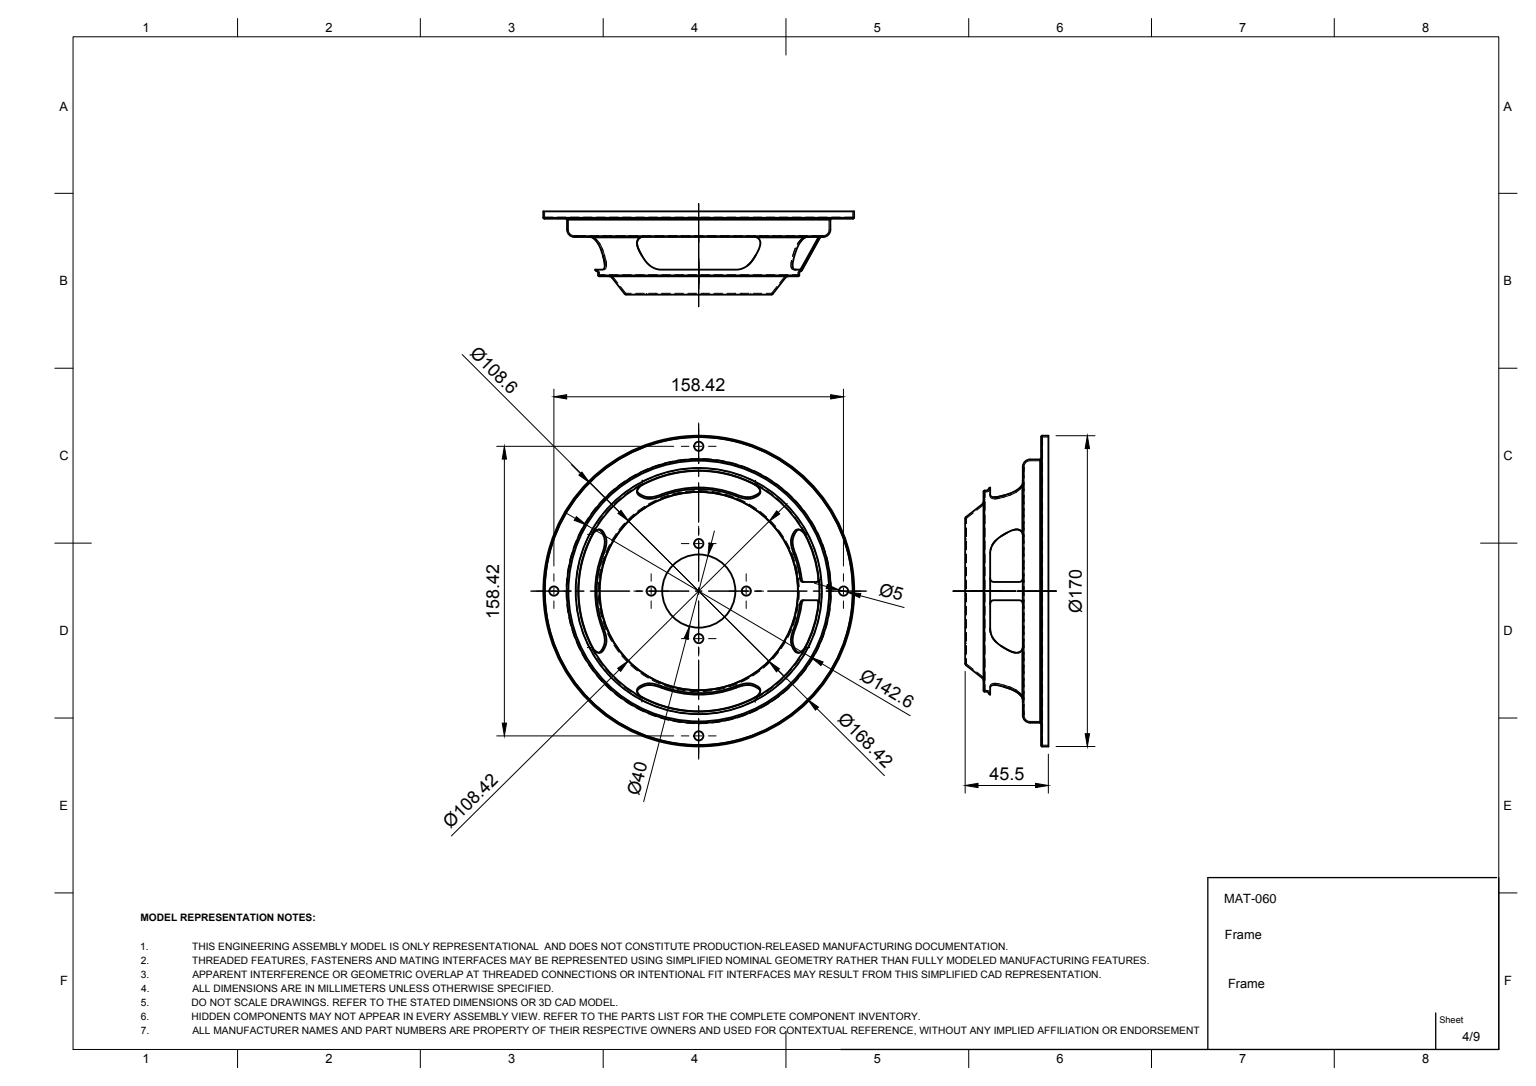
ISO-10303-21;
HEADER;
FILE_DESCRIPTION (('STEP AP214'),
    '1' );
FILE_NAME ('Frame.step',
    '2026-10-29T23:46:56',
    ( '' ),
    ( '' ),
    'SwSTEP 2.0',
    'SolidWorks 2020',
    '' );
FILE_SCHEMA (( 'AUTOMOTIVE_DESIGN' ));
ENDSEC;

DATA;
#1=ADVANCED_FACE ( 'NONE', ( #23407 ), #603, .F. ) ;
#9=CARTESIAN_POINT ( 'NONE',  ( 52.18344119656808289, -5.936379232154279428, 107.4303245894588628 ) ) ;
#10=ORIENTED_EDGE ( 'NONE', *, *, #17862, .T. ) ;
#11=DIRECTION ( 'NONE',  ( 0.000000000000000000, 0.000000000000000000, -1.000000000000000000 ) ) ;
#13=VECTOR ( 'NONE', #9862, 1000.000000000000000 ) ;
#23=DIRECTION ( 'NONE',  ( 0.000000000000000000, 0.000000000000000000, 1.000000000000000000 ) ) ;
#25=CONICAL_SURFACE ( 'NONE', #4214, 67.38776620500242132, 0.5061454830783623793 ) ;
#26=VERTEX_POINT ( 'NONE', #18783 ) ;
#40=CARTESIAN_POINT ( 'NONE',  ( 21.09785597605719332, 12.26495659406217342, 47.04930799450051637 ) ) ;
#48=DIRECTION ( 'NONE',  ( 1.000000000000000000, -3.756723415560144304E-15, 0.000000000000000000 ) ) ;
#62=PLANE ( 'NONE',  #14629 ) ;
#83=CONICAL_SURFACE ( 'NONE', #4821, 67.99999999999998579, 0.5061454830783623793 ) ;
#96=CARTESIAN_POINT ( 'NONE',  ( -35.64882101543633297, 9.925589859889722533, 42.04930799450051637 ) ) ;
#99=EDGE_LOOP ( 'NONE', ( #29307, #17559, #4595, #27909 ) ) ;
#106=DIRECTION ( 'NONE',  ( 0.000000000000000000, 0.000000000000000000, 1.000000000000000000 ) ) ;
#114=CARTESIAN_POINT ( 'NONE',  ( 80.65492537559437380, -5.936611295272316902, 15.94352045161622655 ) ) ;
#138=CIRCLE ( 'NONE', #18459, 2.500000000000003553 ) ;
#147=ORIENTED_EDGE ( 'NONE', *, *, #1574, .F. ) ;
#151=CARTESIAN_POINT ( 'NONE',  ( -9.910881874767294875, -5.936607700120025477, -13.36061728824001804 ) ) ;
#162=PRODUCT_CONTEXT ( 'NONE', #1750, 'mechanical' ) ;
#167=DIRECTION ( 'NONE',  ( -0.000000000000000000, -1.000000000000000000, -0.000000000000000000 ) ) ;
#186=EDGE_CURVE ( 'NONE', #20059, #17152, #210, .T. ) ;
#189=CARTESIAN_POINT ( 'NONE',  ( -29.27613032885505007, 5.786704587343633577, 77.24891569812123748 ) ) ;
#199=CARTESIAN_POINT ( 'NONE',  ( 42.60793425459065986, 11.86918370369814113, 98.63420711611333047 ) ) ;
#203=ORIENTED_EDGE ( 'NONE', *, *, #32319, .T. ) ;
#206=LINE ( 'NONE', #27459, #13028 ) ;
#208=ORIENTED_EDGE ( 'NONE', *, *, #19172, .F. ) ;
#210=CIRCLE ( 'NONE', #18531, 55.85791022362053582 ) ;
#235=CARTESIAN_POINT ( 'NONE',  ( -3.126678918709510313, 11.18855628041951711, -3.738293121569808086 ) ) ;
#239=CARTESIAN_POINT ( 'NONE',  ( 75.35669764717297880, -2.578969365796030200, 80.79736519221168578 ) ) ;
#245=CARTESIAN_POINT ( 'NONE',  ( 75.84373340226019877, -1.823725651226874023, 80.73552270632580985 ) ) ;
#251=DIRECTION ( 'NONE',  ( -0.000000000000000000, 1.000000000000000000, -0.000000000000000000 ) ) ;
#253=VERTEX_POINT ( 'NONE', #29471 ) ;
#259=CIRCLE ( 'NONE', #4453, 2.500000000000002220 ) ;
#274=ORIENTED_EDGE ( 'NONE', *, *, #5995, .T. ) ;
#276=CARTESIAN_POINT ( 'NONE',  ( -5.602943079677954685, 9.702389020015065313, -3.412202488244239884 ) ) ;
#279=CARTESIAN_POINT ( 'NONE',  ( -35.36141981399792655, 11.69881320456492979, 53.11437157513250895 ) ) ;
#288=AXIS2_PLACEMENT_3D ( 'NONE', #28339, #16328, #21250 ) ;
#300=EDGE_CURVE ( 'NONE', #14294, #4546, #9551, .T. ) ;
#302=ORIENTED_EDGE ( 'NONE', *, *, #7357, .T. ) ;
#308=CARTESIAN_POINT ( 'NONE',  ( -10.01358589504979513, -5.935454207834595763, -13.41617548937563598 ) ) ;
#310=ORIENTED_EDGE ( 'NONE', *, *, #2952, .T. ) ;
#313=VERTEX_POINT ( 'NONE', #14149 ) ;
#316=CARTESIAN_POINT ( 'NONE',  ( 54.19940832515395357, -4.668720686625173144, 103.9826627183073668 ) ) ;
#322=LINE ( 'NONE', #29718, #31776 ) ;
#324=CARTESIAN_POINT ( 'NONE',  ( -9.765095477396084078, -5.936631694656546721, 107.5327929641237290 ) ) ;
#336=ORIENTED_EDGE ( 'NONE', *, *, #3292, .T. ) ;
#337=EDGE_CURVE ( 'NONE', #10189, #17291, #29573, .T. ) ;
#343=CARTESIAN_POINT ( 'NONE',  ( 81.50778125879762115, -5.936607700120028142, 16.04057014367610989 ) ) ;
#355=ORIENTED_EDGE ( 'NONE', *, *, #11811, .F. ) ;
#359=CARTESIAN_POINT ( 'NONE',  ( -33.78823724555357444, -3.447124724799344175, 13.40102877645825075 ) ) ;
#370=EDGE_CURVE ( 'NONE', #26491, #3553, #7732, .T. ) ;
#378=DIRECTION ( 'NONE',  ( 1.313185983435984691E-29, -1.000000000000000000, -3.761114140369702165E-15 ) ) ;
#379=EDGE_LOOP ( 'NONE', ( #18763, #24620, #4258, #2283 ) ) ;
#388=CARTESIAN_POINT ( 'NONE',  ( 0.6836613156275053171, 11.92558985988973497, 99.90211174246701376 ) ) ;
#408=CARTESIAN_POINT ( 'NONE',  ( -38.57628410747783221, -4.281489722201563985, 13.63563177263803894 ) ) ;
#418=AXIS2_PLACEMENT_3D ( 'NONE', #18138, #28164, #5678 ) ;
#421=CARTESIAN_POINT ( 'NONE',  ( 49.52052953415556402, 8.310461108307681144, -3.337848843846767721 ) ) ;
#422=CARTESIAN_POINT ( 'NONE',  ( -9.880272688099118739, -5.935454078358227470, 107.6100695915628478 ) ) ;
#426=CARTESIAN_POINT ( 'NONE',  ( -14.15471437217249218, -3.295808585244886402, 97.43646483284780402 ) ) ;
#428=CARTESIAN_POINT ( 'NONE',  ( -34.67891837790644871, -3.387818899234932513, 80.71006381137655694 ) ) ;
#432=CARTESIAN_POINT ( 'NONE',  ( -11.20938414847590003, 2.044662169668923113, 99.18612600487385578 ) ) ;
#439=CARTESIAN_POINT ( 'NONE',  ( 21.09785597605719332, -5.986312001188950127, 47.04930799450051637 ) ) ;
#440=CARTESIAN_POINT ( 'NONE',  ( 21.09785597605719332, -19.93545420775220123, 47.04930799450051637 ) ) ;
#448=AXIS2_PLACEMENT_3D ( 'NONE', #832, #23322, #20846 ) ;
#453=ORIENTED_EDGE ( 'NONE', *, *, #7859, .T. ) ;
#458=AXIS2_PLACEMENT_3D ( 'NONE', #16097, #21670, #13655 ) ;
#461=DIRECTION ( 'NONE',  ( -0.000000000000000000, -1.000000000000000000, -0.000000000000000000 ) ) ;
#462=AXIS2_PLACEMENT_3D ( 'NONE', #31638, #14558, #26541 ) ;
#468=CARTESIAN_POINT ( 'NONE',  ( 52.49730020886497783, -5.900224301042255703, 106.3086101802585404 ) ) ;
#476=CARTESIAN_POINT ( 'NONE',  ( 54.28735269144078757, -4.535950511381776629, 103.8461761130624694 ) ) ;
#487=CARTESIAN_POINT ( 'NONE',  ( 21.09785597605719332, 24.86454579224779948, 73.04930799450052348 ) ) ;
#489=CARTESIAN_POINT ( 'NONE',  ( -31.01957187155556639, 11.71410389684668552, 24.52077559777409732 ) ) ;
#494=VECTOR ( 'NONE', #29690, 1000.000000000000000 ) ;
#499=FACE_OUTER_BOUND ( 'NONE', #20854, .T. ) ;
#501=CARTESIAN_POINT ( 'NONE',  ( -29.27613032885505007, -3.086612947480494196, 80.82450247980625591 ) ) ;
#509=DIRECTION ( 'NONE',  ( 0.000000000000000000, 0.000000000000000000, -1.000000000000000000 ) ) ;
#510=DIRECTION ( 'NONE',  ( 0.000000000000000000, 0.000000000000000000, 1.000000000000000000 ) ) ;
#516=LINE ( 'NONE', #23004, #15630 ) ;
#530=CARTESIAN_POINT ( 'NONE',  ( 21.09785597605719332, 15.56454579224779877, 47.04930799450051637 ) ) ;
#532=CIRCLE ( 'NONE', #18851, 65.75844861871132707 ) ;
#536=CARTESIAN_POINT ( 'NONE',  ( -39.42404159773660410, -5.935581334357459937, 77.97933121608268436 ) ) ;
#539=DIRECTION ( 'NONE',  ( 0.000000000000000000, 9.185193130005556732E-17, 1.000000000000000000 ) ) ;
#541=CIRCLE ( 'NONE', #29390, 39.69941114636694124 ) ;
#546=CARTESIAN_POINT ( 'NONE',  ( 21.09785597605719332, 25.56454579224779877, 73.04930799450052348 ) ) ;
#553=DIRECTION ( 'NONE',  ( 0.000000000000000000, 0.000000000000000000, -1.000000000000000000 ) ) ;
#558=ORIENTED_EDGE ( 'NONE', *, *, #25899, .F. ) ;
#559=CARTESIAN_POINT ( 'NONE',  ( 73.65314367107050941, 0.8961463385898641443, 79.88877559804848261 ) ) ;
#565=ORIENTED_EDGE ( 'NONE', *, *, #7783, .F. ) ;
#567=DIRECTION ( 'NONE',  ( 0.000000000000000000, 0.000000000000000000, 1.000000000000000000 ) ) ;
#588=FACE_OUTER_BOUND ( 'NONE', #2822, .T. ) ;
#592=CARTESIAN_POINT ( 'NONE',  ( -34.60289125444462854, 11.64119122789693961, 41.11328754109207040 ) ) ;
#595=CARTESIAN_POINT ( 'NONE',  ( -14.15471437217249218, -3.295808585244886402, 106.8025418868326284 ) ) ;
#598=CARTESIAN_POINT ( 'NONE',  ( -32.75748891819321074, -0.01103702217111705332, 80.26537595473334363 ) ) ;
#603=CYLINDRICAL_SURFACE ( 'NONE', #6358, 2.500000000000002220 ) ;
#610=FACE_OUTER_BOUND ( 'NONE', #4229, .T. ) ;
#619=ORIENTED_EDGE ( 'NONE', *, *, #25170, .T. ) ;
#621=CARTESIAN_POINT ( 'NONE',  ( -9.326276492376491589, 5.308358430270105899, 99.14268250727589304 ) ) ;
#631=VERTEX_POINT ( 'NONE', #4872 ) ;
#632=EDGE_CURVE ( 'NONE', #253, #29537, #8270, .T. ) ;
#644=CARTESIAN_POINT ( 'NONE',  ( 51.92833871100798149, 4.638969541771024829, 99.33413526210576094 ) ) ;
#649=VERTEX_POINT ( 'NONE', #13679 ) ;
#669=ADVANCED_FACE ( 'NONE', ( #28451, #21524, #18734, #1349, #11366, #13363 ), #3978, .T. ) ;
#674=CARTESIAN_POINT ( 'NONE',  ( 81.53764425905508517, -5.935454354499444918, 15.93786951028389254 ) ) ;
#677=FACE_OUTER_BOUND ( 'NONE', #17845, .T. ) ;
#681=CYLINDRICAL_SURFACE ( 'NONE', #3691, 19.99999999999999645 ) ;
#690=CARTESIAN_POINT ( 'NONE',  ( 51.67081420511490819, 5.053071141216423534, 98.28906612357258155 ) ) ;
#700=CARTESIAN_POINT ( 'NONE',  ( -39.43735134593180902, -5.935500344420906238, 77.98272432681935129 ) ) ;
#715=DIRECTION ( 'NONE',  ( 0.000000000000000000, 0.000000000000000000, -1.000000000000000000 ) ) ;
#716=DIRECTION ( 'NONE',  ( 0.000000000000000000, -1.000000000000000000, 0.000000000000000000 ) ) ;
#719=ORIENTED_EDGE ( 'NONE', *, *, #22379, .T. ) ;
#721=DIRECTION ( 'NONE',  ( 3.761114140369701376E-15, 1.000000000000000000, 0.000000000000000000 ) ) ;
#727=CARTESIAN_POINT ( 'NONE',  ( 21.09785597605720042, -5.935454207752337119, 114.2361189024295527 ) ) ;
#737=FACE_OUTER_BOUND ( 'NONE', #17782, .T. ) ;
#739=CARTESIAN_POINT ( 'NONE',  ( 50.61496291931489111, 6.662067023026866153, -4.700640528948444086 ) ) ;
#746=AXIS2_PLACEMENT_3D ( 'NONE', #5481, #25814, #3329 ) ;
#755=CARTESIAN_POINT ( 'NONE',  ( -35.36966210123092225, 10.42011316249520370, 42.00355930600723298 ) ) ;
#760=CARTESIAN_POINT ( 'NONE',  ( -30.89539544812951277, 5.684769981030545871, 77.22998724337006138 ) ) ;
#779=ORIENTED_EDGE ( 'NONE', *, *, #30659, .T. ) ;
#780=CARTESIAN_POINT ( 'NONE',  ( -12.63151429458831743, -2.181906231262896068, 102.0018054233023577 ) ) ;
#782=EDGE_CURVE ( 'NONE', #6039, #26, #8963, .T. ) ;
#787=ORIENTED_EDGE ( 'NONE', *, *, #4701, .T. ) ;
#794=CARTESIAN_POINT ( 'NONE',  ( 52.07598125554711999, -5.935454207752202116, 106.6682925056943958 ) ) ;
#803=CARTESIAN_POINT ( 'NONE',  ( 41.78490141557333004, 11.92558985988973497, 99.79672416560200077 ) ) ;
#820=EDGE_CURVE ( 'NONE', #7388, #14290, #12583, .T. ) ;
#821=ORIENTED_EDGE ( 'NONE', *, *, #29239, .F. ) ;
#822=AXIS2_PLACEMENT_3D ( 'NONE', #1912, #19630, #21767 ) ;
#825=ORIENTED_EDGE ( 'NONE', *, *, #300, .F. ) ;
#828=CARTESIAN_POINT ( 'NONE',  ( -44.53739698818294102, -4.628387878568079650, 52.16470011384033967 ) ) ;
#832=CARTESIAN_POINT ( 'NONE',  ( 47.09785597605719687, 25.56454579224779877, 47.04930799450042400 ) ) ;
#836=DIRECTION ( 'NONE',  ( 0.000000000000000000, 0.000000000000000000, -1.000000000000000000 ) ) ;
#837=CARTESIAN_POINT ( 'NONE',  ( -38.10732830366966084, -5.882756053366322568, 78.42076464377196032 ) ) ;
#840=DIRECTION ( 'NONE',  ( -0.000000000000000000, 1.000000000000000000, -0.000000000000000000 ) ) ;
#845=ORIENTED_EDGE ( 'NONE', *, *, #14632, .T. ) ;
#849=CARTESIAN_POINT ( 'NONE',  ( 50.74134730670688498, 6.496515553941725862, 97.90908627297329758 ) ) ;
#857=ADVANCED_FACE ( 'NONE', ( #10211 ), #16281, .F. ) ;
#859=CARTESIAN_POINT ( 'NONE',  ( -39.50719276739945229, -5.935457263800389960, 77.87558390080170057 ) ) ;
#870=ORIENTED_EDGE ( 'NONE', *, *, #17750, .F. ) ;
#872=CARTESIAN_POINT ( 'NONE',  ( 47.79865503179234310, 9.702389020015065313, 97.51081847724526597 ) ) ;
#874=CARTESIAN_POINT ( 'NONE',  ( -5.602943079677954685, 9.702389020015065313, 98.41455612196619995 ) ) ;
#880=CARTESIAN_POINT ( 'NONE',  ( 76.87534014094269708, -3.386628651589064898, 80.70757180512225659 ) ) ;
#892=ADVANCED_FACE ( 'NONE', ( #20693 ), #17421, .F. ) ;
#902=CARTESIAN_POINT ( 'NONE',  ( -36.15844848744088580, -5.643691937041874773, 79.05968474335206508 ) ) ;
#916=EDGE_LOOP ( 'NONE', ( #23883, #16207, #15273, #30027 ) ) ;
#919=ORIENTED_EDGE ( 'NONE', *, *, #1291, .F. ) ;
#923=CARTESIAN_POINT ( 'NONE',  ( 21.09785597605719332, -5.935454207752083988, -18.70914062421081425 ) ) ;
#935=CARTESIAN_POINT ( 'NONE',  ( -12.30971848159242121, -4.161241697801305151, 103.4774498197331667 ) ) ;
#946=LINE ( 'NONE', #24559, #9376 ) ;
#957=EDGE_LOOP ( 'NONE', ( #2500, #18429, #8067, #18740 ) ) ;
#960=CARTESIAN_POINT ( 'NONE',  ( 47.79865503179234310, 9.702389020015065313, 98.41455612196619995 ) ) ;
#966=EDGE_LOOP ( 'NONE', ( #8106, #14529, #18674, #26585 ) ) ;
#981=EDGE_LOOP ( 'NONE', ( #5763, #6597, #9287, #17362, #5522 ) ) ;
#999=CARTESIAN_POINT ( 'NONE',  ( 21.09785597605719332, 12.39166260509097484, 47.04930799450051637 ) ) ;
#1007=CARTESIAN_POINT ( 'NONE',  ( -58.11219453028166981, -15.93545420775219945, 49.54930799450023926 ) ) ;
#1009=CARTESIAN_POINT ( 'NONE',  ( -10.63512168728995100, -5.773219817368564044, 105.6277383086626145 ) ) ;
#1018=DIRECTION ( 'NONE',  ( 1.000000000000000000, -3.761114140369701376E-15, 0.000000000000000000 ) ) ;
#1028=DIRECTION ( 'NONE',  ( -0.000000000000000000, 1.000000000000000000, -0.000000000000000000 ) ) ;
#1029=DIRECTION ( 'NONE',  ( 0.000000000000000000, -1.000000000000000000, -1.251509963831984395E-16 ) ) ;
#1038=CARTESIAN_POINT ( 'NONE',  ( -63.90214402394282445, -3.935454207752203892, 40.04930799450051637 ) ) ;
#1050=CARTESIAN_POINT ( 'NONE',  ( 21.09785597605719332, -16.72540370141334520, 131.3493079945005491 ) ) ;
#1056=LINE ( 'NONE', #3025, #19895 ) ;
#1057=FACE_OUTER_BOUND ( 'NONE', #25387, .T. ) ;
#1065=VECTOR ( 'NONE', #30419, 1000.000000000000000 ) ;
#1081=PLANE ( 'NONE',  #5494 ) ;
#1096=DIRECTION ( 'NONE',  ( 0.000000000000000000, -1.000000000000000000, 0.000000000000000000 ) ) ;
#1099=AXIS2_PLACEMENT_3D ( 'NONE', #10139, #25067, #9972 ) ;
#1105=AXIS2_PLACEMENT_3D ( 'NONE', #19154, #12280, #17014 ) ;
#1115=ADVANCED_FACE ( 'NONE', ( #11018 ), #18219, .F. ) ;
#1124=DIRECTION ( 'NONE',  ( 1.177206059073964094E-16, -0.2756373558165849391, 0.9612616959384376880 ) ) ;
#1135=CIRCLE ( 'NONE', #4276, 56.47014401861810029 ) ;
#1141=CARTESIAN_POINT ( 'NONE',  ( -4.902144023942810236, 25.56454579224779877, 47.04930799450078638 ) ) ;
#1147=CARTESIAN_POINT ( 'NONE',  ( -36.31353488181962064, 10.17485700342523458, 42.04930799450051637 ) ) ;
#1152=VERTEX_POINT ( 'NONE', #19517 ) ;
#1175=ADVANCED_FACE ( 'NONE', ( #19187 ), #14452, .F. ) ;
#1176=ORIENTED_EDGE ( 'NONE', *, *, #19284, .F. ) ;
#1178=DIRECTION ( 'NONE',  ( 1.000000000000000000, -0.000000000000000000, -0.000000000000000000 ) ) ;
#1194=DIRECTION ( 'NONE',  ( 0.000000000000000000, 1.000000000000000000, 0.000000000000000000 ) ) ;
#1198=ORIENTED_EDGE ( 'NONE', *, *, #25045, .T. ) ;
#1208=CARTESIAN_POINT ( 'NONE',  ( 53.51600554467332671, -5.395280703882722406, -10.73892745771225599 ) ) ;
#1210=ORIENTED_EDGE ( 'NONE', *, *, #8305, .T. ) ;
#1215=VERTEX_POINT ( 'NONE', #17056 ) ;
#1220=CARTESIAN_POINT ( 'NONE',  ( -33.86637752982123573, -3.544489376609568421, 80.67335282074090230 ) ) ;
#1223=CARTESIAN_POINT ( 'NONE',  ( -34.46767470602752326, 11.80860034638430989, 40.73713547295701431 ) ) ;
#1224=VERTEX_POINT ( 'NONE', #15093 ) ;
#1230=CARTESIAN_POINT ( 'NONE',  ( 21.09785597605719332, -15.93545420775219945, 47.04930799450051637 ) ) ;
#1248=CARTESIAN_POINT ( 'NONE',  ( -10.01616728275229740, -5.935340315990530691, -13.32263710021335612 ) ) ;
#1273=CARTESIAN_POINT ( 'NONE',  ( 0.6836613156275053171, 11.92558985988973497, -5.803495753465989893 ) ) ;
#1285=FACE_OUTER_BOUND ( 'NONE', #3726, .T. ) ;
#1290=LINE ( 'NONE', #23943, #31888 ) ;
#1291=EDGE_CURVE ( 'NONE', #10579, #24958, #20556, .T. ) ;
#1299=EDGE_LOOP ( 'NONE', ( #8915, #25452, #7300, #565, #2321, #17317 ) ) ;
#1305=AXIS2_PLACEMENT_3D ( 'NONE', #9730, #19722, #27116 ) ;
#1309=CARTESIAN_POINT ( 'NONE',  ( -35.14417515838577089, 11.92558985988973674, 40.19270369045111124 ) ) ;
#1340=VERTEX_POINT ( 'NONE', #27894 ) ;
#1341=DIRECTION ( 'NONE',  ( -1.000000000000000000, 0.000000000000000000, 0.000000000000000000 ) ) ;
#1349=FACE_BOUND ( 'NONE', #4250, .T. ) ;
#1354=DIRECTION ( 'NONE',  ( 0.000000000000000000, 0.000000000000000000, 1.000000000000000000 ) ) ;
#1366=DIRECTION ( 'NONE',  ( -1.000000000000000000, -0.000000000000000000, -3.491481338843133355E-15 ) ) ;
#1367=CARTESIAN_POINT ( 'NONE',  ( 21.09785597605719332, -19.93545420775220123, 47.04930799450051637 ) ) ;
#1370=DIRECTION ( 'NONE',  ( -0.000000000000000000, -0.000000000000000000, -1.000000000000000000 ) ) ;
#1372=CARTESIAN_POINT ( 'NONE',  ( 51.66808379569695830, 5.388785998227650254, 106.7232700815558957 ) ) ;
#1430=ORIENTED_EDGE ( 'NONE', *, *, #12094, .F. ) ;
#1431=CARTESIAN_POINT ( 'NONE',  ( -10.77327584252841675, 2.854128177266956445, -4.829733788720330878 ) ) ;
#1464=MANIFOLD_SOLID_BREP ( 'Stock-MAT-060-1', #18928 ) ;
#1469=CARTESIAN_POINT ( 'NONE',  ( 76.12931116418575073, -2.304636120132655286, 13.31869760836049466 ) ) ;
#1509=ADVANCED_FACE ( 'NONE', ( #13448 ), #18665, .F. ) ;
#1524=CARTESIAN_POINT ( 'NONE',  ( -39.54681582271551576, -5.935578394679064118, 77.88069024016000697 ) ) ;
#1527=CARTESIAN_POINT ( 'NONE',  ( -44.16105795751995799, -3.935454207752190126, 42.04930799450051637 ) ) ;
#1535=AXIS2_PLACEMENT_3D ( 'NONE', #14725, #29989, #106 ) ;
#1552=DIRECTION ( 'NONE',  ( -0.000000000000000000, 1.000000000000000000, -0.000000000000000000 ) ) ;
#1562=DIRECTION ( 'NONE',  ( 0.000000000000000000, 0.000000000000000000, -1.000000000000000000 ) ) ;
#1563=CARTESIAN_POINT ( 'NONE',  ( -35.12632216515690686, 11.92558985988973674, 40.04930799450050216 ) ) ;
#1572=ORIENTED_EDGE ( 'NONE', *, *, #13901, .T. ) ;
#1574=EDGE_CURVE ( 'NONE', #5070, #14564, #7015, .T. ) ;
#1578=EDGE_CURVE ( 'NONE', #29191, #20681, #12935, .T. ) ;
#1592=AXIS2_PLACEMENT_3D ( 'NONE', #8643, #21258, #11114 ) ;
#1600=DIRECTION ( 'NONE',  ( 0.000000000000000000, 0.000000000000000000, 1.000000000000000000 ) ) ;
#1603=FACE_OUTER_BOUND ( 'NONE', #20703, .T. ) ;
#1620=FACE_OUTER_BOUND ( 'NONE', #14364, .T. ) ;
#1623=VECTOR ( 'NONE', #1124, 1000.000000000000000 ) ;
#1629=CARTESIAN_POINT ( 'NONE',  ( 21.09785597605719332, 15.63322284159649556, -0.008722863421593840538 ) ) ;
#1632=AXIS2_PLACEMENT_3D ( 'NONE', #17122, #14681, #14197 ) ;
#1636=CARTESIAN_POINT ( 'NONE',  ( 75.71263776093286424, -1.580002914024330574, 13.40786461638758098 ) ) ;
#1652=FACE_BOUND ( 'NONE', #19233, .T. ) ;
#1654=CARTESIAN_POINT ( 'NONE',  ( -9.316012264051970249, 5.323792735596123649, -5.040144599709082129 ) ) ;
#1661=CARTESIAN_POINT ( 'NONE',  ( 21.09785597605719332, -19.93545420775220123, 67.04930799450050927 ) ) ;
#1675=CARTESIAN_POINT ( 'NONE',  ( 54.84591317376816022, -2.578969365796082158, -7.209533676615418329 ) ) ;
#1689=ORIENTED_EDGE ( 'NONE', *, *, #14950, .F. ) ;
#1699=DIRECTION ( 'NONE',  ( -1.000000000000000000, 0.000000000000000000, 2.775557561562888984E-15 ) ) ;
#1701=CARTESIAN_POINT ( 'NONE',  ( 72.51299575579318457, 10.39233698702945929, 21.28292367868997204 ) ) ;
#1708=EDGE_CURVE ( 'NONE', #32242, #3463, #29778, .T. ) ;
#1713=VECTOR ( 'NONE', #6688, 1000.000000000000000 ) ;
#1716=CARTESIAN_POINT ( 'NONE',  ( -29.68171735516254373, 11.15114065686176303, 71.33410141647549096 ) ) ;
#1717=CARTESIAN_POINT ( 'NONE',  ( 81.75997733922811506, -5.936629510748242744, 77.99024554604916659 ) ) ;
#1737=CARTESIAN_POINT ( 'NONE',  ( -44.28695544631908376, -5.935454207752205669, 40.04930799450050216 ) ) ;
#1744=ORIENTED_EDGE ( 'NONE', *, *, #22791, .F. ) ;
#1750=APPLICATION_CONTEXT ( 'automotive_design' ) ;
#1755=VECTOR ( 'NONE', #11846, 1000.000000000000000 ) ;
#1763=CARTESIAN_POINT ( 'NONE',  ( -12.56410411622038303, -3.374355247260697244, -7.781004297996404695 ) ) ;
#1791=ADVANCED_FACE ( 'NONE', ( #17996 ), #8000, .F. ) ;
#1794=CARTESIAN_POINT ( 'NONE',  ( 21.09785597605719332, 15.06454579224778456, 102.0493079945005093 ) ) ;
#1800=CARTESIAN_POINT ( 'NONE',  ( 78.44397203118849404, -5.043292969097946887, 14.24782339319855318 ) ) ;
#1808=CARTESIAN_POINT ( 'NONE',  ( 21.09785597605719332, -15.93545420775219945, 126.2593585008393831 ) ) ;
#1809=CARTESIAN_POINT ( 'NONE',  ( -45.58211410561983001, -5.881662548112003286, 40.51623134221831890 ) ) ;
#1818=ORIENTED_EDGE ( 'NONE', *, *, #5124, .F. ) ;
#1819=CARTESIAN_POINT ( 'NONE',  ( -11.94109704398765537, 0.4256545730735167288, -6.630874157835914495 ) ) ;
#1822=DIRECTION ( 'NONE',  ( 0.000000000000000000, 0.000000000000000000, -1.000000000000000000 ) ) ;
#1827=AXIS2_PLACEMENT_3D ( 'NONE', #13329, #10539, #25781 ) ;
#1841=CARTESIAN_POINT ( 'NONE',  ( 21.09785597605720397, -15.43545420775221366, -24.95069200549946586 ) ) ;
#1857=CARTESIAN_POINT ( 'NONE',  ( -39.56017130034231144, -5.935730392421668888, 77.88797225724067630 ) ) ;
#1859=CARTESIAN_POINT ( 'NONE',  ( 80.71684048725118998, -5.935454207752202116, 16.07118271501079221 ) ) ;
#1864=CARTESIAN_POINT ( 'NONE',  ( 21.09785597605719332, 25.56454579224779877, 70.54930799450050927 ) ) ;
#1869=ORIENTED_EDGE ( 'NONE', *, *, #28980, .T. ) ;
#1873=ORIENTED_EDGE ( 'NONE', *, *, #18457, .T. ) ;
#1878=VERTEX_POINT ( 'NONE', #8638 ) ;
#1893=ADVANCED_FACE ( 'NONE', ( #9279 ), #83, .T. ) ;
#1894=VERTEX_POINT ( 'NONE', #21900 ) ;
#1907=AXIS2_PLACEMENT_3D ( 'NONE', #28226, #27904, #5419 ) ;
#1912=CARTESIAN_POINT ( 'NONE',  ( 21.09785597605719332, 25.56454579224779877, 47.04930799450051637 ) ) ;
#1918=CARTESIAN_POINT ( 'NONE',  ( -11.49897738644833645, -5.264348929021194223, -9.633576251181647621 ) ) ;
#1920=CARTESIAN_POINT ( 'NONE',  ( 81.79971628361815306, -5.937448199248381187, 77.92687966219790496 ) ) ;
#1922=AXIS2_PLACEMENT_3D ( 'NONE', #20265, #2460, #29877 ) ;
#1924=CARTESIAN_POINT ( 'NONE',  ( 21.09785597605719332, -8.535454207752287914, 47.04930799450051637 ) ) ;
#1931=CARTESIAN_POINT ( 'NONE',  ( 21.09785597605719332, -5.935454207752083988, 47.04930799449963530 ) ) ;
#1934=CARTESIAN_POINT ( 'NONE',  ( 41.51205063648687599, 11.92558985988973497, -37.95069200549950494 ) ) ;
#1938=CARTESIAN_POINT ( 'NONE',  ( -29.27337757263006424, 2.267350949466874432, 14.79705809024468088 ) ) ;
#1946=EDGE_LOOP ( 'NONE', ( #12322, #14844, #6465, #22478 ) ) ;
#1957=CARTESIAN_POINT ( 'NONE',  ( 75.25323102592015800, -0.6709275202869922072, 13.62290469009603022 ) ) ;
#1976=CARTESIAN_POINT ( 'NONE',  ( -6.242780362964605700, 9.162376348828958683, -4.318210402824582239 ) ) ;
#1986=ORIENTED_EDGE ( 'NONE', *, *, #27426, .F. ) ;
#1991=EDGE_CURVE ( 'NONE', #17686, #12130, #16391, .T. ) ;
#1999=CARTESIAN_POINT ( 'NONE',  ( 53.71827270862435455, -5.211355130743560160, -9.585364147679955593 ) ) ;
#2013=VECTOR ( 'NONE', #10033, 1000.000000000000000 ) ;
#2014=CARTESIAN_POINT ( 'NONE',  ( 52.81327818505165794, -5.811083640285383822, 104.5757368101217679 ) ) ;
#2015=ORIENTED_EDGE ( 'NONE', *, *, #27426, .T. ) ;
#2028=CARTESIAN_POINT ( 'NONE',  ( 72.31638179958355295, 11.69718155787697356, 24.43823011782819776 ) ) ;
#2039=CARTESIAN_POINT ( 'NONE',  ( -30.66701073789274901, 11.92468888572869723, 68.04721722412880069 ) ) ;
#2040=CARTESIAN_POINT ( 'NONE',  ( -29.27613032885505007, -5.935454207752198563, 77.87546120947918382 ) ) ;
#2043=CARTESIAN_POINT ( 'NONE',  ( 51.92400919103563695, -5.935454207752202116, -13.39445452378610568 ) ) ;
#2046=DIRECTION ( 'NONE',  ( -0.000000000000000000, -1.000000000000000000, -0.000000000000000000 ) ) ;
#2047=CARTESIAN_POINT ( 'NONE',  ( 71.61810346057937693, 10.40257568944042710, 72.79952121014760280 ) ) ;
#2073=CARTESIAN_POINT ( 'NONE',  ( 21.09785597605719332, 16.86454579224779948, 47.04930799450051637 ) ) ;
#2083=CARTESIAN_POINT ( 'NONE',  ( 21.09785597605719332, -6.314304012688826795, -18.91914050022838012 ) ) ;
#2085=CARTESIAN_POINT ( 'NONE',  ( -12.50119137592388441, -1.331120222581884560, -6.486951009445048655 ) ) ;
#2086=VERTEX_POINT ( 'NONE', #727 ) ;
#2104=CARTESIAN_POINT ( 'NONE',  ( -29.27337757263006424, 11.92558985988973497, 26.63511333407100778 ) ) ;
#2105=ORIENTED_EDGE ( 'NONE', *, *, #26289, .F. ) ;
#2109=ORIENTED_EDGE ( 'NONE', *, *, #21254, .T. ) ;
#2113=EDGE_CURVE ( 'NONE', #11449, #13013, #22617, .T. ) ;
#2127=DIRECTION ( 'NONE',  ( 0.000000000000000000, 3.754529891495955404E-16, -1.000000000000000000 ) ) ;
#2128=EDGE_LOOP ( 'NONE', ( #25205, #31539, #7322, #24885 ) ) ;
#2130=B_SPLINE_CURVE_WITH_KNOTS ( 'NONE', 3,
 ( #29565, #16909, #16580, #14301, #31697, #16739, #9209, #27088, #28917, #26765, #26929, #11503, #4284, #13979, #31855, #24302, #19200, #21499, #21673, #11838, #1819, #29396, #4445, #9370, #24627, #19533, #1654, #19366, #14467, #19039, #14623, #2147, #24461, #1976, #14138, #16425 ),
 .UNSPECIFIED., .F., .F.,
 ( 4, 2, 2, 2, 2, 2, 2, 2, 2, 2, 2, 2, 2, 2, 2, 2, 2, 4 ),
 ( 2.602085213965210642E-18, 0.001253900128824282905, 0.001880850193236422189, 0.002507800257648561473, 0.003134750322060700974, 0.003761700386472840475, 0.005015600515297116008, 0.005642550579709253340, 0.006269500644121390673, 0.007523400772945662736, 0.008777300901769934799, 0.01003120103059420773, 0.01253900128824275012, 0.01504680154589129598, 0.01630070167471556544, 0.01755460180353983837, 0.01880850193236410783, 0.02006240206118838076 ),
 .UNSPECIFIED. ) ;
#2147=CARTESIAN_POINT ( 'NONE',  ( -7.125208762201825863, 8.281585831149227417, -4.396110345893636584 ) ) ;
#2151=ORIENTED_EDGE ( 'NONE', *, *, #17153, .F. ) ;
#2152=CARTESIAN_POINT ( 'NONE',  ( 21.09785597605719332, 25.56454579224779877, 73.04930799450052348 ) ) ;
#2165=VERTEX_POINT ( 'NONE', #13372 ) ;
#2166=CIRCLE ( 'NONE', #8471, 54.49999999999997868 ) ;
#2169=CARTESIAN_POINT ( 'NONE',  ( 49.11022725746682482, 8.508769500014663478, -3.454732803723541412 ) ) ;
#2177=FACE_BOUND ( 'NONE', #7800, .T. ) ;
#2183=CARTESIAN_POINT ( 'NONE',  ( -30.20912666432285576, 4.777658832336100225, 16.29113105709203779 ) ) ;
#2187=FACE_OUTER_BOUND ( 'NONE', #30023, .T. ) ;
#2195=CARTESIAN_POINT ( 'NONE',  ( -9.880269303432738681, -5.935454207752202116, -12.62465409255485582 ) ) ;
#2196=CARTESIAN_POINT ( 'NONE',  ( -39.45773241730296377, -5.935454212835550969, 77.98461610899785512 ) ) ;
#2197=AXIS2_PLACEMENT_3D ( 'NONE', #3174, #13217, #12896 ) ;
#2201=ORIENTED_EDGE ( 'NONE', *, *, #8975, .T. ) ;
#2207=CARTESIAN_POINT ( 'NONE',  ( -30.66127778995677033, 3.242016564995574335, 78.70398512147052372 ) ) ;
#2223=DIRECTION ( 'NONE',  ( 0.000000000000000000, 0.000000000000000000, -1.000000000000000000 ) ) ;
#2240=ORIENTED_EDGE ( 'NONE', *, *, #13865, .T. ) ;
#2243=AXIS2_PLACEMENT_3D ( 'NONE', #9490, #16213, #21781 ) ;
#2251=CARTESIAN_POINT ( 'NONE',  ( -8.054007235165986600, 7.161243906346020260, 97.76730497187020319 ) ) ;
#2253=CARTESIAN_POINT ( 'NONE',  ( -30.29083761341767911, 10.19527012171080393, 20.98910367824052159 ) ) ;
#2256=CARTESIAN_POINT ( 'NONE',  ( 81.79971628361815306, -5.937394935145312580, 77.97850100859398026 ) ) ;
#2259=CARTESIAN_POINT ( 'NONE',  ( 52.07598125554711999, -5.935454207752202116, 107.5832303370038403 ) ) ;
#2268=CARTESIAN_POINT ( 'NONE',  ( 106.0978559760574313, 1.925589859889728972, 67.46350265493050813 ) ) ;
#2273=CARTESIAN_POINT ( 'NONE',  ( -29.27337757263006424, -3.086620340690746644, 13.27411520529475020 ) ) ;
#2280=AXIS2_PLACEMENT_3D ( 'NONE', #12246, #32269, #2712 ) ;
#2282=AXIS2_PLACEMENT_3D ( 'NONE', #8168, #15877, #13267 ) ;
#2283=ORIENTED_EDGE ( 'NONE', *, *, #5714, .F. ) ;
#2301=SHAPE_DEFINITION_REPRESENTATION ( #8290, #3604 ) ;
#2306=EDGE_CURVE ( 'NONE', #17291, #14793, #22637, .T. ) ;
#2313=CARTESIAN_POINT ( 'NONE',  ( 52.07598125554711999, -5.935454207752203004, 107.5573216553427187 ) ) ;
#2321=ORIENTED_EDGE ( 'NONE', *, *, #21254, .F. ) ;
#2324=CARTESIAN_POINT ( 'NONE',  ( 73.19394920542428906, 11.69997306056223607, 69.64732492378499273 ) ) ;
#2334=DIRECTION ( 'NONE',  ( -0.000000000000000000, 1.000000000000000000, -0.000000000000000000 ) ) ;
#2344=FACE_OUTER_BOUND ( 'NONE', #18141, .T. ) ;
#2370=B_SPLINE_CURVE_WITH_KNOTS ( 'NONE', 3,
 ( #26492, #9256, #1701, #11084, #6306, #13541, #14023, #16794, #16311, #21071, #11722, #18604 ),
 .UNSPECIFIED., .F., .F.,
 ( 4, 2, 2, 2, 2, 4 ),
 ( 0.0003422370341462280100, 0.002080102550335780759, 0.003817968066525333128, 0.005555833582714885498, 0.006424766340809661899, 0.007293699098904438301 ),
 .UNSPECIFIED. ) ;
#2381=ORIENTED_EDGE ( 'NONE', *, *, #26036, .T. ) ;
#2385=CARTESIAN_POINT ( 'NONE',  ( 72.66453678218256584, 3.903925281081655818, 78.31450457581732394 ) ) ;
#2388=DIRECTION ( 'NONE',  ( -0.000000000000000000, -1.000000000000000000, -0.000000000000000000 ) ) ;
#2426=CARTESIAN_POINT ( 'NONE',  ( -35.12632216515691397, 11.92558985988973674, 54.04930799450053769 ) ) ;
#2434=CARTESIAN_POINT ( 'NONE',  ( -44.16105795751995799, -3.935454207752183020, 52.04930799450050927 ) ) ;
#2435=ORIENTED_EDGE ( 'NONE', *, *, #10167, .T. ) ;
#2448=FACE_OUTER_BOUND ( 'NONE', #29487, .T. ) ;
#2449=EDGE_CURVE ( 'NONE', #28013, #10438, #11704, .T. ) ;
#2460=DIRECTION ( 'NONE',  ( -0.000000000000000000, -1.000000000000000000, -0.000000000000000000 ) ) ;
#2467=VERTEX_POINT ( 'NONE', #8521 ) ;
#2494=DIRECTION ( 'NONE',  ( 1.313185983435984691E-29, -1.000000000000000000, -3.761114140369702165E-15 ) ) ;
#2496=B_SPLINE_SURFACE_WITH_KNOTS ( 'NONE', 3, 1, ( 
 ( #29765, #9584 ),
 ( #21872, #27467 ),
 ( #9252, #19905 ),
 ( #19413, #31899 ) ),
 .UNSPECIFIED., .F., .F., .F.,
 ( 4, 4 ),
 ( 2, 2 ),
 ( 0.9958781556774846111, 1.000000000000000000 ),
 ( 0.000000000000000000, 1.000000000000000000 ),
 .UNSPECIFIED. ) ;
#2500=ORIENTED_EDGE ( 'NONE', *, *, #9156, .F. ) ;
#2508=CARTESIAN_POINT ( 'NONE',  ( 41.51205063648687599, 11.92558985988973497, -4.944603100128015960 ) ) ;
#2509=ORIENTED_EDGE ( 'NONE', *, *, #10196, .T. ) ;
#2514=DIRECTION ( 'NONE',  ( -0.000000000000000000, -1.000000000000000000, -0.000000000000000000 ) ) ;
#2519=ORIENTED_EDGE ( 'NONE', *, *, #32257, .F. ) ;
#2526=CARTESIAN_POINT ( 'NONE',  ( -9.883074696779189594, -5.935345006353231589, 107.4930705127871846 ) ) ;
#2530=ORIENTED_EDGE ( 'NONE', *, *, #20490, .F. ) ;
#2538=CARTESIAN_POINT ( 'NONE',  ( 71.64025509781936307, 8.185031362399408650, 75.36104810003064358 ) ) ;
#2541=DIRECTION ( 'NONE',  ( 0.000000000000000000, -0.2756373558169902815, -0.9612616959383214477 ) ) ;
#2543=CARTESIAN_POINT ( 'NONE',  ( 21.09785597605719332, 17.56454579224779877, 47.04930799450051637 ) ) ;
#2545=DIRECTION ( 'NONE',  ( 0.000000000000000000, 0.000000000000000000, -1.000000000000000000 ) ) ;
#2547=EDGE_LOOP ( 'NONE', ( #24954, #30069, #15985, #23180 ) ) ;
#2548=LINE ( 'NONE', #29481, #18243 ) ;
#2550=ORIENTED_EDGE ( 'NONE', *, *, #23423, .T. ) ;
#2553=EDGE_CURVE ( 'NONE', #1215, #16982, #10146, .T. ) ;
#2561=FACE_OUTER_BOUND ( 'NONE', #28539, .T. ) ;
#2563=ORIENTED_EDGE ( 'NONE', *, *, #21276, .T. ) ;
#2565=CARTESIAN_POINT ( 'NONE',  ( 73.61977373202824992, 0.9814505390143158925, 14.24566699581558638 ) ) ;
#2566=CARTESIAN_POINT ( 'NONE',  ( 42.05610609765635388, 11.92558985988972964, -5.593356398450009870 ) ) ;
#2569=CARTESIAN_POINT ( 'NONE',  ( 21.09785597605719332, 14.56957104541719694, -7.455717258668906666 ) ) ;
#2571=CARTESIAN_POINT ( 'NONE',  ( -12.59080382683723442, -1.820484904611798349, 100.8496278133052897 ) ) ;
#2579=CIRCLE ( 'NONE', #8852, 67.36417311134211161 ) ;
#2581=FACE_OUTER_BOUND ( 'NONE', #27056, .T. ) ;
#2591=EDGE_CURVE ( 'NONE', #27103, #29537, #16694, .T. ) ;
#2593=LINE ( 'NONE', #30336, #17952 ) ;
#2614=VERTEX_POINT ( 'NONE', #4241 ) ;
#2617=ORIENTED_EDGE ( 'NONE', *, *, #25045, .F. ) ;
#2619=CARTESIAN_POINT ( 'NONE',  ( 21.09785597605719332, 15.56454579224779877, -7.450692005499464088 ) ) ;
#2631=EDGE_CURVE ( 'NONE', #3463, #27012, #9072, .T. ) ;
#2635=ORIENTED_EDGE ( 'NONE', *, *, #31498, .F. ) ;
#2650=AXIS2_PLACEMENT_3D ( 'NONE', #6932, #27605, #24486 ) ;
#2662=CARTESIAN_POINT ( 'NONE',  ( 41.51205063648687599, 11.92558985988973497, 99.04321908912902472 ) ) ;
#2667=ORIENTED_EDGE ( 'NONE', *, *, #32219, .F. ) ;
#2671=DIRECTION ( 'NONE',  ( 0.000000000000000000, -1.000000000000000000, 0.000000000000000000 ) ) ;
#2672=CARTESIAN_POINT ( 'NONE',  ( 54.82737574693081939, -2.284241381456145970, 101.1271600646791029 ) ) ;
#2685=B_SPLINE_CURVE_WITH_KNOTS ( 'NONE', 3,
 ( #29665, #11936, #4547, #4713, #21932, #14733, #2251, #14563, #12271, #5374, #25228, #27525, #8157, #14894, #432, #12600, #30316, #15532, #5203, #10457, #2571, #5046, #15054, #22419, #20129, #2739, #15377, #30486, #18147, #13086, #12435, #32454, #15213, #9966, #29995, #7830 ),
 .UNSPECIFIED., .F., .F.,
 ( 4, 2, 2, 2, 2, 2, 2, 2, 2, 2, 2, 2, 2, 2, 2, 2, 2, 4 ),
 ( 0.000000000000000000, 0.001327013081135473057, 0.002654026162270946114, 0.003981039243406417003, 0.005308052324541888758, 0.006635065405677360514, 0.007962078486812830536, 0.01061610464908377231, 0.01194311773021923886, 0.01327013081135470368, 0.01459714389249017023, 0.01592415697362563679, 0.01725117005476110160, 0.01857818313589656642, 0.01924168967646430056, 0.01990519621703203124, 0.02056870275759976191, 0.02123220929816749258 ),
 .UNSPECIFIED. ) ;
#2686=ORIENTED_EDGE ( 'NONE', *, *, #28464, .F. ) ;
#2689=CARTESIAN_POINT ( 'NONE',  ( 21.09785597605719332, 14.77459629858661572, 101.3493079945005206 ) ) ;
#2703=CARTESIAN_POINT ( 'NONE',  ( 71.55760889374487022, 9.126991894476596201, 74.42996348956144459 ) ) ;
#2708=FACE_OUTER_BOUND ( 'NONE', #13436, .T. ) ;
#2709=ORIENTED_EDGE ( 'NONE', *, *, #12911, .F. ) ;
#2712=DIRECTION ( 'NONE',  ( 0.000000000000000000, 0.000000000000000000, 1.000000000000000000 ) ) ;
#2713=ORIENTED_EDGE ( 'NONE', *, *, #4530, .T. ) ;
#2715=CARTESIAN_POINT ( 'NONE',  ( 21.09785597605719332, -19.93545420775220123, 47.04930799450051637 ) ) ;
#2726=VERTEX_POINT ( 'NONE', #25241 ) ;
#2733=CARTESIAN_POINT ( 'NONE',  ( 43.69587290534151691, 11.69997306056223607, -5.046785234866655756 ) ) ;
#2734=CARTESIAN_POINT ( 'NONE',  ( -5.602943079677954685, 9.702389020015065313, 98.41455612196619995 ) ) ;
#2735=CARTESIAN_POINT ( 'NONE',  ( -30.56895382951262619, 7.047361869319173522, 76.28100816727524602 ) ) ;
#2739=CARTESIAN_POINT ( 'NONE',  ( -12.07837398813756913, -4.576799740321095378, 102.9520008778022913 ) ) ;
#2744=EDGE_LOOP ( 'NONE', ( #13844, #8496 ) ) ;
#2747=CARTESIAN_POINT ( 'NONE',  ( 81.71508932399986236, -5.936918531481694572, 15.99626209184008552 ) ) ;
#2755=CYLINDRICAL_SURFACE ( 'NONE', #17209, 2.500000000000002220 ) ;
#2783=CARTESIAN_POINT ( 'NONE',  ( 54.63702927177264002, -3.812314126620138577, 103.1735800200605553 ) ) ;
#2790=DIRECTION ( 'NONE',  ( -1.000000000000000000, 0.000000000000000000, -1.110223024625155594E-14 ) ) ;
#2800=AXIS2_PLACEMENT_3D ( 'NONE', #1931, #21944, #9653 ) ;
#2806=EDGE_CURVE ( 'NONE', #1340, #8773, #10695, .T. ) ;
#2812=CARTESIAN_POINT ( 'NONE',  ( 52.12585496443453081, -5.943281723642242831, -10.93395394839392587 ) ) ;
#2815=DIRECTION ( 'NONE',  ( 0.000000000000000000, 0.000000000000000000, -1.000000000000000000 ) ) ;
#2822=EDGE_LOOP ( 'NONE', ( #10818, #13643, #14022, #11285 ) ) ;
#2823=ORIENTED_EDGE ( 'NONE', *, *, #22749, .T. ) ;
#2825=CARTESIAN_POINT ( 'NONE',  ( -31.67509402814005881, 0.3087484226586330038, 13.94399873050154781 ) ) ;
#2826=CARTESIAN_POINT ( 'NONE',  ( 53.37090610332811025, 2.112486173643655096, 99.16308969199836554 ) ) ;
#2830=VERTEX_POINT ( 'NONE', #4894 ) ;
#2837=CIRCLE ( 'NONE', #31726, 1.700000000000000178 ) ;
#2846=EDGE_CURVE ( 'NONE', #11299, #8773, #3328, .T. ) ;
#2855=CARTESIAN_POINT ( 'NONE',  ( -0.4058007941739975033, 11.88152873911358753, 99.49782616222140064 ) ) ;
#2871=CARTESIAN_POINT ( 'NONE',  ( -10.30158825675060008, -5.900224301042254815, -12.20999419125749696 ) ) ;
#2872=CARTESIAN_POINT ( 'NONE',  ( -45.72330504332163059, -5.935454207752205669, 40.04930799450050216 ) ) ;
#2873=CARTESIAN_POINT ( 'NONE',  ( -38.57628410747783221, -5.935454207752202116, 16.07118271501078866 ) ) ;
#2880=VECTOR ( 'NONE', #12997, 1000.000000000000000 ) ;
#2882=B_SPLINE_CURVE_WITH_KNOTS ( 'NONE', 3,
 ( #12590, #422, #15365, #9514, #20119, #23068, #25534, #8147, #30150, #7818, #20275, #20441 ),
 .UNSPECIFIED., .F., .F.,
 ( 4, 2, 2, 2, 2, 4 ),
 ( 0.0003195369756189209219, 0.0003994212195236353908, 0.0004793054634283499139, 0.0005192475853807071483, 0.0005591897073330643828, 0.0006390739512378048725 ),
 .UNSPECIFIED. ) ;
#2886=CARTESIAN_POINT ( 'NONE',  ( 21.09785597605719332, -9.935454207752199451, 118.3493079945004922 ) ) ;
#2892=CARTESIAN_POINT ( 'NONE',  ( -44.02786950842664027, -5.204346380200058242, 52.49783445483662803 ) ) ;
#2898=VERTEX_POINT ( 'NONE', #8649 ) ;
#2903=CARTESIAN_POINT ( 'NONE',  ( -35.22851096958370221, 11.86391768464652152, 53.48664131055646465 ) ) ;
#2934=ORIENTED_EDGE ( 'NONE', *, *, #7599, .T. ) ;
#2937=CARTESIAN_POINT ( 'NONE',  ( 54.80744232836631369, -3.171899563477265094, 102.6569140501756152 ) ) ;
#2945=CARTESIAN_POINT ( 'NONE',  ( 21.09785597605720397, -15.93545420775219945, 131.5493079945005377 ) ) ;
#2952=EDGE_CURVE ( 'NONE', #16490, #29214, #12461, .T. ) ;
#2960=ORIENTED_EDGE ( 'NONE', *, *, #12826, .T. ) ;
#2961=CARTESIAN_POINT ( 'NONE',  ( -29.27613032885505007, 11.92558985988973497, 67.46350265493038023 ) ) ;
#2972=CARTESIAN_POINT ( 'NONE',  ( 43.70893385272968601, 11.69718155787697356, 98.26783381802677297 ) ) ;
#2979=DIRECTION ( 'NONE',  ( 0.000000000000000000, 0.000000000000000000, -1.000000000000000000 ) ) ;
#2991=CARTESIAN_POINT ( 'NONE',  ( -39.48645896158937774, -5.935494601668936276, 77.87709717717420688 ) ) ;
#2999=ORIENTED_EDGE ( 'NONE', *, *, #19749, .F. ) ;
#3010=CARTESIAN_POINT ( 'NONE',  ( 76.42527971025482714, -3.977894809549873401, 80.53958960090274388 ) ) ;
#3016=CARTESIAN_POINT ( 'NONE',  ( 76.50383461303660226, -2.878806504921911813, 80.77738562869335226 ) ) ;
#3022=EDGE_LOOP ( 'NONE', ( #4299, #29590, #26515, #5708 ) ) ;
#3025=CARTESIAN_POINT ( 'NONE',  ( 51.92400919103565116, -5.935454207752198563, -37.95069200549950494 ) ) ;
#3026=ADVANCED_FACE ( 'NONE', ( #17143 ), #18019, .F. ) ;
#3027=CARTESIAN_POINT ( 'NONE',  ( 53.25347890682692054, -5.581242224118425632, -11.00365297242568374 ) ) ;
#3030=ORIENTED_EDGE ( 'NONE', *, *, #14643, .T. ) ;
#3035=AXIS2_PLACEMENT_3D ( 'NONE', #2073, #9793, #12757 ) ;
#3043=ORIENTED_EDGE ( 'NONE', *, *, #3175, .F. ) ;
#3076=CIRCLE ( 'NONE', #462, 2.500000000000003553 ) ;
#3078=VERTEX_POINT ( 'NONE', #10430 ) ;
#3086=ORIENTED_EDGE ( 'NONE', *, *, #29203, .F. ) ;
#3092=CIRCLE ( 'NONE', #25726, 66.44011198581388555 ) ;
#3100=ORIENTED_EDGE ( 'NONE', *, *, #20202, .T. ) ;
#3108=EDGE_CURVE ( 'NONE', #17233, #18486, #24710, .T. ) ;
#3120=CARTESIAN_POINT ( 'NONE',  ( -29.27613032885505007, 2.267353962593735339, 79.30155859000750240 ) ) ;
#3124=CIRCLE ( 'NONE', #28819, 4.000000000000000000 ) ;
#3126=DIRECTION ( 'NONE',  ( -0.000000000000000000, 1.000000000000000000, -0.000000000000000000 ) ) ;
#3137=CARTESIAN_POINT ( 'NONE',  ( 21.09785597605719332, -16.63545420775219696, 123.7593585008393831 ) ) ;
#3145=CONICAL_SURFACE ( 'NONE', #21477, 67.36417311134205477, 1.291543646476234874 ) ;
#3149=CARTESIAN_POINT ( 'NONE',  ( -34.55638539710868429, 11.69883593934741128, 53.11441734066968934 ) ) ;
#3154=CARTESIAN_POINT ( 'NONE',  ( 51.92400919103563695, -5.935454207752202116, -13.56214536183033381 ) ) ;
#3162=CIRCLE ( 'NONE', #17846, 55.87116166729571631 ) ;
#3174=CARTESIAN_POINT ( 'NONE',  ( 21.09785597605719332, -9.935454207752199451, 47.04930799450051637 ) ) ;
#3175=EDGE_CURVE ( 'NONE', #2467, #21280, #30595, .T. ) ;
#3177=CARTESIAN_POINT ( 'NONE',  ( 21.09785597605719332, 24.56454579224780232, 47.04930799450051637 ) ) ;
#3185=CARTESIAN_POINT ( 'NONE',  ( -63.90214402394282445, -5.935454207752202116, 16.07118271501078510 ) ) ;
#3188=CARTESIAN_POINT ( 'NONE',  ( 51.52198844449087289, 5.308358430270121886, -5.044066518274861188 ) ) ;
#3191=AXIS2_PLACEMENT_3D ( 'NONE', #30328, #27374, #7354 ) ;
#3195=EDGE_CURVE ( 'NONE', #7566, #32110, #18003, .T. ) ;
#3198=B_SPLINE_CURVE_WITH_KNOTS ( 'NONE', 3,
 ( #28375, #13595, #25577, #13444, #468, #28048, #3568, #26053, #28208, #794 ),
 .UNSPECIFIED., .F., .F.,
 ( 4, 2, 2, 2, 4 ),
 ( 0.000000000000000000, 0.0008384749106984661516, 0.001257712366047681338, 0.001467331093722273319, 0.001676949821396865299 ),
 .UNSPECIFIED. ) ;
#3209=CARTESIAN_POINT ( 'NONE',  ( -9.728297238921257417, -5.935454207752202116, 106.8025418868326284 ) ) ;
#3210=AXIS2_PLACEMENT_3D ( 'NONE', #25361, #32104, #7646 ) ;
#3212=CARTESIAN_POINT ( 'NONE',  ( -35.20928760015869585, -4.023206877552709670, 80.51010491862120944 ) ) ;
#3218=VERTEX_POINT ( 'NONE', #12743 ) ;
#3224=CARTESIAN_POINT ( 'NONE',  ( -36.31236502847541914, 10.17695955431967114, 52.04930799450051637 ) ) ;
#3232=ORIENTED_EDGE ( 'NONE', *, *, #2113, .F. ) ;
#3239=CARTESIAN_POINT ( 'NONE',  ( -7.669325564611453316, 7.651854857429011503, 98.59257673948808076 ) ) ;
#3240=UNCERTAINTY_MEASURE_WITH_UNIT (LENGTH_MEASURE( 1.000000000000000082E-05 ), #27118, 'distance_accuracy_value', 'NONE');
#3258=( LENGTH_UNIT ( ) NAMED_UNIT ( * ) SI_UNIT ( .MILLI., .METRE. ) );
#3265=TOROIDAL_SURFACE ( 'NONE', #8018, 39.69941114636694834, 1.000000000000000000 ) ;
#3275=CARTESIAN_POINT ( 'NONE',  ( 21.09785597605719687, 25.56454579224779877, 87.23645172943334103 ) ) ;
#3281=ORIENTED_EDGE ( 'NONE', *, *, #3887, .F. ) ;
#3289=CARTESIAN_POINT ( 'NONE',  ( 81.48020857097124292, -5.936921830459689353, 16.01322791396358625 ) ) ;
#3292=EDGE_CURVE ( 'NONE', #7831, #23399, #14353, .T. ) ;
#3301=CYLINDRICAL_SURFACE ( 'NONE', #7374, 2.500000000000002220 ) ;
#3303=CARTESIAN_POINT ( 'NONE',  ( 21.09785597605719332, -16.93042895458276575, 47.04930799450051637 ) ) ;
#3309=ORIENTED_EDGE ( 'NONE', *, *, #32473, .F. ) ;
#3310=CIRCLE ( 'NONE', #21643, 2.500000000000002220 ) ;
#3311=DIRECTION ( 'NONE',  ( 0.000000000000000000, -9.185193130005556732E-17, 1.000000000000000000 ) ) ;
#3317=CARTESIAN_POINT ( 'NONE',  ( -39.40475928260197946, -5.936129750639523195, 77.92715501466686590 ) ) ;
#3318=ORIENTED_EDGE ( 'NONE', *, *, #17652, .F. ) ;
#3319=CIRCLE ( 'NONE', #14866, 65.75844861871132707 ) ;
#3325=CIRCLE ( 'NONE', #4907, 71.29999999999996874 ) ;
#3328=CIRCLE ( 'NONE', #2282, 2.000000000000001776 ) ;
#3329=DIRECTION ( 'NONE',  ( 0.000000000000000000, 0.000000000000000000, 1.000000000000000000 ) ) ;
#3330=PLANE ( 'NONE',  #15126 ) ;
#3335=DIRECTION ( 'NONE',  ( 0.000000000000000000, 0.000000000000000000, 1.000000000000000000 ) ) ;
#3336=EDGE_CURVE ( 'NONE', #26270, #6305, #23780, .T. ) ;
#3338=CARTESIAN_POINT ( 'NONE',  ( -2.054138246187894534, 11.56016961077985350, 98.98610059691263530 ) ) ;
#3340=( NAMED_UNIT ( * ) PLANE_ANGLE_UNIT ( ) SI_UNIT ( $, .RADIAN. ) );
#3344=B_SPLINE_CURVE_WITH_KNOTS ( 'NONE', 3,
 ( #1737, #18641, #31775, #11595, #21417, #28665, #21752, #18794, #6179, #24223, #21266, #23738, #31297, #9288 ),
 .UNSPECIFIED., .F., .F.,
 ( 4, 2, 2, 2, 2, 2, 4 ),
 ( 0.0002010756753325377709, 0.001030312595864772912, 0.001444931056130880969, 0.001859549516396989026, 0.002274167976663097300, 0.002688786436929205791, 0.003518023357461414966 ),
 .UNSPECIFIED. ) ;
#3347=DIRECTION ( 'NONE',  ( 0.000000000000000000, 0.000000000000000000, 1.000000000000000000 ) ) ;
#3356=CARTESIAN_POINT ( 'NONE',  ( 49.32263122391440646, 8.279996179725067407, -4.396176344842519512 ) ) ;
#3373=CARTESIAN_POINT ( 'NONE',  ( -31.01722238679535337, 5.224609680351743002, 77.52734172137031976 ) ) ;
#3383=CARTESIAN_POINT ( 'NONE',  ( -35.57732732147984223, 11.39140128989992817, 52.68243506491521799 ) ) ;
#3394=EDGE_CURVE ( 'NONE', #15480, #14564, #3325, .T. ) ;
#3396=CARTESIAN_POINT ( 'NONE',  ( -12.59179267514473821, -3.218976025668840002, 102.6991991216207936 ) ) ;
#3406=ORIENTED_EDGE ( 'NONE', *, *, #820, .F. ) ;
#3407=CARTESIAN_POINT ( 'NONE',  ( 71.49893360114317886, -3.295808585244882849, 11.79002343214940041 ) ) ;
#3409=VERTEX_POINT ( 'NONE', #1527 ) ;
#3424=CARTESIAN_POINT ( 'NONE',  ( 49.32092071431622315, 8.281585831149220311, 98.49472633489467910 ) ) ;
#3425=FACE_OUTER_BOUND ( 'NONE', #1946, .T. ) ;
#3441=COLOUR_RGB ( '',0.7921568627450980005, 0.8196078431372548767, 0.9333333333333333481 ) ;
#3446=CARTESIAN_POINT ( 'NONE',  ( -44.97602486328538163, -5.513888518307795472, 52.81728120461330889 ) ) ;
#3449=ORIENTED_EDGE ( 'NONE', *, *, #27458, .F. ) ;
#3451=CARTESIAN_POINT ( 'NONE',  ( 81.47887257101615432, -5.936379232154268770, 15.96372277398939588 ) ) ;
#3463=VERTEX_POINT ( 'NONE', #1859 ) ;
#3465=AXIS2_PLACEMENT_3D ( 'NONE', #24622, #14945, #2790 ) ;
#3468=CARTESIAN_POINT ( 'NONE',  ( 21.09785597605720042, -9.935454207752199451, 115.0493079945004951 ) ) ;
#3480=CARTESIAN_POINT ( 'NONE',  ( 52.07077173907278933, -5.935668157269684109, -13.53804821299738492 ) ) ;
#3482=CARTESIAN_POINT ( 'NONE',  ( 21.09785597605719332, -15.93545420775219945, 47.04930799450051637 ) ) ;
#3486=DIRECTION ( 'NONE',  ( 0.000000000000000000, 1.000000000000000000, 0.000000000000000000 ) ) ;
#3488=ORIENTED_EDGE ( 'NONE', *, *, #4254, .F. ) ;
#3493=CARTESIAN_POINT ( 'NONE',  ( -5.145516081992131951, 10.07216359114295479, 98.42132851406103100 ) ) ;
#3515=VERTEX_POINT ( 'NONE', #16463 ) ;
#3517=EDGE_CURVE ( 'NONE', #31078, #18206, #13625, .T. ) ;
#3520=EDGE_CURVE ( 'NONE', #2165, #20059, #21994, .T. ) ;
#3522=AXIS2_PLACEMENT_3D ( 'NONE', #9220, #1341, #11357 ) ;
#3550=DIRECTION ( 'NONE',  ( -0.000000000000000000, -1.000000000000000000, -0.000000000000000000 ) ) ;
#3552=CARTESIAN_POINT ( 'NONE',  ( -9.970446611220443955, -5.937394852768786535, -13.32263710021335612 ) ) ;
#3553=VERTEX_POINT ( 'NONE', #22523 ) ;
#3555=CARTESIAN_POINT ( 'NONE',  ( -6.244038915535443657, 9.161285963347376438, 98.41684214693681554 ) ) ;
#3564=FACE_OUTER_BOUND ( 'NONE', #24438, .T. ) ;
#3568=CARTESIAN_POINT ( 'NONE',  ( 52.31247960063809899, -5.928581419070744651, 106.5177822622708703 ) ) ;
#3571=ORIENTED_EDGE ( 'NONE', *, *, #22749, .F. ) ;
#3587=DIRECTION ( 'NONE',  ( -0.000000000000000000, -1.000000000000000000, -0.000000000000000000 ) ) ;
#3588=CARTESIAN_POINT ( 'NONE',  ( -34.34161333937292682, -4.095223881812850131, 13.61950888151727312 ) ) ;
#3604=SHAPE_REPRESENTATION ( 'Frame', ( #8172 ), #19670 ) ;
#3620=DIRECTION ( 'NONE',  ( 0.000000000000000000, 0.000000000000000000, -1.000000000000000000 ) ) ;
#3624=VERTEX_POINT ( 'NONE', #9744 ) ;
#3632=CARTESIAN_POINT ( 'NONE',  ( -10.74933306299440083, -5.721341737285946749, 105.3592130793008721 ) ) ;
#3640=DIRECTION ( 'NONE',  ( -3.761114140369701376E-15, -1.000000000000000000, 0.000000000000000000 ) ) ;
#3641=CIRCLE ( 'NONE', #32489, 2.500000000000002220 ) ;
#3642=ORIENTED_EDGE ( 'NONE', *, *, #31100, .T. ) ;
#3647=ORIENTED_EDGE ( 'NONE', *, *, #21276, .F. ) ;
#3649=CARTESIAN_POINT ( 'NONE',  ( 21.09785597605719332, 24.86454579224779948, 73.04930799450052348 ) ) ;
#3651=CARTESIAN_POINT ( 'NONE',  ( 71.60181765360115946, 8.510833471476306755, 19.03915849818731232 ) ) ;
#3654=AXIS2_PLACEMENT_3D ( 'NONE', #24340, #4001, #31900 ) ;
#3656=CARTESIAN_POINT ( 'NONE',  ( 21.09785597605719332, 11.92558985988973497, 47.04930799450051637 ) ) ;
#3658=CYLINDRICAL_SURFACE ( 'NONE', #9530, 10.00000000000000178 ) ;
#3666=EDGE_CURVE ( 'NONE', #17152, #7388, #17536, .T. ) ;
#3689=CARTESIAN_POINT ( 'NONE',  ( -36.06597331586808508, -5.586840335632118126, 79.16021068330404376 ) ) ;
#3691=AXIS2_PLACEMENT_3D ( 'NONE', #5934, #840, #25627 ) ;
#3692=ORIENTED_EDGE ( 'NONE', *, *, #5002, .F. ) ;
#3697=LINE ( 'NONE', #13724, #29945 ) ;
#3709=EDGE_CURVE ( 'NONE', #5045, #14332, #24600, .T. ) ;
#3720=CARTESIAN_POINT ( 'NONE',  ( 47.09785597605719687, 25.56454579224779877, 44.54930799450042400 ) ) ;
#3721=CIRCLE ( 'NONE', #8458, 0.2999999999999999334 ) ;
#3724=ORIENTED_EDGE ( 'NONE', *, *, #23274, .F. ) ;
#3726=EDGE_LOOP ( 'NONE', ( #27510, #3449 ) ) ;
#3737=VERTEX_POINT ( 'NONE', #28433 ) ;
#3740=VECTOR ( 'NONE', #4058, 1000.000000000000000 ) ;
#3748=CARTESIAN_POINT ( 'NONE',  ( -3.661041915257567947, 10.95084857405595713, -4.515295244921526674 ) ) ;
#3775=CARTESIAN_POINT ( 'NONE',  ( 74.92883917873734845, 0.05876815387845962801, 13.86745137419974050 ) ) ;
#3778=ORIENTED_EDGE ( 'NONE', *, *, #5714, .T. ) ;
#3797=DIRECTION ( 'NONE',  ( -0.000000000000000000, 1.000000000000000000, -0.000000000000000000 ) ) ;
#3812=AXIS2_PLACEMENT_3D ( 'NONE', #26913, #19184, #28897 ) ;
#3819=VECTOR ( 'NONE', #6668, 1000.000000000000114 ) ;
#3821=DIRECTION ( 'NONE',  ( -0.000000000000000000, -0.000000000000000000, -1.000000000000000000 ) ) ;
#3824=VERTEX_POINT ( 'NONE', #7070 ) ;
#3845=B_SPLINE_CURVE_WITH_KNOTS ( 'NONE', 3,
 ( #10261, #30274, #22876, #23032, #30118, #17626, #18109, #27642 ),
 .UNSPECIFIED., .F., .F.,
 ( 4, 2, 2, 4 ),
 ( 4.856180139528653963E-16, 0.0004427811193179412167, 0.0008855622386353968192, 0.001771124477270308133 ),
 .UNSPECIFIED. ) ;
#3854=CARTESIAN_POINT ( 'NONE',  ( -36.69065127708124407, -5.900665263871069932, 78.38950784583703069 ) ) ;
#3860=AXIS2_PLACEMENT_3D ( 'NONE', #25966, #13511, #18572 ) ;
#3871=DIRECTION ( 'NONE',  ( 0.000000000000000000, 0.000000000000000000, 1.000000000000000000 ) ) ;
#3878=ORIENTED_EDGE ( 'NONE', *, *, #18336, .F. ) ;
#3886=AXIS2_PLACEMENT_3D ( 'NONE', #17092, #9880, #4626 ) ;
#3887=EDGE_CURVE ( 'NONE', #13889, #32220, #14468, .T. ) ;
#3891=CARTESIAN_POINT ( 'NONE',  ( 21.09785597605720042, 16.86454579224779948, 95.68336035963606889 ) ) ;
#3900=CARTESIAN_POINT ( 'NONE',  ( -12.13387836560771582, -4.491775094913932342, -8.765527212216683850 ) ) ;
#3908=AXIS2_PLACEMENT_3D ( 'NONE', #22141, #29549, #21655 ) ;
#3911=AXIS2_PLACEMENT_3D ( 'NONE', #5524, #10130, #25056 ) ;
#3927=B_SPLINE_CURVE_WITH_KNOTS ( 'NONE', 3,
 ( #26709, #31650, #16531, #11621 ),
 .UNSPECIFIED., .F., .F.,
 ( 4, 4 ),
 ( 0.07242793514135081878, 0.08828840816840291539 ),
 .UNSPECIFIED. ) ;
#3928=EDGE_CURVE ( 'NONE', #10149, #6712, #14396, .T. ) ;
#3944=DIRECTION ( 'NONE',  ( -0.000000000000000000, -1.000000000000000000, -0.000000000000000000 ) ) ;
#3945=CARTESIAN_POINT ( 'NONE',  ( 77.48905355674300210, -4.114116020023757869, 13.63154984733677644 ) ) ;
#3978=PLANE ( 'NONE',  #24103 ) ;
#3993=CARTESIAN_POINT ( 'NONE',  ( -39.57297000773472462, -5.936060209327997939, 77.91230730958153572 ) ) ;
#4001=DIRECTION ( 'NONE',  ( 0.000000000000000000, -1.000000000000000000, 0.000000000000000000 ) ) ;
#4010=CONICAL_SURFACE ( 'NONE', #1922, 55.00000000000000000, 0.7853981633974552734 ) ;
#4011=CARTESIAN_POINT ( 'NONE',  ( 21.09785597605719332, 24.86454579224779948, 21.04930799450051282 ) ) ;
#4014=ORIENTED_EDGE ( 'NONE', *, *, #20879, .T. ) ;
#4029=DIRECTION ( 'NONE',  ( 0.000000000000000000, 0.000000000000000000, 1.000000000000000000 ) ) ;
#4032=DIRECTION ( 'NONE',  ( 0.000000000000000000, 0.000000000000000000, -1.000000000000000000 ) ) ;
#4035=CARTESIAN_POINT ( 'NONE',  ( -30.89605511857140741, 11.92558985988973497, 26.63511333407100423 ) ) ;
#4040=ADVANCED_FACE ( 'NONE', ( #23762 ), #16258, .T. ) ;
#4058=DIRECTION ( 'NONE',  ( 0.000000000000000000, -0.7071067811865426878, -0.7071067811865524577 ) ) ;
#4065=CARTESIAN_POINT ( 'NONE',  ( 106.0978559760576019, 9.702389020015065313, 20.34850893876566857 ) ) ;
#4067=CARTESIAN_POINT ( 'NONE',  ( -63.90214402394282445, -3.935454207752200340, 54.04930799450051637 ) ) ;
#4073=DIRECTION ( 'NONE',  ( 1.177206059073821606E-16, -0.2756373558169902815, 0.9612616959383214477 ) ) ;
#4076=LINE ( 'NONE', #16873, #9868 ) ;
#4081=CIRCLE ( 'NONE', #25568, 2.500000000000002220 ) ;
#4090=AXIS2_PLACEMENT_3D ( 'NONE', #29104, #1194, #5979 ) ;
#4093=CARTESIAN_POINT ( 'NONE',  ( 78.85204100697130514, -5.379633064793138963, 14.58826358935728607 ) ) ;
#4096=ORIENTED_EDGE ( 'NONE', *, *, #5611, .F. ) ;
#4098=FACE_BOUND ( 'NONE', #31253, .T. ) ;
#4107=EDGE_CURVE ( 'NONE', #28880, #11449, #6056, .T. ) ;
#4108=CARTESIAN_POINT ( 'NONE',  ( -10.50890583686613233, -5.822320178462002893, 105.8904890469746221 ) ) ;
#4112=PLANE ( 'NONE',  #5628 ) ;
#4120=AXIS2_PLACEMENT_3D ( 'NONE', #11962, #17647, #12578 ) ;
#4124=CIRCLE ( 'NONE', #7798, 3.299999999999997158 ) ;
#4130=EDGE_LOOP ( 'NONE', ( #2015, #19239 ) ) ;
#4132=CARTESIAN_POINT ( 'NONE',  ( 21.09785597605719332, 13.06454579224779877, 47.04930799450051637 ) ) ;
#4138=DIRECTION ( 'NONE',  ( -0.000000000000000000, -1.000000000000000000, -0.000000000000000000 ) ) ;
#4146=CARTESIAN_POINT ( 'NONE',  ( 21.09785597605719332, 25.13358275951983956, 47.04930799450051637 ) ) ;
#4151=CARTESIAN_POINT ( 'NONE',  ( -39.57027300287975180, -5.936134875209708284, 77.92680640967554950 ) ) ;
#4152=AXIS2_PLACEMENT_3D ( 'NONE', #17893, #13142, #15111 ) ;
#4153=DIRECTION ( 'NONE',  ( -0.000000000000000000, -0.000000000000000000, -1.000000000000000000 ) ) ;
#4163=ORIENTED_EDGE ( 'NONE', *, *, #23422, .T. ) ;
#4164=AXIS2_PLACEMENT_3D ( 'NONE', #16848, #26699, #24072 ) ;
#4167=FACE_OUTER_BOUND ( 'NONE', #5039, .T. ) ;
#4177=ADVANCED_FACE ( 'NONE', ( #19973 ), #17836, .T. ) ;
#4194=LINE ( 'NONE', #21257, #9997 ) ;
#4206=PLANE ( 'NONE',  #22692 ) ;
#4214=AXIS2_PLACEMENT_3D ( 'NONE', #27448, #4963, #19885 ) ;
#4224=DIRECTION ( 'NONE',  ( -0.000000000000000000, -1.000000000000000000, -0.000000000000000000 ) ) ;
#4229=EDGE_LOOP ( 'NONE', ( #3086, #2109, #18719, #13884, #1873, #12457, #27366, #9754, #1869, #10125, #28331, #6387, #19755, #31230, #16179, #22211 ) ) ;
#4234=DIRECTION ( 'NONE',  ( -0.000000000000000000, -1.000000000000000000, -0.000000000000000000 ) ) ;
#4241=CARTESIAN_POINT ( 'NONE',  ( 21.09785597605720042, 13.74476430820393347, -7.250692005499486115 ) ) ;
#4250=EDGE_LOOP ( 'NONE', ( #6915, #11061 ) ) ;
#4254=EDGE_CURVE ( 'NONE', #2898, #12194, #9698, .T. ) ;
#4256=CONICAL_SURFACE ( 'NONE', #10035, 54.74424859897010975, 1.291543646475813212 ) ;
#4258=ORIENTED_EDGE ( 'NONE', *, *, #16249, .T. ) ;
#4260=CARTESIAN_POINT ( 'NONE',  ( -9.728297238921268075, -5.935454207752198563, 132.0493079945005377 ) ) ;
#4262=EDGE_CURVE ( 'NONE', #14332, #21437, #12425, .T. ) ;
#4272=CARTESIAN_POINT ( 'NONE',  ( 47.79865503179234310, 9.702389020015065313, 98.41455612196619995 ) ) ;
#4276=AXIS2_PLACEMENT_3D ( 'NONE', #40, #27452, #29589 ) ;
#4282=CARTESIAN_POINT ( 'NONE',  ( -10.18637189516808661, -5.903366343041435371, 106.3819261045487536 ) ) ;
#4284=CARTESIAN_POINT ( 'NONE',  ( -12.64433984712379022, -2.833757427854236788, -8.318886203631619125 ) ) ;
#4287=FACE_OUTER_BOUND ( 'NONE', #14635, .T. ) ;
#4299=ORIENTED_EDGE ( 'NONE', *, *, #3928, .T. ) ;
#4305=CARTESIAN_POINT ( 'NONE',  ( 49.40959608158721039, 8.185031362399394439, -3.493091127261788387 ) ) ;
#4306=CARTESIAN_POINT ( 'NONE',  ( 21.09785597605719332, -16.72540370141334520, 47.04930799450051637 ) ) ;
#4307=CARTESIAN_POINT ( 'NONE',  ( 21.09785597605719332, 24.86454579224780304, 47.04930799450051637 ) ) ;
#4312=SHAPE_REPRESENTATION_RELATIONSHIP ( 'NONE' , 'NONE' ,  #3604, #11641 ) ;
#4321=CARTESIAN_POINT ( 'NONE',  ( -39.57114867957335491, -5.935958996647427988, 77.90247845943434868 ) ) ;
#4322=DIRECTION ( 'NONE',  ( -1.000000000000000000, 0.000000000000000000, 0.000000000000000000 ) ) ;
#4340=EDGE_CURVE ( 'NONE', #5527, #631, #23350, .T. ) ;
#4386=VERTEX_POINT ( 'NONE', #6657 ) ;
#4387=CARTESIAN_POINT ( 'NONE',  ( -10.13620514147193141, 3.957035103101699480, -4.501820123519951977 ) ) ;
#4408=DIRECTION ( 'NONE',  ( 0.000000000000000000, 0.000000000000000000, -1.000000000000000000 ) ) ;
#4415=ORIENTED_EDGE ( 'NONE', *, *, #14632, .F. ) ;
#4422=AXIS2_PLACEMENT_3D ( 'NONE', #8583, #27967, #715 ) ;
#4426=CARTESIAN_POINT ( 'NONE',  ( 78.30589944682461123, -4.922489993312327172, 14.14175782364709022 ) ) ;
#4429=EDGE_LOOP ( 'NONE', ( #11142, #29816 ) ) ;
#4430=TOROIDAL_SURFACE ( 'NONE', #9136, 67.99999999999997158, 3.299999999999999822 ) ;
#4439=EDGE_LOOP ( 'NONE', ( #9037, #18861 ) ) ;
#4442=ADVANCED_FACE ( 'NONE', ( #16650 ), #20994, .T. ) ;
#4444=EDGE_LOOP ( 'NONE', ( #6813, #8336, #26570, #30583, #8215, #19693 ) ) ;
#4445=CARTESIAN_POINT ( 'NONE',  ( -11.46327885171858441, 1.504766047489272562, -6.222272583143227287 ) ) ;
#4453=AXIS2_PLACEMENT_3D ( 'NONE', #1808, #8867, #23799 ) ;
#4460=DIRECTION ( 'NONE',  ( -0.000000000000000000, 1.000000000000000000, -0.000000000000000000 ) ) ;
#4466=FACE_OUTER_BOUND ( 'NONE', #10088, .T. ) ;
#4478=AXIS2_PLACEMENT_3D ( 'NONE', #32260, #12233, #29468 ) ;
#4480=CARTESIAN_POINT ( 'NONE',  ( -29.36731150373160659, 9.857091600108821794, 20.53851473532732541 ) ) ;
#4487=EDGE_LOOP ( 'NONE', ( #26246, #25574, #8529, #24402 ) ) ;
#4491=DIRECTION ( 'NONE',  ( -0.000000000000000000, 1.000000000000000000, -0.000000000000000000 ) ) ;
#4492=EDGE_CURVE ( 'NONE', #29979, #22133, #4194, .T. ) ;
#4499=CARTESIAN_POINT ( 'NONE',  ( 52.12082631206856576, -5.937449718911894436, 107.6772108465075490 ) ) ;
#4503=CARTESIAN_POINT ( 'NONE',  ( -32.42863249666554282, -1.325152302235995894, 80.65782899193297339 ) ) ;
#4504=CARTESIAN_POINT ( 'NONE',  ( -38.65545646816406133, 11.92558985988973497, 67.46350265493038023 ) ) ;
#4510=DIRECTION ( 'NONE',  ( -0.000000000000000000, -1.000000000000000000, -0.000000000000000000 ) ) ;
#4529=ORIENTED_EDGE ( 'NONE', *, *, #20159, .F. ) ;
#4530=EDGE_CURVE ( 'NONE', #7835, #22873, #541, .T. ) ;
#4546=VERTEX_POINT ( 'NONE', #9449 ) ;
#4547=CARTESIAN_POINT ( 'NONE',  ( -6.282799519003591016, 9.126991894476592648, 97.50906091218828919 ) ) ;
#4548=EDGE_LOOP ( 'NONE', ( #7695, #20621 ) ) ;
#4549=CARTESIAN_POINT ( 'NONE',  ( -11.23515816165873993, -5.485531640240842499, -9.925875039342111350 ) ) ;
#4550=ORIENTED_EDGE ( 'NONE', *, *, #32280, .F. ) ;
#4555=CARTESIAN_POINT ( 'NONE',  ( 41.51205063648687599, 11.92558985988973497, -4.944603100128015960 ) ) ;
#4558=CARTESIAN_POINT ( 'NONE',  ( 21.09785597605719332, -5.935454207752083988, 47.04930799450039558 ) ) ;
#4563=CARTESIAN_POINT ( 'NONE',  ( -38.57628410747783221, -5.432165593243111879, 14.50875660354866703 ) ) ;
#4564=VERTEX_POINT ( 'NONE', #9609 ) ;
#4565=ORIENTED_EDGE ( 'NONE', *, *, #18730, .T. ) ;
#4568=CIRCLE ( 'NONE', #23944, 39.69941114636694124 ) ;
#4569=ORIENTED_EDGE ( 'NONE', *, *, #13901, .F. ) ;
#4578=DIRECTION ( 'NONE',  ( 0.000000000000000000, 0.000000000000000000, -1.000000000000000000 ) ) ;
#4580=ORIENTED_EDGE ( 'NONE', *, *, #30075, .F. ) ;
#4586=ORIENTED_EDGE ( 'NONE', *, *, #1574, .T. ) ;
#4591=VECTOR ( 'NONE', #2541, 1000.000000000000000 ) ;
#4595=ORIENTED_EDGE ( 'NONE', *, *, #32322, .F. ) ;
#4600=CARTESIAN_POINT ( 'NONE',  ( -38.59984781516420327, -5.935454207752198563, 77.87546120947918382 ) ) ;
#4601=ORIENTED_EDGE ( 'NONE', *, *, #13315, .F. ) ;
#4617=CARTESIAN_POINT ( 'NONE',  ( 21.09785597605719332, 11.92558985988973497, 47.04930799450051637 ) ) ;
#4622=CYLINDRICAL_SURFACE ( 'NONE', #30145, 85.00000000000001421 ) ;
#4624=CARTESIAN_POINT ( 'NONE',  ( 21.09785597605719332, 24.74924423484549507, 47.04930799450051637 ) ) ;
#4626=DIRECTION ( 'NONE',  ( 0.000000000000000000, 0.000000000000000000, 1.000000000000000000 ) ) ;
#4631=DIRECTION ( 'NONE',  ( 0.000000000000000000, 0.000000000000000000, 1.000000000000000000 ) ) ;
#4634=ORIENTED_EDGE ( 'NONE', *, *, #11776, .T. ) ;
#4642=CARTESIAN_POINT ( 'NONE',  ( 80.85108986838918099, 5.388785998227653806, 77.62194537253992621 ) ) ;
#4643=VERTEX_POINT ( 'NONE', #14375 ) ;
#4687=CARTESIAN_POINT ( 'NONE',  ( -45.22799897120231094, -5.771451657996960805, 53.24836847294543674 ) ) ;
#4701=EDGE_CURVE ( 'NONE', #6259, #6661, #5339, .T. ) ;
#4707=CARTESIAN_POINT ( 'NONE',  ( -44.29239190677800053, -5.820133356959887649, 53.36605615429809291 ) ) ;
#4713=CARTESIAN_POINT ( 'NONE',  ( -6.914515305352443519, 8.508769500014659926, 97.55334879272453463 ) ) ;
#4715=CARTESIAN_POINT ( 'NONE',  ( -35.39862181984237566, -4.229295130874948683, 13.68382211909319146 ) ) ;
#4717=ORIENTED_EDGE ( 'NONE', *, *, #18469, .T. ) ;
#4721=CARTESIAN_POINT ( 'NONE',  ( 52.20930123405432965, -5.935454061169745721, 107.5404866792554799 ) ) ;
#4722=CARTESIAN_POINT ( 'NONE',  ( 21.09785597605719332, 15.06454579224778456, 47.04930799450051637 ) ) ;
#4729=DIRECTION ( 'NONE',  ( -0.000000000000000000, -1.000000000000000000, -1.446921688628131436E-16 ) ) ;
#4730=AXIS2_PLACEMENT_3D ( 'NONE', #530, #10563, #18237 ) ;
#4735=ORIENTED_EDGE ( 'NONE', *, *, #8766, .T. ) ;
#4740=ADVANCED_FACE ( 'NONE', ( #12898 ), #29218, .F. ) ;
#4747=DIRECTION ( 'NONE',  ( -0.000000000000000000, -0.000000000000000000, -1.000000000000000000 ) ) ;
#4755=EDGE_CURVE ( 'NONE', #30294, #9364, #30129, .T. ) ;
#4761=EDGE_LOOP ( 'NONE', ( #18620, #18777, #13731, #18965, #20198 ) ) ;
#4763=CARTESIAN_POINT ( 'NONE',  ( -63.90214402394282445, -5.935454207752202116, 16.07118271501078510 ) ) ;
#4770=DIRECTION ( 'NONE',  ( 0.000000000000000000, 0.000000000000000000, -1.000000000000000000 ) ) ;
#4780=VECTOR ( 'NONE', #13694, 1000.000000000000000 ) ;
#4799=CARTESIAN_POINT ( 'NONE',  ( -58.11219453028166981, -16.63545420775219696, 47.04930799450023926 ) ) ;
#4803=EDGE_LOOP ( 'NONE', ( #31160, #20007, #3642, #29614 ) ) ;
#4806=CARTESIAN_POINT ( 'NONE',  ( 21.09785597605807439, -5.935454207752083988, 47.04930799450051637 ) ) ;
#4814=EDGE_LOOP ( 'NONE', ( #11083, #7217, #16094, #23055 ) ) ;
#4821=AXIS2_PLACEMENT_3D ( 'NONE', #19444, #24370, #21740 ) ;
#4822=CARTESIAN_POINT ( 'NONE',  ( 71.88545709212758084, 11.18855628041951711, 22.82477309973399926 ) ) ;
#4832=AXIS2_PLACEMENT_3D ( 'NONE', #26622, #4138, #14162 ) ;
#4843=DIRECTION ( 'NONE',  ( -0.000000000000000000, -1.000000000000000000, 0.000000000000000000 ) ) ;
#4850=FACE_OUTER_BOUND ( 'NONE', #7607, .T. ) ;
#4872=CARTESIAN_POINT ( 'NONE',  ( 81.56333945993378620, -5.935454207834600204, 15.93786612339379083 ) ) ;
#4874=CARTESIAN_POINT ( 'NONE',  ( 47.34122803410652836, 10.07216359114295479, -4.322712525059973387 ) ) ;
#4876=DIRECTION ( 'NONE',  ( 0.000000000000000000, -1.000000000000000000, 0.000000000000000000 ) ) ;
#4880=DIRECTION ( 'NONE',  ( -0.000000000000000000, -1.000000000000000000, -0.000000000000000000 ) ) ;
#4886=FACE_OUTER_BOUND ( 'NONE', #8031, .T. ) ;
#4887=CARTESIAN_POINT ( 'NONE',  ( 52.15090187871769700, -5.936918531481693684, 107.6665413424431961 ) ) ;
#4894=CARTESIAN_POINT ( 'NONE',  ( -36.45222641229887017, 9.925589859889722533, 42.04930799450051637 ) ) ;
#4907=AXIS2_PLACEMENT_3D ( 'NONE', #25518, #10911, #567 ) ;
#4909=AXIS2_PLACEMENT_3D ( 'NONE', #8571, #3640, #1018 ) ;
#4912=CARTESIAN_POINT ( 'NONE',  ( -4.902144023942810236, 25.56454579224779877, 44.54930799450078638 ) ) ;
#4913=CARTESIAN_POINT ( 'NONE',  ( 51.67049335409638644, 5.388785998227653806, -12.70392589783158499 ) ) ;
#4916=CARTESIAN_POINT ( 'NONE',  ( 0.6836613156275018754, 1.925589859889728972, -37.95069200549950494 ) ) ;
#4921=DIRECTION ( 'NONE',  ( 0.000000000000000000, -1.000000000000000000, -0.000000000000000000 ) ) ;
#4949=TOROIDAL_SURFACE ( 'NONE', #3911, 56.00000000000000000, 1.000000000000000000 ) ;
#4951=CARTESIAN_POINT ( 'NONE',  ( 72.46310410352278097, 9.702389020015065313, 73.75010705023584023 ) ) ;
#4952=AXIS2_PLACEMENT_3D ( 'NONE', #18542, #3126, #8233 ) ;
#4961=DIRECTION ( 'NONE',  ( 0.000000000000000000, -1.000000000000000000, 0.000000000000000000 ) ) ;
#4963=DIRECTION ( 'NONE',  ( -0.000000000000000000, -1.000000000000000000, -0.000000000000000000 ) ) ;
#4969=ADVANCED_FACE ( 'NONE', ( #2344 ), #11921, .F. ) ;
#4998=LINE ( 'NONE', #30113, #17691 ) ;
#5002=EDGE_CURVE ( 'NONE', #9845, #7831, #9894, .T. ) ;
#5013=CARTESIAN_POINT ( 'NONE',  ( 76.14455416958249145, -3.653843372214094387, 80.65498324892040216 ) ) ;
#5034=CIRCLE ( 'NONE', #7116, 71.29999999999996874 ) ;
#5039=EDGE_LOOP ( 'NONE', ( #6246, #6530, #31787, #5377 ) ) ;
#5041=CARTESIAN_POINT ( 'NONE',  ( -44.22675629202193903, -5.639587714294394871, 52.99386105124461466 ) ) ;
#5043=DIRECTION ( 'NONE',  ( 0.000000000000000000, 0.000000000000000000, -1.000000000000000000 ) ) ;
#5045=VERTEX_POINT ( 'NONE', #9738 ) ;
#5046=CARTESIAN_POINT ( 'NONE',  ( -12.65020122165379668, -2.578969365796068836, 101.3081496656164688 ) ) ;
#5047=EDGE_LOOP ( 'NONE', ( #821, #23775, #19329, #27376 ) ) ;
#5048=CARTESIAN_POINT ( 'NONE',  ( -35.21912017334022948, -4.034017897931858165, 13.59333530262071932 ) ) ;
#5053=DIRECTION ( 'NONE',  ( -0.000000000000000000, -1.000000000000000000, -0.000000000000000000 ) ) ;
#5054=EDGE_CURVE ( 'NONE', #29214, #18754, #26487, .T. ) ;
#5057=DIRECTION ( 'NONE',  ( 0.000000000000000000, 0.000000000000000000, 1.000000000000000000 ) ) ;
#5070=VERTEX_POINT ( 'NONE', #20063 ) ;
#5090=ORIENTED_EDGE ( 'NONE', *, *, #27637, .F. ) ;
#5095=DIRECTION ( 'NONE',  ( 1.000000000000000000, -0.000000000000000000, -0.000000000000000000 ) ) ;
#5097=CARTESIAN_POINT ( 'NONE',  ( 52.20591152541699387, -5.935668773294350054, 107.4618278357158374 ) ) ;
#5110=VERTEX_POINT ( 'NONE', #13459 ) ;
#5111=CARTESIAN_POINT ( 'NONE',  ( -38.65545646816406133, -3.086612947480494196, 80.82450247980625591 ) ) ;
#5117=DIRECTION ( 'NONE',  ( 0.000000000000000000, -1.000000000000000000, 0.000000000000000000 ) ) ;
#5124=EDGE_CURVE ( 'NONE', #13889, #26169, #22408, .T. ) ;
#5126=EDGE_CURVE ( 'NONE', #3409, #6259, #206, .T. ) ;
#5131=ORIENTED_EDGE ( 'NONE', *, *, #9830, .F. ) ;
#5135=CARTESIAN_POINT ( 'NONE',  ( 80.85108986838918099, -5.935454207752202116, 77.87546120947918382 ) ) ;
#5145=AXIS2_PLACEMENT_3D ( 'NONE', #10290, #17324, #17159 ) ;
#5172=CARTESIAN_POINT ( 'NONE',  ( 78.71125094149621759, -5.832427868686499650, 78.63111537559601061 ) ) ;
#5173=CARTESIAN_POINT ( 'NONE',  ( -9.880269303432735128, -5.935454207752202116, -13.51052302966392205 ) ) ;
#5176=CARTESIAN_POINT ( 'NONE',  ( 75.45786391719093444, -1.094061166257011664, 80.59074881016049119 ) ) ;
#5181=DIRECTION ( 'NONE',  ( -0.000000000000000000, 1.000000000000000000, -0.000000000000000000 ) ) ;
#5197=CARTESIAN_POINT ( 'NONE',  ( -44.30341829581058022, -5.862881430098965119, 53.49729029702648830 ) ) ;
#5203=CARTESIAN_POINT ( 'NONE',  ( -12.32273293319885532, -0.6526263882323729559, 100.2535347340254219 ) ) ;
#5246=VERTEX_POINT ( 'NONE', #14098 ) ;
#5254=ORIENTED_EDGE ( 'NONE', *, *, #8808, .T. ) ;
#5259=DIRECTION ( 'NONE',  ( -0.000000000000000000, 1.000000000000000000, -0.000000000000000000 ) ) ;
#5283=FACE_OUTER_BOUND ( 'NONE', #4444, .T. ) ;
#5284=CARTESIAN_POINT ( 'NONE',  ( 81.47077242904269667, -5.936694392936851195, 15.97589416290124831 ) ) ;
#5286=CARTESIAN_POINT ( 'NONE',  ( 21.09785597605719332, 13.06454579224779877, 47.04930799450051637 ) ) ;
#5289=FACE_BOUND ( 'NONE', #2744, .T. ) ;
#5298=ORIENTED_EDGE ( 'NONE', *, *, #31466, .T. ) ;
#5307=CARTESIAN_POINT ( 'NONE',  ( 21.09785597605719332, 11.92558985988973497, 47.04930799450051637 ) ) ;
#5312=B_SPLINE_CURVE_WITH_KNOTS ( 'NONE', 3,
 ( #19104, #26508, #6489, #8779, #8947, #9109, #26834, #16326, #11258, #6649 ),
 .UNSPECIFIED., .F., .F.,
 ( 4, 2, 2, 2, 4 ),
 ( 0.0006731324393515002820, 0.002417216000136425402, 0.004161299560921350414, 0.005905383121706275426, 0.007649466682491198703 ),
 .UNSPECIFIED. ) ;
#5320=EDGE_CURVE ( 'NONE', #31117, #7831, #32147, .T. ) ;
#5332=CARTESIAN_POINT ( 'NONE',  ( -10.74933306299440083, -5.721341737285946749, 105.3592130793008721 ) ) ;
#5339=B_SPLINE_CURVE_WITH_KNOTS ( 'NONE', 3,
 ( #17959, #25672, #27980, #22727 ),
 .UNSPECIFIED., .F., .F.,
 ( 4, 4 ),
 ( 0.07166325488466616933, 0.08752405979088770382 ),
 .UNSPECIFIED. ) ;
#5352=CARTESIAN_POINT ( 'NONE',  ( -38.57628410747783221, -5.906256089375805374, 15.45647446568822225 ) ) ;
#5357=CIRCLE ( 'NONE', #13236, 65.96844849472888939 ) ;
#5367=ORIENTED_EDGE ( 'NONE', *, *, #4492, .F. ) ;
#5371=CARTESIAN_POINT ( 'NONE',  ( -30.26451050232878615, 9.135310954698587338, 74.43234153126013553 ) ) ;
#5374=CARTESIAN_POINT ( 'NONE',  ( -9.278155635207900431, 5.370505999354209692, 98.20157670830246843 ) ) ;
#5377=ORIENTED_EDGE ( 'NONE', *, *, #25128, .F. ) ;
#5382=AXIS2_PLACEMENT_3D ( 'NONE', #27898, #7221, #27410 ) ;
#5399=AXIS2_PLACEMENT_3D ( 'NONE', #5725, #30999, #18345 ) ;
#5406=EDGE_CURVE ( 'NONE', #21437, #14294, #29157, .T. ) ;
#5419=DIRECTION ( 'NONE',  ( 0.000000000000000000, 0.000000000000000000, 1.000000000000000000 ) ) ;
#5427=AXIS2_PLACEMENT_3D ( 'NONE', #19961, #4876, #5043 ) ;
#5437=CARTESIAN_POINT ( 'NONE',  ( -38.03217016322641086, -5.870668399053029951, 15.62619681354832046 ) ) ;
#5438=CARTESIAN_POINT ( 'NONE',  ( -45.06166779280743384, -5.721341737285086992, 53.14897153969102561 ) ) ;
#5442=CARTESIAN_POINT ( 'NONE',  ( -38.65545646816406133, 5.786704587343633577, 77.24891569812123748 ) ) ;
#5443=DIRECTION ( 'NONE',  ( 0.000000000000000000, 0.000000000000000000, 1.000000000000000000 ) ) ;
#5454=CIRCLE ( 'NONE', #21672, 71.99999999999998579 ) ;
#5459=CARTESIAN_POINT ( 'NONE',  ( 21.09785597605719332, 12.74140866975414887, -8.821853672795185730 ) ) ;
#5466=CARTESIAN_POINT ( 'NONE',  ( -39.45773241730296377, -5.935454212835550969, 77.98461610899785512 ) ) ;
#5474=CARTESIAN_POINT ( 'NONE',  ( 47.79865503179234310, 9.702389020015065313, -37.95069200549950494 ) ) ;
#5481=CARTESIAN_POINT ( 'NONE',  ( 21.09785597605719332, -19.93545420775220123, 47.04930799450051637 ) ) ;
#5483=DIRECTION ( 'NONE',  ( 0.000000000000000000, -1.000000000000000000, 0.000000000000000000 ) ) ;
#5492=CARTESIAN_POINT ( 'NONE',  ( 74.30208271558197453, -0.6526263882323326548, 80.46989690375676219 ) ) ;
#5494=AXIS2_PLACEMENT_3D ( 'NONE', #5530, #15534, #28178 ) ;
#5505=CARTESIAN_POINT ( 'NONE',  ( 21.09785597605719332, 25.56454579224780232, -32.16074251183835031 ) ) ;
#5507=CYLINDRICAL_SURFACE ( 'NONE', #20941, 71.99999999999998579 ) ;
#5509=CARTESIAN_POINT ( 'NONE',  ( 54.63043436083805915, -3.866180060838560806, -9.113925348800353987 ) ) ;
#5513=ORIENTED_EDGE ( 'NONE', *, *, #19632, .T. ) ;
#5514=AXIS2_PLACEMENT_3D ( 'NONE', #4916, #29868, #12638 ) ;
#5515=AXIS2_PLACEMENT_3D ( 'NONE', #28903, #26586, #19354 ) ;
#5516=CIRCLE ( 'NONE', #29623, 55.85791022362053582 ) ;
#5517=CIRCLE ( 'NONE', #25933, 72.21005050633880273 ) ;
#5522=ORIENTED_EDGE ( 'NONE', *, *, #16961, .F. ) ;
#5524=CARTESIAN_POINT ( 'NONE',  ( 21.09785597605719332, 13.74476430820393347, 47.04930799450051637 ) ) ;
#5525=CARTESIAN_POINT ( 'NONE',  ( -30.33962712718416910, 8.338190197707957552, 75.22269307782707415 ) ) ;
#5527=VERTEX_POINT ( 'NONE', #10957 ) ;
#5529=ORIENTED_EDGE ( 'NONE', *, *, #6400, .T. ) ;
#5530=CARTESIAN_POINT ( 'NONE',  ( 106.0978559760575735, 11.92558985988973497, 26.63511333407112858 ) ) ;
#5531=DIRECTION ( 'NONE',  ( 0.000000000000000000, 3.761114140369702165E-15, -1.000000000000000000 ) ) ;
#5547=ADVANCED_FACE ( 'NONE', ( #15546 ), #2755, .F. ) ;
#5581=CARTESIAN_POINT ( 'NONE',  ( -9.794785901691708929, -5.936920032134867853, 107.5052597691543070 ) ) ;
#5599=CARTESIAN_POINT ( 'NONE',  ( -29.27613032885505007, 11.23353054871637013, 71.85461326257689052 ) ) ;
#5603=DIRECTION ( 'NONE',  ( 0.000000000000000000, 0.000000000000000000, 1.000000000000000000 ) ) ;
#5611=EDGE_CURVE ( 'NONE', #30781, #6259, #3344, .T. ) ;
#5618=CARTESIAN_POINT ( 'NONE',  ( -5.602943079677954685, 9.702389020015065313, -3.412202488244239884 ) ) ;
#5622=LINE ( 'NONE', #15471, #1065 ) ;
#5628=AXIS2_PLACEMENT_3D ( 'NONE', #31372, #6909, #11677 ) ;
#5637=CARTESIAN_POINT ( 'NONE',  ( 79.18332612743283505, -5.935454207752198563, 77.87546120947918382 ) ) ;
#5639=CARTESIAN_POINT ( 'NONE',  ( 76.48178494842512976, -4.032327822094600833, 13.59507165472702894 ) ) ;
#5644=LINE ( 'NONE', #17954, #17598 ) ;
#5660=CARTESIAN_POINT ( 'NONE',  ( 21.09785597605719332, 11.78014697381582643, 47.04930799450051637 ) ) ;
#5665=B_SPLINE_SURFACE_WITH_KNOTS ( 'NONE', 3, 1, ( 
 ( #23593, #13114 ),
 ( #6043, #8337 ),
 ( #20960, #13590 ),
 ( #11134, #3407 ),
 ( #25573, #6192 ),
 ( #8029, #10488 ) ),
 .UNSPECIFIED., .F., .F., .F.,
 ( 4, 1, 1, 4 ),
 ( 2, 2 ),
 ( 0.1800733115436725096, 0.4989925988945991819, 0.7849997004460342875, 1.000000000000000000 ),
 ( 0.000000000000000000, 1.000000000000000000 ),
 .UNSPECIFIED. ) ;
#5668=EDGE_CURVE ( 'NONE', #10579, #10718, #28829, .T. ) ;
#5678=DIRECTION ( 'NONE',  ( 0.000000000000000000, 0.000000000000000000, -1.000000000000000000 ) ) ;
#5696=CARTESIAN_POINT ( 'NONE',  ( 73.09176707068564838, 11.92558985988973497, 67.46350265493038023 ) ) ;
#5704=CARTESIAN_POINT ( 'NONE',  ( -9.880269303432738681, -5.935454207752202116, -13.57859485750651629 ) ) ;
#5708=ORIENTED_EDGE ( 'NONE', *, *, #15601, .F. ) ;
#5714=EDGE_CURVE ( 'NONE', #20563, #6650, #8966, .T. ) ;
#5725=CARTESIAN_POINT ( 'NONE',  ( 21.09785597605719332, 25.56454579224779877, 47.04930799450051637 ) ) ;
#5732=CARTESIAN_POINT ( 'NONE',  ( 47.79865503179234310, 9.702389020015065313, 98.41455612196619995 ) ) ;
#5733=CARTESIAN_POINT ( 'NONE',  ( 54.76993271253332551, -1.761407059904337880, 101.7633224016298925 ) ) ;
#5746=EDGE_CURVE ( 'NONE', #13269, #11793, #2548, .T. ) ;
#5762=CARTESIAN_POINT ( 'NONE',  ( 21.09785597605720042, 14.56957104541719694, 101.5543332476699305 ) ) ;
#5763=ORIENTED_EDGE ( 'NONE', *, *, #28355, .T. ) ;
#5764=CYLINDRICAL_SURFACE ( 'NONE', #448, 2.500000000000002220 ) ;
#5765=CARTESIAN_POINT ( 'NONE',  ( 81.56333945993378620, -5.935454207834600204, 15.93786612339379083 ) ) ;
#5766=CARTESIAN_POINT ( 'NONE',  ( 21.09785597605719332, 11.92558985988973497, 47.04930799450051637 ) ) ;
#5775=DIRECTION ( 'NONE',  ( 0.000000000000000000, 0.000000000000000000, -1.000000000000000000 ) ) ;
#5788=ORIENTED_EDGE ( 'NONE', *, *, #11673, .F. ) ;
#5796=CARTESIAN_POINT ( 'NONE',  ( -39.39899823193098172, -5.936009779471990377, 77.95343643848875104 ) ) ;
#5799=EDGE_CURVE ( 'NONE', #4386, #30985, #22529, .T. ) ;
#5806=DIRECTION ( 'NONE',  ( 0.000000000000000000, 0.000000000000000000, -1.000000000000000000 ) ) ;
#5829=B_SPLINE_CURVE_WITH_KNOTS ( 'NONE', 3,
 ( #8076, #15603, #23326, #837, #10862, #27361, #22263, #21611, #31645, #24403 ),
 .UNSPECIFIED., .F., .F.,
 ( 4, 2, 2, 2, 4 ),
 ( 0.000000000000000000, 0.0008791187685415481319, 0.001318678152812310976, 0.001538457844947706656, 0.001758237537083101685 ),
 .UNSPECIFIED. ) ;
#5831=CARTESIAN_POINT ( 'NONE',  ( -10.11676764852370880, -5.928581419070745540, -12.41916627326984290 ) ) ;
#5836=CARTESIAN_POINT ( 'NONE',  ( 54.83359747464948697, -2.706209967029943986, -8.239931912618725818 ) ) ;
#5843=B_SPLINE_CURVE_WITH_KNOTS ( 'NONE', 3,
 ( #28896, #1147, #21160, #31522, #8862, #9192, #19183, #23794, #18695, #31199, #1309, #16563 ),
 .UNSPECIFIED., .F., .F.,
 ( 4, 2, 2, 2, 2, 4 ),
 ( 0.0002262581842376736074, 0.001077027684495157536, 0.001927797184752641328, 0.002778566685010125121, 0.003203951435138863331, 0.003629336185267601107 ),
 .UNSPECIFIED. ) ;
#5848=CARTESIAN_POINT ( 'NONE',  ( -35.78489663495318496, -5.401021002517912173, 79.44869760013504845 ) ) ;
#5857=CARTESIAN_POINT ( 'NONE',  ( -30.49287641343807209, 11.01517781903025650, 71.67080780280015517 ) ) ;
#5858=ADVANCED_FACE ( 'NONE', ( #737 ), #9941, .T. ) ;
#5869=CARTESIAN_POINT ( 'NONE',  ( -36.45222641229887017, 9.925589859889724309, 52.04930799450051637 ) ) ;
#5879=CARTESIAN_POINT ( 'NONE',  ( -44.28695544631908376, -5.935454207752205669, 40.04930799450050216 ) ) ;
#5882=CARTESIAN_POINT ( 'NONE',  ( -12.44358483960257189, -1.094061166256872442, 101.4093159356342682 ) ) ;
#5883=EDGE_LOOP ( 'NONE', ( #31295, #1572 ) ) ;
#5895=VERTEX_POINT ( 'NONE', #20426 ) ;
#5900=CARTESIAN_POINT ( 'NONE',  ( 54.62670865243408258, -1.035104995753989954, 101.3786800976585738 ) ) ;
#5905=VERTEX_POINT ( 'NONE', #17966 ) ;
#5922=CARTESIAN_POINT ( 'NONE',  ( -44.35282064072296748, -4.283462843672324105, 52.07173525871509412 ) ) ;
#5930=ORIENTED_EDGE ( 'NONE', *, *, #1708, .T. ) ;
#5934=CARTESIAN_POINT ( 'NONE',  ( 21.09785597605719332, -19.93545420775220123, 47.04930799450051637 ) ) ;
#5939=ORIENTED_EDGE ( 'NONE', *, *, #5054, .T. ) ;
#5944=CARTESIAN_POINT ( 'NONE',  ( 51.44386815995735418, 5.417291301124356195, 98.18922675647870335 ) ) ;
#5952=ADVANCED_FACE ( 'NONE', ( #13385 ), #28155, .F. ) ;
#5957=CARTESIAN_POINT ( 'NONE',  ( -39.39870901941788617, -5.936041284844024268, 77.94996054681324438 ) ) ;
#5960=CARTESIAN_POINT ( 'NONE',  ( 51.92840300912122586, -5.935709855254033940, -13.61832391111114937 ) ) ;
#5967=DIRECTION ( 'NONE',  ( 0.000000000000000000, 0.000000000000000000, -1.000000000000000000 ) ) ;
#5968=ADVANCED_FACE ( 'NONE', ( #27660 ), #5507, .T. ) ;
#5971=VERTEX_POINT ( 'NONE', #2872 ) ;
#5977=DIRECTION ( 'NONE',  ( 1.000000000000000000, 0.000000000000000000, 0.000000000000000000 ) ) ;
#5979=DIRECTION ( 'NONE',  ( 0.000000000000000000, 0.000000000000000000, -1.000000000000000000 ) ) ;
#5981=CARTESIAN_POINT ( 'NONE',  ( 76.05035340485899553, -2.181906231263063933, 80.77867826514622607 ) ) ;
#5989=CARTESIAN_POINT ( 'NONE',  ( 21.09785597605719332, 24.86454579224779948, 23.54930799450051637 ) ) ;
#5990=CARTESIAN_POINT ( 'NONE',  ( 52.94504501510867556, -5.721341737285968065, -11.26059709029990330 ) ) ;
#5995=EDGE_CURVE ( 'NONE', #20242, #18754, #18128, .T. ) ;
#6009=CARTESIAN_POINT ( 'NONE',  ( -9.728297238921257417, -5.935454207752202116, 97.43646483284780402 ) ) ;
#6039=VERTEX_POINT ( 'NONE', #24178 ) ;
#6043=CARTESIAN_POINT ( 'NONE',  ( 80.77181806311266143, 8.310461108307681144, 18.62663443640236238 ) ) ;
#6044=EDGE_CURVE ( 'NONE', #1224, #3218, #26325, .T. ) ;
#6054=( NAMED_UNIT ( * ) PLANE_ANGLE_UNIT ( ) SI_UNIT ( $, .RADIAN. ) );
#6055=ORIENTED_EDGE ( 'NONE', *, *, #24268, .F. ) ;
#6056=LINE ( 'NONE', #28862, #25174 ) ;
#6058=CARTESIAN_POINT ( 'NONE',  ( 50.60998280159589058, 6.668192824305383404, 98.79818430532178297 ) ) ;
#6060=CARTESIAN_POINT ( 'NONE',  ( 21.09785597605720042, -5.986312001188950127, 114.4134811058425640 ) ) ;
#6064=CARTESIAN_POINT ( 'NONE',  ( -34.53047946185701988, -4.295946708764400768, 13.71755887862822476 ) ) ;
#6079=DIRECTION ( 'NONE',  ( 0.000000000000000000, 0.000000000000000000, -1.000000000000000000 ) ) ;
#6085=CARTESIAN_POINT ( 'NONE',  ( 21.09785597605719332, 24.56454579224780232, 47.04930799450051637 ) ) ;
#6089=LINE ( 'NONE', #28576, #11765 ) ;
#6091=DIRECTION ( 'NONE',  ( 0.000000000000000000, 0.000000000000000000, -1.000000000000000000 ) ) ;
#6093=ORIENTED_EDGE ( 'NONE', *, *, #22791, .T. ) ;
#6096=DIRECTION ( 'NONE',  ( 1.313185983435984691E-29, -1.000000000000000000, -3.761114140369702165E-15 ) ) ;
#6097=FACE_BOUND ( 'NONE', #18381, .T. ) ;
#6126=SURFACE_STYLE_USAGE ( .BOTH. , #28613 ) ;
#6142=CARTESIAN_POINT ( 'NONE',  ( 51.94105711998279418, 4.618558202237299071, -5.241157233405584925 ) ) ;
#6153=CARTESIAN_POINT ( 'NONE',  ( 100.3079064823960493, -16.63545420775219696, 49.54930799450134771 ) ) ;
#6165=CYLINDRICAL_SURFACE ( 'NONE', #16000, 71.29999999999996874 ) ;
#6168=ORIENTED_EDGE ( 'NONE', *, *, #20528, .T. ) ;
#6172=CARTESIAN_POINT ( 'NONE',  ( 21.09785597605719332, -5.935454207752205669, 47.04930799450050927 ) ) ;
#6179=CARTESIAN_POINT ( 'NONE',  ( -43.97745734477487645, -5.102102110272670465, 41.67880536011271175 ) ) ;
#6192=CARTESIAN_POINT ( 'NONE',  ( 71.49893360114316465, -5.983766253076982622, 14.98546771274981637 ) ) ;
#6202=DIRECTION ( 'NONE',  ( -0.000000000000000000, -1.000000000000000000, -0.000000000000000000 ) ) ;
#6216=CARTESIAN_POINT ( 'NONE',  ( 21.09785597605720042, 11.92558985988973497, -8.808602229120017668 ) ) ;
#6219=ADVANCED_FACE ( 'NONE', ( #31742 ), #2496, .F. ) ;
#6243=CARTESIAN_POINT ( 'NONE',  ( 73.18730857026689307, 5.323792735596109438, 16.63543975439153400 ) ) ;
#6246=ORIENTED_EDGE ( 'NONE', *, *, #26861, .F. ) ;
#6249=CARTESIAN_POINT ( 'NONE',  ( 21.09785597605719332, 25.56454579224779877, 73.04930799450052348 ) ) ;
#6259=VERTEX_POINT ( 'NONE', #19863 ) ;
#6286=CARTESIAN_POINT ( 'NONE',  ( 0.000000000000000000, 0.000000000000000000, 0.000000000000000000 ) ) ;
#6288=CIRCLE ( 'NONE', #4730, 48.97546517713167447 ) ;
#6291=CARTESIAN_POINT ( 'NONE',  ( 81.63175399755476747, -5.935454207809698346, 78.02743327247107175 ) ) ;
#6301=CARTESIAN_POINT ( 'NONE',  ( 0.6836613156275053171, 11.92558985988973497, 132.0493079945005377 ) ) ;
#6305=VERTEX_POINT ( 'NONE', #6912 ) ;
#6306=CARTESIAN_POINT ( 'NONE',  ( 72.77034215320227872, 11.18784031540631574, 22.82302068831501884 ) ) ;
#6313=VECTOR ( 'NONE', #19241, 1000.000000000000000 ) ;
#6321=ORIENTED_EDGE ( 'NONE', *, *, #14947, .T. ) ;
#6328=CARTESIAN_POINT ( 'NONE',  ( 79.37786958444415575, -5.721341737285090545, 15.14745076809877133 ) ) ;
#6337=VECTOR ( 'NONE', #30692, 1000.000000000000000 ) ;
#6358=AXIS2_PLACEMENT_3D ( 'NONE', #20935, #10630, #30967 ) ;
#6362=CARTESIAN_POINT ( 'NONE',  ( 21.09785597605719332, 25.56454579224779877, 23.54930799450051637 ) ) ;
#6368=ORIENTED_EDGE ( 'NONE', *, *, #820, .T. ) ;
#6372=ORIENTED_EDGE ( 'NONE', *, *, #13912, .T. ) ;
#6384=DIRECTION ( 'NONE',  ( 0.000000000000000000, 0.000000000000000000, 1.000000000000000000 ) ) ;
#6387=ORIENTED_EDGE ( 'NONE', *, *, #25885, .F. ) ;
#6398=CARTESIAN_POINT ( 'NONE',  ( -44.16105795751995799, -3.935454207752183020, 52.04930799450050927 ) ) ;
#6400=EDGE_CURVE ( 'NONE', #32220, #26256, #27172, .T. ) ;
#6406=VERTEX_POINT ( 'NONE', #24961 ) ;
#6408=EDGE_CURVE ( 'NONE', #18864, #9903, #18050, .T. ) ;
#6419=DIRECTION ( 'NONE',  ( 0.000000000000000000, 3.761114140369702165E-15, -1.000000000000000000 ) ) ;
#6431=CARTESIAN_POINT ( 'NONE',  ( -35.50889619860521407, 10.17704670261596966, 52.04930799450050927 ) ) ;
#6434=DIRECTION ( 'NONE',  ( -1.000000000000000000, -0.000000000000000000, -3.491481338843133355E-15 ) ) ;
#6445=CARTESIAN_POINT ( 'NONE',  ( 71.55936645880203173, 9.702389020015065313, 20.34850893876554423 ) ) ;
#6448=EDGE_CURVE ( 'NONE', #7700, #27037, #10193, .T. ) ;
#6458=CARTESIAN_POINT ( 'NONE',  ( 81.57562808514117592, -5.935708903123444458, 78.02297485689277323 ) ) ;
#6465=ORIENTED_EDGE ( 'NONE', *, *, #11344, .T. ) ;
#6469=CARTESIAN_POINT ( 'NONE',  ( 49.52052953415556402, 8.310461108307681144, 97.45038561958638468 ) ) ;
#6474=CIRCLE ( 'NONE', #29002, 2.500000000000002220 ) ;
#6479=CARTESIAN_POINT ( 'NONE',  ( -32.17061786723157724, -0.8103308248208600517, 80.53195812376419838 ) ) ;
#6480=DIRECTION ( 'NONE',  ( 0.000000000000000000, 0.000000000000000000, -1.000000000000000000 ) ) ;
#6484=ORIENTED_EDGE ( 'NONE', *, *, #20274, .F. ) ;
#6489=CARTESIAN_POINT ( 'NONE',  ( -0.4050397648088443492, 11.88159288520707690, 98.63211136878676655 ) ) ;
#6490=ORIENTED_EDGE ( 'NONE', *, *, #32117, .T. ) ;
#6493=DIRECTION ( 'NONE',  ( 7.539678551159015339E-17, -0.7880107536067239016, 0.6156614753256557382 ) ) ;
#6499=DIRECTION ( 'NONE',  ( 0.000000000000000000, 3.759183808608825436E-15, -1.000000000000000000 ) ) ;
#6514=CIRCLE ( 'NONE', #6593, 55.67821551822382276 ) ;
#6530=ORIENTED_EDGE ( 'NONE', *, *, #5320, .T. ) ;
#6531=CARTESIAN_POINT ( 'NONE',  ( -12.63166379481645585, -2.284241381456149078, -7.028544075678079039 ) ) ;
#6546=DIRECTION ( 'NONE',  ( 0.000000000000000000, 0.000000000000000000, -1.000000000000000000 ) ) ;
#6550=DIRECTION ( 'NONE',  ( 0.000000000000000000, -1.000000000000000000, 0.000000000000000000 ) ) ;
#6571=CARTESIAN_POINT ( 'NONE',  ( 75.81187038318674354, -1.761407059904347649, 13.37723125802458490 ) ) ;
#6573=EDGE_LOOP ( 'NONE', ( #17580, #13110 ) ) ;
#6578=CARTESIAN_POINT ( 'NONE',  ( -45.72330504332163059, -5.935454207752205669, 40.04930799450050216 ) ) ;
#6593=AXIS2_PLACEMENT_3D ( 'NONE', #29090, #24481, #26306 ) ;
#6597=ORIENTED_EDGE ( 'NONE', *, *, #13062, .F. ) ;
#6608=CARTESIAN_POINT ( 'NONE',  ( 21.09785597605719332, 13.06454579224779877, 101.3493079945005064 ) ) ;
#6609=CARTESIAN_POINT ( 'NONE',  ( 21.09785597605719332, -16.63545420775219696, 47.04930799450051637 ) ) ;
#6625=EDGE_CURVE ( 'NONE', #28013, #32254, #1290, .T. ) ;
#6632=ORIENTED_EDGE ( 'NONE', *, *, #10196, .F. ) ;
#6639=B_SPLINE_CURVE_WITH_KNOTS ( 'NONE', 3,
 ( #25364, #28154, #18127, #22734, #2871, #15665, #5831, #20262, #15836, #25837 ),
 .UNSPECIFIED., .F., .F.,
 ( 4, 2, 2, 2, 4 ),
 ( 0.000000000000000000, 0.0008384749106984347097, 0.001257712366047654233, 0.001467331093722267898, 0.001676949821396881346 ),
 .UNSPECIFIED. ) ;
#6649=CARTESIAN_POINT ( 'NONE',  ( -5.602943079677954685, 9.702389020015065313, 97.51081847724526597 ) ) ;
#6650=VERTEX_POINT ( 'NONE', #6709 ) ;
#6657=CARTESIAN_POINT ( 'NONE',  ( -45.72330504332160217, -5.935454207752198563, 54.04930799450053058 ) ) ;
#6661=VERTEX_POINT ( 'NONE', #96 ) ;
#6667=ADVANCED_FACE ( 'NONE', ( #1620 ), #18257, .F. ) ;
#6668=DIRECTION ( 'NONE',  ( 8.659560562354932858E-17, -0.7071067811865474617, 0.7071067811865474617 ) ) ;
#6669=ORIENTED_EDGE ( 'NONE', *, *, #8030, .T. ) ;
#6688=DIRECTION ( 'NONE',  ( -0.000000000000000000, 1.000000000000000000, -0.000000000000000000 ) ) ;
#6690=FACE_OUTER_BOUND ( 'NONE', #27098, .T. ) ;
#6698=DIRECTION ( 'NONE',  ( 0.000000000000000000, 0.000000000000000000, -1.000000000000000000 ) ) ;
#6704=EDGE_LOOP ( 'NONE', ( #15581, #10, #9805, #21447 ) ) ;
#6706=AXIS2_PLACEMENT_3D ( 'NONE', #10992, #2671, #19893 ) ;
#6709=CARTESIAN_POINT ( 'NONE',  ( 21.09785597605719332, -16.63545420775219696, -25.16074251183828636 ) ) ;
#6711=AXIS2_PLACEMENT_3D ( 'NONE', #26336, #25699, #23236 ) ;
#6712=VERTEX_POINT ( 'NONE', #21467 ) ;
#6721=AXIS2_PLACEMENT_3D ( 'NONE', #32380, #29755, #22192 ) ;
#6725=CARTESIAN_POINT ( 'NONE',  ( 79.37786958444415575, -5.721341737285090545, 15.14745076809877133 ) ) ;
#6766=FACE_OUTER_BOUND ( 'NONE', #21262, .T. ) ;
#6777=CIRCLE ( 'NONE', #25129, 85.00000000000001421 ) ;
#6780=CARTESIAN_POINT ( 'NONE',  ( -39.56822316924148453, -5.935876471981492486, 77.89643810228372445 ) ) ;
#6789=CARTESIAN_POINT ( 'NONE',  ( 53.16169625780806740, -5.983766253076982622, 97.45038561958638468 ) ) ;
#6813=ORIENTED_EDGE ( 'NONE', *, *, #16112, .T. ) ;
#6815=DIRECTION ( 'NONE',  ( 0.000000000000000000, -1.000000000000000000, 0.000000000000000000 ) ) ;
#6828=CARTESIAN_POINT ( 'NONE',  ( -45.38823791396688989, -5.820268484099551998, 53.36341473305946437 ) ) ;
#6838=CONICAL_SURFACE ( 'NONE', #17322, 84.50502525316943547, 0.7853981633974621568 ) ;
#6840=CIRCLE ( 'NONE', #2650, 55.85791022362053582 ) ;
#6844=EDGE_CURVE ( 'NONE', #8185, #11676, #2579, .T. ) ;
#6875=CARTESIAN_POINT ( 'NONE',  ( -29.27337757263006424, 11.92829594627139933, 24.97746215641624090 ) ) ;
#6878=ORIENTED_EDGE ( 'NONE', *, *, #186, .T. ) ;
#6881=ORIENTED_EDGE ( 'NONE', *, *, #23468, .F. ) ;
#6882=AXIS2_PLACEMENT_3D ( 'NONE', #17019, #9492, #16864 ) ;
#6890=EDGE_LOOP ( 'NONE', ( #453, #30917 ) ) ;
#6909=DIRECTION ( 'NONE',  ( -0.000000000000000000, 1.000000000000000000, 0.000000000000000000 ) ) ;
#6912=CARTESIAN_POINT ( 'NONE',  ( -58.11219453028166981, -15.93545420775219945, 44.54930799450023216 ) ) ;
#6915=ORIENTED_EDGE ( 'NONE', *, *, #5124, .T. ) ;
#6926=CARTESIAN_POINT ( 'NONE',  ( 54.07257848512811194, -4.853532562205614020, -9.150780730119983275 ) ) ;
#6930=EDGE_CURVE ( 'NONE', #2726, #8315, #10608, .T. ) ;
#6932=CARTESIAN_POINT ( 'NONE',  ( 21.09785597605719332, 11.92558985988973497, 47.04930799450051637 ) ) ;
#6942=CARTESIAN_POINT ( 'NONE',  ( 21.09785597605719332, 13.06454579224779877, 102.0493079945005093 ) ) ;
#6943=CARTESIAN_POINT ( 'NONE',  ( 54.32959031772210068, -4.491775094913927013, 102.8641432012177148 ) ) ;
#6946=CARTESIAN_POINT ( 'NONE',  ( -39.57252254196389885, -5.936104880602451672, 77.91875142326841797 ) ) ;
#6947=LINE ( 'NONE', #8753, #12716 ) ;
#6954=CARTESIAN_POINT ( 'NONE',  ( 49.52052953415556402, 8.310461108307681144, 106.7232700815558957 ) ) ;
#6956=CARTESIAN_POINT ( 'NONE',  ( 71.55936645880203173, 9.702389020015065313, 20.34850893876554423 ) ) ;
#6963=ORIENTED_EDGE ( 'NONE', *, *, #15397, .F. ) ;
#6968=DIRECTION ( 'NONE',  ( 0.000000000000000000, -1.000000000000000000, 0.000000000000000000 ) ) ;
#6969=ORIENTED_EDGE ( 'NONE', *, *, #12260, .T. ) ;
#6971=ORIENTED_EDGE ( 'NONE', *, *, #11130, .F. ) ;
#6975=CARTESIAN_POINT ( 'NONE',  ( 72.15764468888175998, 11.56063108660457495, 70.19967134400259567 ) ) ;
#6988=ORIENTED_EDGE ( 'NONE', *, *, #28124, .T. ) ;
#6998=EDGE_CURVE ( 'NONE', #27103, #29811, #2370, .T. ) ;
#7002=ORIENTED_EDGE ( 'NONE', *, *, #22194, .F. ) ;
#7015=LINE ( 'NONE', #16528, #1713 ) ;
#7019=CARTESIAN_POINT ( 'NONE',  ( 52.07920815280782989, -5.935668478901860112, 107.6362644806661990 ) ) ;
#7020=DIRECTION ( 'NONE',  ( -0.000000000000000000, -1.000000000000000000, -0.000000000000000000 ) ) ;
#7048=CYLINDRICAL_SURFACE ( 'NONE', #5514, 10.00000000000000178 ) ;
#7057=CARTESIAN_POINT ( 'NONE',  ( 21.09785597605719332, 12.78350261226561280, 47.04930799450051637 ) ) ;
#7067=LINE ( 'NONE', #17561, #25617 ) ;
#7069=DIRECTION ( 'NONE',  ( -0.000000000000000000, 1.000000000000000000, -0.000000000000000000 ) ) ;
#7070=CARTESIAN_POINT ( 'NONE',  ( -5.602943079677954685, 9.702389020015065313, 97.51081847724526597 ) ) ;
#7080=ADVANCED_FACE ( 'NONE', ( #9421, #12542 ), #62, .F. ) ;
#7095=AXIS2_PLACEMENT_3D ( 'NONE', #16200, #16675, #31156 ) ;
#7104=CARTESIAN_POINT ( 'NONE',  ( -29.34881829548723786, 9.303215551142470119, 19.84796387032580967 ) ) ;
#7105=AXIS2_PLACEMENT_3D ( 'NONE', #3482, #13033, #28282 ) ;
#7106=CARTESIAN_POINT ( 'NONE',  ( 54.77221030306374416, -1.714651486836145322, 100.7893516206941342 ) ) ;
#7109=DIRECTION ( 'NONE',  ( 0.000000000000000000, 0.000000000000000000, -1.000000000000000000 ) ) ;
#7111=ORIENTED_EDGE ( 'NONE', *, *, #23868, .F. ) ;
#7116=AXIS2_PLACEMENT_3D ( 'NONE', #22131, #29369, #14766 ) ;
#7123=EDGE_CURVE ( 'NONE', #29537, #3515, #15676, .T. ) ;
#7125=EDGE_CURVE ( 'NONE', #31589, #15480, #30248, .T. ) ;
#7126=CARTESIAN_POINT ( 'NONE',  ( 52.16615856333482526, -5.937394852768787423, 107.6772108465075490 ) ) ;
#7132=CARTESIAN_POINT ( 'NONE',  ( -30.97925791506041904, 2.249770678923472378, 79.23692945862572401 ) ) ;
#7134=EDGE_LOOP ( 'NONE', ( #13048, #22772 ) ) ;
#7139=DIRECTION ( 'NONE',  ( 0.000000000000000000, -1.000000000000000000, 0.000000000000000000 ) ) ;
#7140=ORIENTED_EDGE ( 'NONE', *, *, #5320, .F. ) ;
#7141=DIRECTION ( 'NONE',  ( 0.000000000000000000, 0.000000000000000000, -1.000000000000000000 ) ) ;
#7143=CARTESIAN_POINT ( 'NONE',  ( -9.905649660384604260, -5.936382080411358508, -13.56946478339649964 ) ) ;
#7147=EDGE_LOOP ( 'NONE', ( #8126, #7980, #7277, #25868 ) ) ;
#7153=FACE_OUTER_BOUND ( 'NONE', #27737, .T. ) ;
#7155=EDGE_LOOP ( 'NONE', ( #1198, #12944 ) ) ;
#7157=AXIS2_PLACEMENT_3D ( 'NONE', #7057, #24948, #12480 ) ;
#7166=CARTESIAN_POINT ( 'NONE',  ( 76.06281145073309347, -3.543532154952161228, 13.42751279571587375 ) ) ;
#7169=FACE_OUTER_BOUND ( 'NONE', #15398, .T. ) ;
#7186=ORIENTED_EDGE ( 'NONE', *, *, #4340, .T. ) ;
#7187=CARTESIAN_POINT ( 'NONE',  ( 21.09785597605719332, 24.86454579224779948, 47.04930799450051637 ) ) ;
#7195=ORIENTED_EDGE ( 'NONE', *, *, #10167, .F. ) ;
#7205=CARTESIAN_POINT ( 'NONE',  ( 56.35042632428687881, -3.295808585244886402, -12.70392589783158499 ) ) ;
#7210=ADVANCED_FACE ( 'NONE', ( #27074 ), #4010, .T. ) ;
#7217=ORIENTED_EDGE ( 'NONE', *, *, #18967, .T. ) ;
#7221=DIRECTION ( 'NONE',  ( 3.761114140369701376E-15, 1.000000000000000000, 0.000000000000000000 ) ) ;
#7232=CIRCLE ( 'NONE', #25052, 39.69941114636694124 ) ;
#7248=VERTEX_POINT ( 'NONE', #9687 ) ;
#7249=CYLINDRICAL_SURFACE ( 'NONE', #22778, 71.29999999999996874 ) ;
#7256=EDGE_CURVE ( 'NONE', #21115, #6406, #29178, .T. ) ;
#7267=ORIENTED_EDGE ( 'NONE', *, *, #4107, .T. ) ;
#7272=EDGE_CURVE ( 'NONE', #23768, #16751, #16075, .T. ) ;
#7277=ORIENTED_EDGE ( 'NONE', *, *, #31220, .T. ) ;
#7278=CARTESIAN_POINT ( 'NONE',  ( -39.53644225062161155, -5.935901483590497740, 77.96306619390172443 ) ) ;
#7300=ORIENTED_EDGE ( 'NONE', *, *, #2553, .F. ) ;
#7304=DIRECTION ( 'NONE',  ( 0.000000000000000000, 0.000000000000000000, -1.000000000000000000 ) ) ;
#7306=CARTESIAN_POINT ( 'NONE',  ( 72.55809747643107244, 4.272108154687154880, 78.09619054489033374 ) ) ;
#7312=CARTESIAN_POINT ( 'NONE',  ( 72.70371229542294600, 7.324825086315909672, 76.07540346930043995 ) ) ;
#7314=CARTESIAN_POINT ( 'NONE',  ( 21.09785597605719332, -15.93545420775219945, -34.66074251183835031 ) ) ;
#7318=B_SPLINE_CURVE_WITH_KNOTS ( 'NONE', 3,
 ( #22551, #7639, #2703, #29962, #2538, #9930, #19930, #19762, #10421, #24866, #7963, #7306, #2385, #10103, #7477, #559, #15179, #27977, #5492, #15501, #12403, #239, #25511, #5013, #3010, #13049, #23040, #30125, #29793, #15023, #22387, #27648, #5172, #25191, #12733, #22724 ),
 .UNSPECIFIED., .F., .F.,
 ( 4, 2, 2, 2, 2, 2, 2, 2, 2, 2, 2, 2, 2, 2, 2, 2, 2, 4 ),
 ( 0.000000000000000000, 0.001327013081135465034, 0.002654026162270930068, 0.003981039243406394451, 0.005308052324541860136, 0.006635065405677324953, 0.007962078486812788902, 0.01061610464908372894, 0.01194311773021918509, 0.01327013081135464123, 0.01459714389249009564, 0.01592415697362555005, 0.01725117005476100446, 0.01857818313589645540, 0.01924168967646419648, 0.01990519621703193062, 0.02056870275759966823, 0.02123220929816740585 ),
 .UNSPECIFIED. ) ;
#7322=ORIENTED_EDGE ( 'NONE', *, *, #7125, .T. ) ;
#7334=CARTESIAN_POINT ( 'NONE',  ( -43.97612096762308198, -5.099423983826959272, 52.41794874062419751 ) ) ;
#7341=CARTESIAN_POINT ( 'NONE',  ( -36.86160217714372322, -5.510939734907921661, 14.80706798662212265 ) ) ;
#7350=EDGE_CURVE ( 'NONE', #3737, #30294, #23424, .T. ) ;
#7354=DIRECTION ( 'NONE',  ( 0.000000000000000000, 0.000000000000000000, 1.000000000000000000 ) ) ;
#7357=EDGE_CURVE ( 'NONE', #2614, #3078, #20272, .T. ) ;
#7360=CARTESIAN_POINT ( 'NONE',  ( 21.09785597605719332, -5.935454207752205669, 47.04930799450048085 ) ) ;
#7370=AXIS2_PLACEMENT_3D ( 'NONE', #24822, #7591, #29587 ) ;
#7374=AXIS2_PLACEMENT_3D ( 'NONE', #6249, #28257, #6091 ) ;
#7381=EDGE_CURVE ( 'NONE', #10189, #20217, #13711, .T. ) ;
#7388=VERTEX_POINT ( 'NONE', #19544 ) ;
#7392=EDGE_LOOP ( 'NONE', ( #26591, #27893, #18183, #30315 ) ) ;
#7398=EDGE_CURVE ( 'NONE', #13343, #2726, #22356, .T. ) ;
#7406=CARTESIAN_POINT ( 'NONE',  ( 52.20929446027399479, -5.935454354499447582, 107.4890962774978220 ) ) ;
#7409=DIRECTION ( 'NONE',  ( 0.000000000000000000, 0.000000000000000000, -1.000000000000000000 ) ) ;
#7415=EDGE_CURVE ( 'NONE', #9903, #20095, #19206, .T. ) ;
#7422=ORIENTED_EDGE ( 'NONE', *, *, #31509, .F. ) ;
#7433=DIRECTION ( 'NONE',  ( 0.000000000000000000, -1.000000000000000000, 0.000000000000000000 ) ) ;
#7439=ORIENTED_EDGE ( 'NONE', *, *, #31466, .F. ) ;
#7443=CARTESIAN_POINT ( 'NONE',  ( 71.48501281440435662, -3.295808585244886402, 82.30187834273039016 ) ) ;
#7448=ORIENTED_EDGE ( 'NONE', *, *, #15523, .T. ) ;
#7455=CARTESIAN_POINT ( 'NONE',  ( 73.09176707068579049, 11.92558985988973497, 26.63511333407100778 ) ) ;
#7476=ORIENTED_EDGE ( 'NONE', *, *, #20274, .T. ) ;
#7477=CARTESIAN_POINT ( 'NONE',  ( 73.23467398643032311, 2.044662169668950646, 79.35654811903377492 ) ) ;
#7481=CARTESIAN_POINT ( 'NONE',  ( 73.38832120396322978, 4.618558202237204924, 77.89250913842629132 ) ) ;
#7502=CARTESIAN_POINT ( 'NONE',  ( 74.08334718032483579, -0.1676091211930581248, 13.78591818875846364 ) ) ;
#7504=CARTESIAN_POINT ( 'NONE',  ( 45.32003422012917326, 11.18949478403750142, -4.624087122051892429 ) ) ;
#7512=CARTESIAN_POINT ( 'NONE',  ( -31.41155082672278454, 3.821193253715539750, 15.70784009975334250 ) ) ;
#7513=CARTESIAN_POINT ( 'NONE',  ( 80.71684048725118998, -5.935454207752202116, 16.07118271501079221 ) ) ;
#7514=ORIENTED_EDGE ( 'NONE', *, *, #21691, .F. ) ;
#7522=FACE_OUTER_BOUND ( 'NONE', #14012, .T. ) ;
#7538=EDGE_CURVE ( 'NONE', #29304, #1340, #25298, .T. ) ;
#7545=ORIENTED_EDGE ( 'NONE', *, *, #5611, .T. ) ;
#7548=CARTESIAN_POINT ( 'NONE',  ( -9.949682596861894268, -5.936967987714537820, -13.32519756455022808 ) ) ;
#7563=DIRECTION ( 'NONE',  ( 5.937205496305277864E-17, -0.8746197071393925215, 0.4848096202463429982 ) ) ;
#7565=CARTESIAN_POINT ( 'NONE',  ( 52.07598125554711999, -5.935454207752202116, 107.5832303370038403 ) ) ;
#7566=VERTEX_POINT ( 'NONE', #10202 ) ;
#7573=EDGE_CURVE ( 'NONE', #14294, #30985, #18400, .T. ) ;
#7575=CONICAL_SURFACE ( 'NONE', #30122, 54.50502525316942126, 0.7853981633974552734 ) ;
#7581=AXIS2_PLACEMENT_3D ( 'NONE', #1141, #11171, #8542 ) ;
#7582=ORIENTED_EDGE ( 'NONE', *, *, #12172, .T. ) ;
#7583=CARTESIAN_POINT ( 'NONE',  ( -29.27613032885505007, -5.472247659560185440, 79.55937378679692529 ) ) ;
#7591=DIRECTION ( 'NONE',  ( -0.000000000000000000, -1.000000000000000000, -0.000000000000000000 ) ) ;
#7592=CARTESIAN_POINT ( 'NONE',  ( 41.78468839005763158, 11.92558985988973497, 98.93617424376159875 ) ) ;
#7596=ORIENTED_EDGE ( 'NONE', *, *, #8345, .T. ) ;
#7599=EDGE_CURVE ( 'NONE', #11226, #25945, #10288, .T. ) ;
#7600=CARTESIAN_POINT ( 'NONE',  ( 54.81484111678624771, -3.025068871688596062, 101.6183422021972689 ) ) ;
#7607=EDGE_LOOP ( 'NONE', ( #15072, #15613, #17684, #15117 ) ) ;
#7608=DIRECTION ( 'NONE',  ( 0.000000000000000000, 0.000000000000000000, -1.000000000000000000 ) ) ;
#7612=CIRCLE ( 'NONE', #27513, 55.85791022362053582 ) ;
#7639=CARTESIAN_POINT ( 'NONE',  ( 71.55165960851208240, 9.421471677506302100, 74.09761384657856809 ) ) ;
#7641=CARTESIAN_POINT ( 'NONE',  ( 81.70930933238793159, -5.935454207752202116, 77.87546120947918382 ) ) ;
#7646=DIRECTION ( 'NONE',  ( 0.000000000000000000, 0.000000000000000000, -1.000000000000000000 ) ) ;
#7649=DIRECTION ( 'NONE',  ( 0.000000000000000000, 0.000000000000000000, 1.000000000000000000 ) ) ;
#7651=EDGE_CURVE ( 'NONE', #11226, #26412, #31192, .T. ) ;
#7657=AXIS2_PLACEMENT_3D ( 'NONE', #9735, #19726, #17595 ) ;
#7664=CARTESIAN_POINT ( 'NONE',  ( 77.20159755473073915, -4.768257113790719259, 14.00407067606322897 ) ) ;
#7665=CARTESIAN_POINT ( 'NONE',  ( -43.80906883710621713, -4.771375425951670302, 52.22812131641889977 ) ) ;
#7673=CARTESIAN_POINT ( 'NONE',  ( -31.70662748216360782, 2.874681785498175657, 15.18106132554749621 ) ) ;
#7691=CARTESIAN_POINT ( 'NONE',  ( 21.09785597605719332, -15.93545420775219945, 126.2593585008393831 ) ) ;
#7695=ORIENTED_EDGE ( 'NONE', *, *, #30631, .T. ) ;
#7700=VERTEX_POINT ( 'NONE', #18690 ) ;
#7717=DIRECTION ( 'NONE',  ( 0.000000000000000000, 1.000000000000000000, 0.000000000000000000 ) ) ;
#7725=CARTESIAN_POINT ( 'NONE',  ( 52.08014736722963534, -5.935653941159263702, 107.5318010694234374 ) ) ;
#7732=CIRCLE ( 'NONE', #3522, 1.000000000000000888 ) ;
#7735=AXIS2_PLACEMENT_3D ( 'NONE', #23973, #7069, #17071 ) ;
#7739=CARTESIAN_POINT ( 'NONE',  ( -29.27613032885505007, -0.7885532610349046401, 80.71350123316483405 ) ) ;
#7749=FACE_OUTER_BOUND ( 'NONE', #2547, .T. ) ;
#7756=CARTESIAN_POINT ( 'NONE',  ( -36.90670693849242667, -5.935454207752202116, 16.07118271501078510 ) ) ;
#7758=CARTESIAN_POINT ( 'NONE',  ( 21.09785597605719687, 24.56454579224780232, 7.349896848133565364 ) ) ;
#7762=CARTESIAN_POINT ( 'NONE',  ( -39.46303006544686554, -5.935456067349330844, 77.98454154827626894 ) ) ;
#7770=CARTESIAN_POINT ( 'NONE',  ( -5.602943079677954685, 9.702389020015065313, -12.62465409255485582 ) ) ;
#7783=EDGE_CURVE ( 'NONE', #18205, #1215, #17201, .T. ) ;
#7796=CARTESIAN_POINT ( 'NONE',  ( 81.60546541303523327, -5.936248947737075454, 77.89911125597754449 ) ) ;
#7798=AXIS2_PLACEMENT_3D ( 'NONE', #3468, #15309, #2979 ) ;
#7800=EDGE_LOOP ( 'NONE', ( #9294, #14881 ) ) ;
#7805=EDGE_CURVE ( 'NONE', #14564, #15480, #5034, .T. ) ;
#7807=DIRECTION ( 'NONE',  ( 0.000000000000000000, 0.000000000000000000, -1.000000000000000000 ) ) ;
#7809=CARTESIAN_POINT ( 'NONE',  ( 21.09785597605719332, -16.43545420775217281, -37.95069200549950494 ) ) ;
#7816=ADVANCED_FACE ( 'NONE', ( #2448 ), #15609, .F. ) ;
#7818=CARTESIAN_POINT ( 'NONE',  ( -9.732691057006816138, -5.935709855254034828, 107.7169399001122230 ) ) ;
#7822=VERTEX_POINT ( 'NONE', #12468 ) ;
#7825=CARTESIAN_POINT ( 'NONE',  ( 46.84924186968671478, 10.40182650318958224, -4.367473334732002499 ) ) ;
#7827=CARTESIAN_POINT ( 'NONE',  ( -31.75494777190924367, 11.92558985988973319, 67.46350265493038023 ) ) ;
#7828=DIRECTION ( 'NONE',  ( -0.000000000000000000, -1.000000000000000000, -0.000000000000000000 ) ) ;
#7829=ORIENTED_EDGE ( 'NONE', *, *, #30550, .T. ) ;
#7830=CARTESIAN_POINT ( 'NONE',  ( -9.728297238921268075, -5.935454207752198563, 105.1347781458764103 ) ) ;
#7831=VERTEX_POINT ( 'NONE', #1794 ) ;
#7832=CARTESIAN_POINT ( 'NONE',  ( -32.76246291686640433, -0.03437377967876181079, 13.81659845049603597 ) ) ;
#7834=AXIS2_PLACEMENT_3D ( 'NONE', #18466, #28494, #18142 ) ;
#7835=VERTEX_POINT ( 'NONE', #10446 ) ;
#7838=CARTESIAN_POINT ( 'NONE',  ( 81.66333222936422942, -5.936209625872264972, 15.95776322560501015 ) ) ;
#7849=CIRCLE ( 'NONE', #27779, 0.2999999999999947153 ) ;
#7851=ORIENTED_EDGE ( 'NONE', *, *, #2591, .F. ) ;
#7859=EDGE_CURVE ( 'NONE', #22567, #11560, #16420, .T. ) ;
#7892=CARTESIAN_POINT ( 'NONE',  ( 21.09785597605719332, -8.535454207752287914, -20.95069200549947652 ) ) ;
#7895=CARTESIAN_POINT ( 'NONE',  ( -31.36119014644065572, 11.88414354777924942, 25.57570259114776690 ) ) ;
#7898=AXIS2_PLACEMENT_3D ( 'NONE', #25163, #17769, #27788 ) ;
#7903=DIRECTION ( 'NONE',  ( 0.000000000000000000, -0.7880107536067239016, -0.6156614753256557382 ) ) ;
#7906=EDGE_LOOP ( 'NONE', ( #30339, #18008, #15921, #16017 ) ) ;
#7916=DIRECTION ( 'NONE',  ( 0.000000000000000000, 0.000000000000000000, -1.000000000000000000 ) ) ;
#7923=ORIENTED_EDGE ( 'NONE', *, *, #24392, .F. ) ;
#7928=CARTESIAN_POINT ( 'NONE',  ( -31.11772464322190856, 1.828802932772627399, 14.64222532548598465 ) ) ;
#7929=CARTESIAN_POINT ( 'NONE',  ( 54.36124578179943967, -0.1676091211930509361, 100.0347991987680984 ) ) ;
#7940=CARTESIAN_POINT ( 'NONE',  ( -39.39844553691329310, -5.936069987316967556, 77.94679389045192863 ) ) ;
#7963=CARTESIAN_POINT ( 'NONE',  ( 72.35058027291680105, 5.005525289648620202, 77.65196428233004156 ) ) ;
#7974=CARTESIAN_POINT ( 'NONE',  ( 21.09785597605720042, -6.704410789454799513, 114.3782204971654721 ) ) ;
#7980=ORIENTED_EDGE ( 'NONE', *, *, #18729, .T. ) ;
#7986=CARTESIAN_POINT ( 'NONE',  ( 51.92911259730841067, -5.935667572904989697, -13.50884708582312754 ) ) ;
#7987=FACE_OUTER_BOUND ( 'NONE', #27315, .T. ) ;
#8000=PLANE ( 'NONE',  #15804 ) ;
#8018=AXIS2_PLACEMENT_3D ( 'NONE', #14101, #17188, #16542 ) ;
#8021=EDGE_CURVE ( 'NONE', #13639, #29498, #30222, .T. ) ;
#8022=B_SPLINE_CURVE_WITH_KNOTS ( 'NONE', 3,
 ( #30211, #7406, #5097, #9, #30054, #10028, #17889, #19694, #17563, #7725, #2313, #7565 ),
 .UNSPECIFIED., .F., .F.,
 ( 4, 2, 2, 2, 2, 4 ),
 ( 0.0003078418816934655748, 0.0003848023521168218177, 0.0004232825873285107812, 0.0004617628225401997446, 0.0005387232929635631974, 0.0006156837633869265960 ),
 .UNSPECIFIED. ) ;
#8024=ORIENTED_EDGE ( 'NONE', *, *, #9156, .T. ) ;
#8026=B_SPLINE_SURFACE_WITH_KNOTS ( 'NONE', 3, 1, ( 
 ( #7770, #10077 ),
 ( #22039, #19580 ),
 ( #24677, #15317 ),
 ( #20074, #30103 ),
 ( #32068, #17771 ),
 ( #2195, #27791 ) ),
 .UNSPECIFIED., .F., .F., .F.,
 ( 4, 1, 1, 4 ),
 ( 2, 2 ),
 ( 0.1800733115436725096, 0.4989925988945991819, 0.7849997004460342875, 1.000000000000000000 ),
 ( 0.000000000000000000, 1.000000000000000000 ),
 .UNSPECIFIED. ) ;
#8029=CARTESIAN_POINT ( 'NONE',  ( 80.77181806311267565, -5.935454207752202116, 16.07118271501079576 ) ) ;
#8030=EDGE_CURVE ( 'NONE', #17109, #8696, #8184, .T. ) ;
#8031=EDGE_LOOP ( 'NONE', ( #19966, #10291 ) ) ;
#8044=CARTESIAN_POINT ( 'NONE',  ( 54.68827974814350767, -3.654479441960587049, 103.0408807978937347 ) ) ;
#8066=EDGE_LOOP ( 'NONE', ( #17641, #9786, #28569, #31788 ) ) ;
#8067=ORIENTED_EDGE ( 'NONE', *, *, #19664, .T. ) ;
#8072=CARTESIAN_POINT ( 'NONE',  ( -38.65545646816406133, 2.267353962593735339, 79.30155859000750240 ) ) ;
#8076=CARTESIAN_POINT ( 'NONE',  ( -37.21204910874186567, -5.721341737285086992, 78.89649703355408406 ) ) ;
#8081=CYLINDRICAL_SURFACE ( 'NONE', #16807, 10.00000000000000178 ) ;
#8100=CARTESIAN_POINT ( 'NONE',  ( -39.40864382708623737, -5.936121150865079521, 77.92057279823603722 ) ) ;
#8106=ORIENTED_EDGE ( 'NONE', *, *, #30902, .F. ) ;
#8109=DIRECTION ( 'NONE',  ( 0.000000000000000000, -1.000000000000000000, 0.000000000000000000 ) ) ;
#8118=CARTESIAN_POINT ( 'NONE',  ( 21.09785597605720397, -15.93545420775219945, -24.25069200549945947 ) ) ;
#8126=ORIENTED_EDGE ( 'NONE', *, *, #28038, .F. ) ;
#8127=CARTESIAN_POINT ( 'NONE',  ( 72.46310410352278097, 9.702389020015065313, 73.75010705023584023 ) ) ;
#8131=DIRECTION ( 'NONE',  ( -0.000000000000000000, -1.000000000000000000, -0.000000000000000000 ) ) ;
#8138=VERTEX_POINT ( 'NONE', #24195 ) ;
#8147=CARTESIAN_POINT ( 'NONE',  ( -9.774954067741020936, -5.936747322758278322, 107.7512220956005820 ) ) ;
#8151=ORIENTED_EDGE ( 'NONE', *, *, #30902, .T. ) ;
#8154=CARTESIAN_POINT ( 'NONE',  ( -35.94335002548523050, -4.770075702498624892, 80.07727748070902862 ) ) ;
#8156=ORIENTED_EDGE ( 'NONE', *, *, #12456, .T. ) ;
#8157=CARTESIAN_POINT ( 'NONE',  ( -10.16734060525942951, 3.903925281081630505, 98.61598880062605588 ) ) ;
#8158=ORIENTED_EDGE ( 'NONE', *, *, #12700, .F. ) ;
#8168=CARTESIAN_POINT ( 'NONE',  ( 21.09785597605720042, 17.56454579224779877, 96.02477317163219084 ) ) ;
#8172=AXIS2_PLACEMENT_3D ( 'NONE', #6286, #1354, #5977 ) ;
#8180=CARTESIAN_POINT ( 'NONE',  ( -11.66034778524429782, 1.102830191789060388, 100.4616804541535515 ) ) ;
#8183=ORIENTED_EDGE ( 'NONE', *, *, #1991, .T. ) ;
#8184=B_SPLINE_CURVE_WITH_KNOTS ( 'NONE', 3,
 ( #26335, #12057, #29457, #16481 ),
 .UNSPECIFIED., .F., .F.,
 ( 4, 4 ),
 ( 0.000000000000000000, 1.000000000000000000 ),
 .UNSPECIFIED. ) ;
#8185=VERTEX_POINT ( 'NONE', #25341 ) ;
#8194=VERTEX_POINT ( 'NONE', #17780 ) ;
#8197=ADVANCED_FACE ( 'NONE', ( #19752 ), #22859, .F. ) ;
#8215=ORIENTED_EDGE ( 'NONE', *, *, #5746, .F. ) ;
#8216=AXIS2_PLACEMENT_3D ( 'NONE', #4617, #30067, #23 ) ;
#8233=DIRECTION ( 'NONE',  ( 0.000000000000000000, 0.000000000000000000, 1.000000000000000000 ) ) ;
#8254=CARTESIAN_POINT ( 'NONE',  ( -35.09106279755485502, 10.89041806307759686, 52.27948292994979340 ) ) ;
#8259=CARTESIAN_POINT ( 'NONE',  ( 51.97066601985542178, -5.936747322758275658, -13.65260610659960250 ) ) ;
#8268=CARTESIAN_POINT ( 'NONE',  ( -63.90214402394282445, 11.92558985988973497, 67.46350265493038023 ) ) ;
#8270=B_SPLINE_CURVE_WITH_KNOTS ( 'NONE', 3,
 ( #20122, #27180, #27355, #22092, #12265, #29659, #30154, #7664, #19957, #5639, #15642, #7166, #17163, #22256, #32286, #22414, #14886, #9959, #29986, #15048, #7502, #25054, #2565, #12595, #18422, #31077, #9065, #15963, #16447, #21352, #13838, #11211, #3651, #13516, #8736, #6445 ),
 .UNSPECIFIED., .F., .F.,
 ( 4, 2, 2, 2, 2, 2, 2, 2, 2, 2, 2, 2, 2, 2, 2, 2, 2, 4 ),
 ( 0.000000000000000000, 0.0006656200208596524523, 0.001331240041719304905, 0.002662480083438613712, 0.003993720125157922303, 0.004659340146017577032, 0.005324960166877230894, 0.005990580187736883888, 0.006656200208596539485, 0.007987440250315827259, 0.009318680292035115900, 0.01064992033375440454, 0.01331240041719298182, 0.01464364045891227914, 0.01597488050063157472, 0.01863736058407016241, 0.01996860062578946146, 0.02129984066750875704 ),
 .UNSPECIFIED. ) ;
#8278=DIRECTION ( 'NONE',  ( 0.000000000000000000, 1.000000000000000000, 0.000000000000000000 ) ) ;
#8281=DIRECTION ( 'NONE',  ( 0.000000000000000000, -1.000000000000000000, 0.000000000000000000 ) ) ;
#8288=DIRECTION ( 'NONE',  ( 0.000000000000000000, 0.000000000000000000, 1.000000000000000000 ) ) ;
#8290=PRODUCT_DEFINITION_SHAPE ( 'NONE', 'NONE',  #25954 ) ;
#8304=ORIENTED_EDGE ( 'NONE', *, *, #3394, .F. ) ;
#8305=EDGE_CURVE ( 'NONE', #18206, #26412, #18101, .T. ) ;
#8308=CARTESIAN_POINT ( 'NONE',  ( -35.39203252561370761, -4.222325579252183658, 80.41835680688559762 ) ) ;
#8311=DIRECTION ( 'NONE',  ( -0.000000000000000000, -1.000000000000000000, -0.000000000000000000 ) ) ;
#8312=ORIENTED_EDGE ( 'NONE', *, *, #31100, .F. ) ;
#8315=VERTEX_POINT ( 'NONE', #21040 ) ;
#8317=CARTESIAN_POINT ( 'NONE',  ( -35.41180783471520499, 11.63092686814241539, 52.99606787449828715 ) ) ;
#8328=CARTESIAN_POINT ( 'NONE',  ( -9.970446611220443955, -5.937394852768786535, -13.57859485750651629 ) ) ;
#8333=CARTESIAN_POINT ( 'NONE',  ( -8.652076904411645231, 6.325917197325520824, 98.88062770172314231 ) ) ;
#8335=VERTEX_POINT ( 'NONE', #5637 ) ;
#8336=ORIENTED_EDGE ( 'NONE', *, *, #18045, .T. ) ;
#8337=CARTESIAN_POINT ( 'NONE',  ( 71.49893360114315044, 8.310461108307681144, 18.62663443640233041 ) ) ;
#8339=ORIENTED_EDGE ( 'NONE', *, *, #16699, .F. ) ;
#8345=EDGE_CURVE ( 'NONE', #8315, #8733, #11244, .T. ) ;
#8346=ADVANCED_FACE ( 'NONE', ( #30913 ), #20400, .F. ) ;
#8356=CIRCLE ( 'NONE', #13149, 71.99999999999998579 ) ;
#8362=CARTESIAN_POINT ( 'NONE',  ( -9.751947285419857891, -5.936248947737087889, 107.5569174314780838 ) ) ;
#8365=DIRECTION ( 'NONE',  ( 0.000000000000000000, 0.000000000000000000, -1.000000000000000000 ) ) ;
#8373=CIRCLE ( 'NONE', #26170, 48.63405236513555963 ) ;
#8378=AXIS2_PLACEMENT_3D ( 'NONE', #9004, #29030, #6546 ) ;
#8382=CARTESIAN_POINT ( 'NONE',  ( 21.09785597605719332, 15.56454579224779877, -1.926157182631158093 ) ) ;
#8391=FACE_OUTER_BOUND ( 'NONE', #17282, .T. ) ;
#8393=CARTESIAN_POINT ( 'NONE',  ( -30.89605511857140741, 11.92558985988973497, 26.63511333407100423 ) ) ;
#8394=DIRECTION ( 'NONE',  ( -0.000000000000000000, -0.000000000000000000, -1.000000000000000000 ) ) ;
#8414=PLANE ( 'NONE',  #4909 ) ;
#8418=EDGE_CURVE ( 'NONE', #3515, #17291, #12828, .T. ) ;
#8420=CARTESIAN_POINT ( 'NONE',  ( 51.95647403453392599, -5.936463533621009425, -13.64747408757448000 ) ) ;
#8442=DIRECTION ( 'NONE',  ( -1.000000000000000000, -0.000000000000000000, -0.000000000000000000 ) ) ;
#8452=CARTESIAN_POINT ( 'NONE',  ( 54.53781794026635055, -0.7249253372050199484, -7.132871347344132751 ) ) ;
#8458=AXIS2_PLACEMENT_3D ( 'NONE', #11710, #16612, #21703 ) ;
#8463=AXIS2_PLACEMENT_3D ( 'NONE', #29919, #7433, #509 ) ;
#8464=CARTESIAN_POINT ( 'NONE',  ( -35.20269728567959078, -4.936580443452697864, 79.94253044896541383 ) ) ;
#8466=ORIENTED_EDGE ( 'NONE', *, *, #26036, .F. ) ;
#8470=CARTESIAN_POINT ( 'NONE',  ( -7.324817582041172948, 8.310461108307681144, 97.43646483284780402 ) ) ;
#8471=AXIS2_PLACEMENT_3D ( 'NONE', #29639, #29970, #2545 ) ;
#8473=CARTESIAN_POINT ( 'NONE',  ( -37.21204910874186567, -5.721341737285086992, 78.89649703355408406 ) ) ;
#8477=CARTESIAN_POINT ( 'NONE',  ( 47.09785597605719687, 25.56454579224779877, 49.54930799450042400 ) ) ;
#8493=AXIS2_PLACEMENT_3D ( 'NONE', #31322, #4234, #25626 ) ;
#8496=ORIENTED_EDGE ( 'NONE', *, *, #22667, .F. ) ;
#8497=CARTESIAN_POINT ( 'NONE',  ( -11.05776695470940041, -5.581242224120388506, 105.1022689614296723 ) ) ;
#8514=ORIENTED_EDGE ( 'NONE', *, *, #31895, .F. ) ;
#8515=( NAMED_UNIT ( * ) SI_UNIT ( $, .STERADIAN. ) SOLID_ANGLE_UNIT ( ) );
#8518=CARTESIAN_POINT ( 'NONE',  ( 54.81458501433218800, -2.123693335316776842, 101.9715971512124497 ) ) ;
#8520=CARTESIAN_POINT ( 'NONE',  ( -9.880269303432738681, -5.935454207752202116, -10.95525492004900769 ) ) ;
#8521=CARTESIAN_POINT ( 'NONE',  ( 21.09785597605720042, 14.77459629858661572, -7.250692005499486115 ) ) ;
#8523=CARTESIAN_POINT ( 'NONE',  ( 21.09785597605719332, 25.56454579224780232, 126.2593585008393831 ) ) ;
#8524=CARTESIAN_POINT ( 'NONE',  ( -30.95419617802911105, 2.325935182154316827, 14.90144108804482492 ) ) ;
#8529=ORIENTED_EDGE ( 'NONE', *, *, #4755, .T. ) ;
#8542=DIRECTION ( 'NONE',  ( 0.000000000000000000, 0.000000000000000000, -1.000000000000000000 ) ) ;
#8546=DIRECTION ( 'NONE',  ( 1.000000000000000000, -0.000000000000000000, -0.000000000000000000 ) ) ;
#8547=CARTESIAN_POINT ( 'NONE',  ( 81.53175786463043551, -5.936215030417564265, 16.05158970249792105 ) ) ;
#8552=CYLINDRICAL_SURFACE ( 'NONE', #4952, 71.99999999999998579 ) ;
#8559=ORIENTED_EDGE ( 'NONE', *, *, #30471, .T. ) ;
#8565=CIRCLE ( 'NONE', #27428, 84.50000000000002842 ) ;
#8571=CARTESIAN_POINT ( 'NONE',  ( -9.880269303432744010, -5.935454207751966749, -37.95069200549950494 ) ) ;
#8579=CARTESIAN_POINT ( 'NONE',  ( 21.09785597605719332, -5.721341737285094098, 47.04930799450051637 ) ) ;
#8580=ORIENTED_EDGE ( 'NONE', *, *, #4107, .F. ) ;
#8583=CARTESIAN_POINT ( 'NONE',  ( 21.09785597605719332, -16.43545420775217281, 47.04930799450051637 ) ) ;
#8590=CARTESIAN_POINT ( 'NONE',  ( 21.09785597605719332, -16.63545420775219696, -29.66074251183834676 ) ) ;
#8592=FILL_AREA_STYLE ('',( #31085 ) ) ;
#8605=DIRECTION ( 'NONE',  ( -0.000000000000000000, -1.000000000000000000, -0.000000000000000000 ) ) ;
#8620=DIRECTION ( 'NONE',  ( 0.000000000000000000, 1.000000000000000000, 0.000000000000000000 ) ) ;
#8623=AXIS2_PLACEMENT_3D ( 'NONE', #16123, #28136, #31079 ) ;
#8638=CARTESIAN_POINT ( 'NONE',  ( -37.21204910874186567, -5.721341737285086992, 78.89649703355408406 ) ) ;
#8643=CARTESIAN_POINT ( 'NONE',  ( 21.09785597605719332, -16.93042895458276575, 47.04930799450051637 ) ) ;
#8649=CARTESIAN_POINT ( 'NONE',  ( 52.07598125554711999, -5.935454207752202116, 107.5832303370038403 ) ) ;
#8658=AXIS2_PLACEMENT_3D ( 'NONE', #26665, #4843, #21736 ) ;
#8661=ORIENTED_EDGE ( 'NONE', *, *, #27387, .F. ) ;
#8670=DIRECTION ( 'NONE',  ( 0.000000000000000000, -0.7880107536067239016, -0.6156614753256557382 ) ) ;
#8676=ADVANCED_FACE ( 'NONE', ( #25138 ), #4622, .T. ) ;
#8683=CARTESIAN_POINT ( 'NONE',  ( -0.6900943036979535483, 11.83469976691315217, -5.307522563224908119 ) ) ;
#8691=ORIENTED_EDGE ( 'NONE', *, *, #14464, .T. ) ;
#8693=EDGE_LOOP ( 'NONE', ( #8466, #19708, #22170, #28356 ) ) ;
#8696=VERTEX_POINT ( 'NONE', #32039 ) ;
#8711=CARTESIAN_POINT ( 'NONE',  ( 73.95065972402362320, 11.92558985988973497, 67.46350265493038023 ) ) ;
#8721=VERTEX_POINT ( 'NONE', #9720 ) ;
#8724=ORIENTED_EDGE ( 'NONE', *, *, #11673, .T. ) ;
#8733=VERTEX_POINT ( 'NONE', #19713 ) ;
#8736=CARTESIAN_POINT ( 'NONE',  ( 71.55170771239784244, 9.423225080673425680, 20.00317117731350791 ) ) ;
#8753=CARTESIAN_POINT ( 'NONE',  ( 41.51205063648687599, 11.92558985988973497, 132.0493079945005377 ) ) ;
#8759=CARTESIAN_POINT ( 'NONE',  ( 21.09785597605720042, 13.06454579224779877, -7.950692005499485404 ) ) ;
#8760=CARTESIAN_POINT ( 'NONE',  ( 54.17610357928707998, 0.3723237022605491719, -6.641372042216689309 ) ) ;
#8766=EDGE_CURVE ( 'NONE', #6406, #21115, #20163, .T. ) ;
#8773=VERTEX_POINT ( 'NONE', #18383 ) ;
#8774=CARTESIAN_POINT ( 'NONE',  ( -34.31970563170438737, 11.92558985988973674, 40.04930799450050216 ) ) ;
#8779=CARTESIAN_POINT ( 'NONE',  ( -1.498743213250539608, 11.70027025134008625, 98.27232293105659267 ) ) ;
#8791=DIRECTION ( 'NONE',  ( -1.313185983435984691E-29, 1.000000000000000000, 3.761114140369702165E-15 ) ) ;
#8792=EDGE_LOOP ( 'NONE', ( #30864, #13839, #24698, #12962 ) ) ;
#8795=ORIENTED_EDGE ( 'NONE', *, *, #17375, .T. ) ;
#8799=EDGE_CURVE ( 'NONE', #631, #5527, #31298, .T. ) ;
#8800=ORIENTED_EDGE ( 'NONE', *, *, #27255, .T. ) ;
#8808=EDGE_CURVE ( 'NONE', #24330, #9903, #26447, .T. ) ;
#8829=FACE_BOUND ( 'NONE', #23192, .T. ) ;
#8830=AXIS2_PLACEMENT_3D ( 'NONE', #13653, #6096, #6419 ) ;
#8831=DIRECTION ( 'NONE',  ( -0.000000000000000000, -1.000000000000000000, -0.000000000000000000 ) ) ;
#8844=EDGE_CURVE ( 'NONE', #29763, #24923, #27925, .T. ) ;
#8845=EDGE_LOOP ( 'NONE', ( #15856, #24222, #10962, #355 ) ) ;
#8852=AXIS2_PLACEMENT_3D ( 'NONE', #20431, #20270, #30463 ) ;
#8862=CARTESIAN_POINT ( 'NONE',  ( -35.76304971539452993, 11.10515806797928207, 41.68537764472188201 ) ) ;
#8863=CARTESIAN_POINT ( 'NONE',  ( 74.36943655370107820, 1.504766047489258574, 14.48817316672491806 ) ) ;
#8867=DIRECTION ( 'NONE',  ( 0.000000000000000000, -1.000000000000000000, 0.000000000000000000 ) ) ;
#8885=AXIS2_PLACEMENT_3D ( 'NONE', #5307, #19575, #12535 ) ;
#8891=ORIENTED_EDGE ( 'NONE', *, *, #8799, .F. ) ;
#8908=EDGE_LOOP ( 'NONE', ( #7111, #10199, #25674, #30798 ) ) ;
#8909=CIRCLE ( 'NONE', #22022, 54.21005050633881694 ) ;
#8915=ORIENTED_EDGE ( 'NONE', *, *, #24392, .T. ) ;
#8917=CARTESIAN_POINT ( 'NONE',  ( -44.97967447175503253, -5.519741149642646505, 41.28481392491793400 ) ) ;
#8927=ADVANCED_FACE ( 'NONE', ( #31679 ), #11278, .T. ) ;
#8935=VECTOR ( 'NONE', #7828, 1000.000000000000000 ) ;
#8947=CARTESIAN_POINT ( 'NONE',  ( -2.052507373444707017, 11.56063108660457495, 98.10909670732513632 ) ) ;
#8956=DIRECTION ( 'NONE',  ( 0.000000000000000000, 0.000000000000000000, 1.000000000000000000 ) ) ;
#8959=ORIENTED_EDGE ( 'NONE', *, *, #7651, .T. ) ;
#8963=CIRCLE ( 'NONE', #24688, 39.93581437244897359 ) ;
#8964=EDGE_LOOP ( 'NONE', ( #10197, #29872, #7267, #15867 ) ) ;
#8966=LINE ( 'NONE', #16507, #19823 ) ;
#8975=EDGE_CURVE ( 'NONE', #2830, #12487, #5843, .T. ) ;
#8977=CIRCLE ( 'NONE', #28906, 67.36417311134211161 ) ;
#9004=CARTESIAN_POINT ( 'NONE',  ( 21.09785597605719332, 15.56454579224779877, 47.04930799450051637 ) ) ;
#9010=CARTESIAN_POINT ( 'NONE',  ( 21.09785597605719332, -15.93545420775219945, -32.16074251183835031 ) ) ;
#9011=AXIS2_PLACEMENT_3D ( 'NONE', #29265, #31255, #19075 ) ;
#9030=ORIENTED_EDGE ( 'NONE', *, *, #1578, .F. ) ;
#9037=ORIENTED_EDGE ( 'NONE', *, *, #13324, .T. ) ;
#9041=ADVANCED_FACE ( 'NONE', ( #17052 ), #7048, .F. ) ;
#9044=ORIENTED_EDGE ( 'NONE', *, *, #15849, .T. ) ;
#9065=CARTESIAN_POINT ( 'NONE',  ( 72.54343063773337974, 4.323180411458211303, 16.03292188782365812 ) ) ;
#9067=DIRECTION ( 'NONE',  ( -0.000000000000000000, -1.000000000000000000, -0.000000000000000000 ) ) ;
#9072=CIRCLE ( 'NONE', #2800, 67.18681090792816235 ) ;
#9077=CARTESIAN_POINT ( 'NONE',  ( 81.54661244041565737, -5.936463391120013533, 77.99460177298303165 ) ) ;
#9082=CARTESIAN_POINT ( 'NONE',  ( -39.56032632130286686, -5.936105616667935791, 77.94281019529569221 ) ) ;
#9090=AXIS2_PLACEMENT_3D ( 'NONE', #440, #30806, #23091 ) ;
#9091=ORIENTED_EDGE ( 'NONE', *, *, #20814, .T. ) ;
#9098=( GEOMETRIC_REPRESENTATION_CONTEXT ( 3 ) GLOBAL_UNCERTAINTY_ASSIGNED_CONTEXT ( ( #13433 ) ) GLOBAL_UNIT_ASSIGNED_CONTEXT ( ( #3258, #6054, #8515 ) ) REPRESENTATION_CONTEXT ( 'NONE', 'WORKASPACE' ) );
#9103=CARTESIAN_POINT ( 'NONE',  ( -29.73671797196985622, 6.636213240270868674, 76.58164681996676393 ) ) ;
#9109=CARTESIAN_POINT ( 'NONE',  ( -3.122697032861657895, 11.19016079752309345, 97.83781872318185435 ) ) ;
#9110=EDGE_LOOP ( 'NONE', ( #20468, #24707, #31764, #26539 ) ) ;
#9136=AXIS2_PLACEMENT_3D ( 'NONE', #25822, #5483, #553 ) ;
#9137=AXIS2_PLACEMENT_3D ( 'NONE', #15285, #21154, #15591 ) ;
#9142=DIRECTION ( 'NONE',  ( -0.000000000000000000, 1.000000000000000000, -0.000000000000000000 ) ) ;
#9147=CARTESIAN_POINT ( 'NONE',  ( -63.90214402394282445, 11.92558985988973674, 54.04930799450053769 ) ) ;
#9156=EDGE_CURVE ( 'NONE', #10438, #28013, #23337, .T. ) ;
#9188=CONICAL_SURFACE ( 'NONE', #21759, 54.55130244989821620, 1.291543646475813212 ) ;
#9192=CARTESIAN_POINT ( 'NONE',  ( -35.51631071586560751, 11.48547954296073570, 41.32792022444346003 ) ) ;
#9209=CARTESIAN_POINT ( 'NONE',  ( -12.09164073932641870, -4.535950511381766859, -9.747560124061404707 ) ) ;
#9214=CARTESIAN_POINT ( 'NONE',  ( -63.90214402394282445, 11.92558985988973674, 40.04930799450050216 ) ) ;
#9220=CARTESIAN_POINT ( 'NONE',  ( 21.09785597605719332, 11.78014697381582643, 102.6448323059792358 ) ) ;
#9231=CARTESIAN_POINT ( 'NONE',  ( 54.78651577895161040, -1.820484904611813670, -6.751011824304275599 ) ) ;
#9242=CARTESIAN_POINT ( 'NONE',  ( -29.95217301285917699, 11.55131472896195710, 23.86477200840625912 ) ) ;
#9245=EDGE_LOOP ( 'NONE', ( #20790, #31187, #32307, #29361 ) ) ;
#9252=CARTESIAN_POINT ( 'NONE',  ( -39.57405207560572791, -5.936374393131169214, 77.91251232197767251 ) ) ;
#9256=CARTESIAN_POINT ( 'NONE',  ( 72.46983671362423252, 10.06999148276586453, 20.80324894526496138 ) ) ;
#9262=CARTESIAN_POINT ( 'NONE',  ( 52.12082631206856576, -5.937449718911894436, 107.4212530892143889 ) ) ;
#9268=CARTESIAN_POINT ( 'NONE',  ( -31.51145727905382188, 0.7402364505617297086, 79.96531199145222502 ) ) ;
#9278=CIRCLE ( 'NONE', #27630, 47.05803085792211249 ) ;
#9279=FACE_OUTER_BOUND ( 'NONE', #26566, .T. ) ;
#9284=EDGE_LOOP ( 'NONE', ( #31778, #9991, #23579, #8312 ) ) ;
#9287=ORIENTED_EDGE ( 'NONE', *, *, #7783, .T. ) ;
#9288=CARTESIAN_POINT ( 'NONE',  ( -43.35833523721898075, -3.935454207752190126, 42.04930799450051637 ) ) ;
#9289=B_SPLINE_CURVE_WITH_KNOTS ( 'NONE', 3,
 ( #21665, #11341, #21330, #14132 ),
 .UNSPECIFIED., .F., .F.,
 ( 4, 4 ),
 ( 0.07446322096370984467, 0.09032397578024474460 ),
 .UNSPECIFIED. ) ;
#9292=ORIENTED_EDGE ( 'NONE', *, *, #300, .T. ) ;
#9294=ORIENTED_EDGE ( 'NONE', *, *, #14679, .F. ) ;
#9302=EDGE_LOOP ( 'NONE', ( #4634, #22631, #7439, #27437 ) ) ;
#9324=AXIS2_PLACEMENT_3D ( 'NONE', #9010, #16704, #4408 ) ;
#9337=EDGE_CURVE ( 'NONE', #22133, #23145, #14958, .T. ) ;
#9339=ADVANCED_FACE ( 'NONE', ( #26700 ), #26384, .F. ) ;
#9347=AXIS2_PLACEMENT_3D ( 'NONE', #29459, #6968, #10533 ) ;
#9350=CIRCLE ( 'NONE', #6721, 2.500000000000002220 ) ;
#9360=DIRECTION ( 'NONE',  ( -0.000000000000000000, -1.000000000000000000, 0.000000000000000000 ) ) ;
#9364=VERTEX_POINT ( 'NONE', #30998 ) ;
#9370=CARTESIAN_POINT ( 'NONE',  ( -10.93321727514354968, 2.565965067347318662, -5.856419385355146723 ) ) ;
#9376=VECTOR ( 'NONE', #9142, 1000.000000000000000 ) ;
#9379=CIRCLE ( 'NONE', #17736, 0.2999999999999999334 ) ;
#9384=CARTESIAN_POINT ( 'NONE',  ( 21.09785597605719332, 13.74476430820393347, 47.04930799450051637 ) ) ;
#9389=CARTESIAN_POINT ( 'NONE',  ( 48.47851147111797587, 9.126991894476594425, -3.410444923187272881 ) ) ;
#9404=CARTESIAN_POINT ( 'NONE',  ( -29.45605141075584754, 10.51278159275453739, 21.50388707020794499 ) ) ;
#9421=FACE_BOUND ( 'NONE', #4130, .T. ) ;
#9436=ORIENTED_EDGE ( 'NONE', *, *, #2631, .T. ) ;
#9438=VERTEX_POINT ( 'NONE', #27357 ) ;
#9449=CARTESIAN_POINT ( 'NONE',  ( -43.35833523721896654, -3.935454207752183020, 52.04930799450050927 ) ) ;
#9456=ADVANCED_FACE ( 'NONE', ( #31956 ), #32274, .T. ) ;
#9471=ORIENTED_EDGE ( 'NONE', *, *, #25091, .F. ) ;
#9483=CARTESIAN_POINT ( 'NONE',  ( -9.475102253000542873, 5.053071141216427975, -4.190450134571573670 ) ) ;
#9485=EDGE_LOOP ( 'NONE', ( #1744, #17144, #7596, #25343 ) ) ;
#9490=CARTESIAN_POINT ( 'NONE',  ( 21.09785597605719332, 24.86454579224779948, 47.04930799450051637 ) ) ;
#9492=DIRECTION ( 'NONE',  ( -0.000000000000000000, -1.000000000000000000, -0.000000000000000000 ) ) ;
#9513=CARTESIAN_POINT ( 'NONE',  ( 56.35042632428687881, -3.295808585244886402, -3.337848843846767721 ) ) ;
#9514=CARTESIAN_POINT ( 'NONE',  ( -9.856458276043465361, -5.936245040125576189, 107.6870354947489403 ) ) ;
#9519=CARTESIAN_POINT ( 'NONE',  ( 72.64116057150748418, 7.652955895019256438, 18.28344188472927456 ) ) ;
#9530=AXIS2_PLACEMENT_3D ( 'NONE', #18583, #3821, #21529 ) ;
#9541=FACE_OUTER_BOUND ( 'NONE', #12620, .T. ) ;
#9551=LINE ( 'NONE', #21681, #30611 ) ;
#9553=CARTESIAN_POINT ( 'NONE',  ( 73.95065972402362320, 11.92558985988973497, 67.46350265493038023 ) ) ;
#9584=CARTESIAN_POINT ( 'NONE',  ( -39.39739818181173803, -5.935416493863505671, 77.98611552785908430 ) ) ;
#9585=DIRECTION ( 'NONE',  ( 1.000000000000000000, -0.000000000000000000, -0.000000000000000000 ) ) ;
#9587=CARTESIAN_POINT ( 'NONE',  ( 72.88142102655359622, 11.91446173404583853, 26.08880013017983401 ) ) ;
#9592=FACE_OUTER_BOUND ( 'NONE', #4429, .T. ) ;
#9596=CARTESIAN_POINT ( 'NONE',  ( -30.10465965134422106, 11.68564528720922979, 69.71257766022019098 ) ) ;
#9600=CARTESIAN_POINT ( 'NONE',  ( 52.02704899015044759, -5.937394935145313468, -13.65255231306078798 ) ) ;
#9601=EDGE_LOOP ( 'NONE', ( #21554, #6372, #9030, #15092, #21309 ) ) ;
#9609=CARTESIAN_POINT ( 'NONE',  ( 21.09785597605719687, 24.86454579224779948, 7.349896848133565364 ) ) ;
#9618=CARTESIAN_POINT ( 'NONE',  ( -45.58207439260966964, -5.881649745666465812, 53.58233204886106904 ) ) ;
#9625=EDGE_LOOP ( 'NONE', ( #2435, #11426, #23644, #25768 ) ) ;
#9635=EDGE_CURVE ( 'NONE', #15925, #13273, #18143, .T. ) ;
#9643=CARTESIAN_POINT ( 'NONE',  ( -32.19571876111664466, 1.434145862199238675, 14.44898717713608427 ) ) ;
#9645=ORIENTED_EDGE ( 'NONE', *, *, #26289, .T. ) ;
#9649=DIRECTION ( 'NONE',  ( 0.000000000000000000, 0.000000000000000000, -1.000000000000000000 ) ) ;
#9653=DIRECTION ( 'NONE',  ( 0.000000000000000000, 3.756723415560144304E-15, -1.000000000000000000 ) ) ;
#9654=VERTEX_POINT ( 'NONE', #2734 ) ;
#9656=CYLINDRICAL_SURFACE ( 'NONE', #15553, 10.00000000000000888 ) ;
#9659=FACE_OUTER_BOUND ( 'NONE', #26721, .T. ) ;
#9660=CARTESIAN_POINT ( 'NONE',  ( -38.57628410747783221, 8.768497289655476479, 19.08884019352816352 ) ) ;
#9671=CARTESIAN_POINT ( 'NONE',  ( 52.07597786784162253, -5.935454337261171887, -13.45772645143417634 ) ) ;
#9672=ADVANCED_FACE ( 'NONE', ( #28335 ), #4949, .F. ) ;
#9687=CARTESIAN_POINT ( 'NONE',  ( 21.09785597605719332, 25.56454579224779877, 67.04930799450050927 ) ) ;
#9698=B_SPLINE_CURVE_WITH_KNOTS ( 'NONE', 3,
 ( #2259, #19485, #7019, #12279, #17013, #12117, #4887, #17177, #32301, #27194, #4721, #22426 ),
 .UNSPECIFIED., .F., .F.,
 ( 4, 2, 2, 2, 2, 4 ),
 ( 0.000000000000000000, 7.696047042341537254E-05, 0.0001154407056351002296, 0.0001539209408467850731, 0.0002308814112701253239, 0.0003078418816934655748 ),
 .UNSPECIFIED. ) ;
#9704=DIRECTION ( 'NONE',  ( -0.000000000000000000, -1.000000000000000000, -0.000000000000000000 ) ) ;
#9720=CARTESIAN_POINT ( 'NONE',  ( -9.880269303432738681, -5.935454207752202116, -12.56967651669337727 ) ) ;
#9723=CARTESIAN_POINT ( 'NONE',  ( 52.14473852644682950, 4.272108154687120241, -4.410933505873395610 ) ) ;
#9726=DIRECTION ( 'NONE',  ( 0.000000000000000000, 1.000000000000000000, 0.000000000000000000 ) ) ;
#9730=CARTESIAN_POINT ( 'NONE',  ( 21.09785597605719332, -16.63545420775219696, 47.04930799450051637 ) ) ;
#9735=CARTESIAN_POINT ( 'NONE',  ( 21.09785597605719332, -15.72540370141337007, 47.04930799450051637 ) ) ;
#9738=CARTESIAN_POINT ( 'NONE',  ( -31.75494777190924367, 11.92558985988973319, 67.46350265493038023 ) ) ;
#9740=CARTESIAN_POINT ( 'NONE',  ( 80.85108986838916678, -3.295808585244886402, 82.30187834273041858 ) ) ;
#9741=EDGE_LOOP ( 'NONE', ( #8183, #12230 ) ) ;
#9742=CARTESIAN_POINT ( 'NONE',  ( -39.56345036642217394, -5.935781861350975852, 77.89068591715864898 ) ) ;
#9744=CARTESIAN_POINT ( 'NONE',  ( -58.11219453028166981, -16.63545420775219696, 44.54930799450023216 ) ) ;
#9752=DIRECTION ( 'NONE',  ( 0.000000000000000000, -0.000000000000000000, -1.000000000000000000 ) ) ;
#9754=ORIENTED_EDGE ( 'NONE', *, *, #18730, .F. ) ;
#9770=DIRECTION ( 'NONE',  ( 0.000000000000000000, 0.000000000000000000, -1.000000000000000000 ) ) ;
#9773=CARTESIAN_POINT ( 'NONE',  ( 21.09785597605719332, 12.26495659406217342, -9.420836024117583918 ) ) ;
#9778=CARTESIAN_POINT ( 'NONE',  ( 72.45825863272662559, 9.437824910247664789, 74.07738419657177076 ) ) ;
#9780=CARTESIAN_POINT ( 'NONE',  ( 73.95065972402376531, 11.92558985988973497, 26.63511333407101134 ) ) ;
#9786=ORIENTED_EDGE ( 'NONE', *, *, #10166, .F. ) ;
#9789=PRODUCT_DEFINITION_CONTEXT ( 'detailed design', #27107, 'design' ) ;
#9791=AXIS2_PLACEMENT_3D ( 'NONE', #9384, #4460, #24809 ) ;
#9793=DIRECTION ( 'NONE',  ( 0.000000000000000000, -1.000000000000000000, 0.000000000000000000 ) ) ;
#9799=CARTESIAN_POINT ( 'NONE',  ( 41.51205063648687599, 11.92558985988973497, -5.803495753465989893 ) ) ;
#9805=ORIENTED_EDGE ( 'NONE', *, *, #12456, .F. ) ;
#9806=CARTESIAN_POINT ( 'NONE',  ( -33.75433321778603357, -2.003187929803778466, 13.34606976912072618 ) ) ;
#9808=VERTEX_POINT ( 'NONE', #10935 ) ;
#9828=AXIS2_PLACEMENT_3D ( 'NONE', #25157, #20067, #24836 ) ;
#9829=ADVANCED_FACE ( 'NONE', ( #16011 ), #7575, .F. ) ;
#9830=EDGE_CURVE ( 'NONE', #31580, #21967, #25408, .T. ) ;
#9831=ORIENTED_EDGE ( 'NONE', *, *, #28980, .F. ) ;
#9832=AXIS2_PLACEMENT_3D ( 'NONE', #4146, #21862, #22355 ) ;
#9839=CARTESIAN_POINT ( 'NONE',  ( 47.79865503179234310, 9.702389020015065313, 132.0493079945005377 ) ) ;
#9845=VERTEX_POINT ( 'NONE', #11405 ) ;
#9850=CARTESIAN_POINT ( 'NONE',  ( 52.70461778898049232, -5.822320178462010887, -11.79187305797365504 ) ) ;
#9854=ORIENTED_EDGE ( 'NONE', *, *, #3517, .T. ) ;
#9862=DIRECTION ( 'NONE',  ( -0.000000000000000000, -1.000000000000000000, -0.000000000000000000 ) ) ;
#9868=VECTOR ( 'NONE', #11317, 1000.000000000000000 ) ;
#9871=EDGE_LOOP ( 'NONE', ( #25042, #29099 ) ) ;
#9872=CARTESIAN_POINT ( 'NONE',  ( -37.21204910874187988, -5.721341737285086992, 15.20211895544695757 ) ) ;
#9873=CARTESIAN_POINT ( 'NONE',  ( 72.66553924771079664, 10.95889540305196519, 71.79150321602543272 ) ) ;
#9879=CARTESIAN_POINT ( 'NONE',  ( 53.93732357960501389, 0.8961463385898192913, -5.505979700512947161 ) ) ;
#9880=DIRECTION ( 'NONE',  ( 0.000000000000000000, -1.000000000000000000, 0.000000000000000000 ) ) ;
#9894=LINE ( 'NONE', #6942, #25541 ) ;
#9897=CARTESIAN_POINT ( 'NONE',  ( 54.71965117484201357, -3.543532154952170110, 102.0142634691762709 ) ) ;
#9902=ORIENTED_EDGE ( 'NONE', *, *, #10857, .F. ) ;
#9903=VERTEX_POINT ( 'NONE', #22834 ) ;
#9910=ADVANCED_FACE ( 'NONE', ( #10371, #5289, #27602, #29584, #27766 ), #15974, .T. ) ;
#9912=CARTESIAN_POINT ( 'NONE',  ( 72.98472222531829345, 11.92558985988973497, 26.36247558050026640 ) ) ;
#9920=CARTESIAN_POINT ( 'NONE',  ( -9.779715691639985664, -5.937448199248382963, 107.7511683020618420 ) ) ;
#9930=CARTESIAN_POINT ( 'NONE',  ( 71.74717038377868050, 7.511668073839866011, 75.93045935148319359 ) ) ;
#9932=B_SPLINE_CURVE_WITH_KNOTS ( 'NONE', 3,
 ( #11570, #19258, #18772, #28641, #1717, #26502, #16635, #31597, #26173, #13715, #11733, #19095 ),
 .UNSPECIFIED., .F., .F.,
 ( 4, 2, 2, 2, 2, 4 ),
 ( 0.0003195369756171903726, 0.0003994212195214846047, 0.0004793054634257787826, 0.0005192475853779258445, 0.0005591897073300729605, 0.0006390739512343661085 ),
 .UNSPECIFIED. ) ;
#9935=CARTESIAN_POINT ( 'NONE',  ( 72.92917568327975175, 6.325917197325471975, 76.79924087496954144 ) ) ;
#9941=TOROIDAL_SURFACE ( 'NONE', #14135, 55.59552431147871232, 1.000000000000000000 ) ;
#9949=EDGE_CURVE ( 'NONE', #13157, #8315, #17586, .T. ) ;
#9957=ORIENTED_EDGE ( 'NONE', *, *, #13716, .F. ) ;
#9958=ORIENTED_EDGE ( 'NONE', *, *, #23868, .T. ) ;
#9959=CARTESIAN_POINT ( 'NONE',  ( 74.83789960225091420, -1.714651486836151983, 13.37495366749414671 ) ) ;
#9960=CARTESIAN_POINT ( 'NONE',  ( -44.28695544631906955, -5.935454207752198563, 54.04930799450053058 ) ) ;
#9966=CARTESIAN_POINT ( 'NONE',  ( -10.12312813457659999, -5.919445383190015342, 104.9138435048736255 ) ) ;
#9968=LINE ( 'NONE', #13088, #25931 ) ;
#9971=CARTESIAN_POINT ( 'NONE',  ( 81.79971628361815306, -5.935345006353228925, 78.03023866733708758 ) ) ;
#9972=DIRECTION ( 'NONE',  ( 0.000000000000000000, 0.000000000000000000, 1.000000000000000000 ) ) ;
#9991=ORIENTED_EDGE ( 'NONE', *, *, #12950, .T. ) ;
#9997=VECTOR ( 'NONE', #14216, 1000.000000000000000 ) ;
#9999=ORIENTED_EDGE ( 'NONE', *, *, #18120, .F. ) ;
#10003=CIRCLE ( 'NONE', #24664, 54.30000000000000426 ) ;
#10028=CARTESIAN_POINT ( 'NONE',  ( 52.14539454897627024, -5.936967987714539596, 107.4238135535513976 ) ) ;
#10033=DIRECTION ( 'NONE',  ( 0.000000000000000000, -0.8746197071393925215, -0.4848096202463429982 ) ) ;
#10035=AXIS2_PLACEMENT_3D ( 'NONE', #32266, #24706, #2223 ) ;
#10051=CARTESIAN_POINT ( 'NONE',  ( 51.92400919103565116, -5.935454207752198563, -11.03616215687537583 ) ) ;
#10054=ADVANCED_FACE ( 'NONE', ( #17913 ), #24356, .F. ) ;
#10067=CARTESIAN_POINT ( 'NONE',  ( -36.05908242950876286, -5.586586463951790371, 14.92569346413818998 ) ) ;
#10072=CARTESIAN_POINT ( 'NONE',  ( 45.83851142336192908, 10.95964320463250630, -3.629547344415893662 ) ) ;
#10077=CARTESIAN_POINT ( 'NONE',  ( -5.602943079677954685, 9.702389020015065313, -3.351769630585352377 ) ) ;
#10088=EDGE_LOOP ( 'NONE', ( #27827, #6093 ) ) ;
#10089=CIRCLE ( 'NONE', #28430, 72.21005050633880273 ) ;
#10091=CARTESIAN_POINT ( 'NONE',  ( -9.779715691639985664, -5.937448199248382963, 107.4930705127871562 ) ) ;
#10094=ORIENTED_EDGE ( 'NONE', *, *, #17862, .F. ) ;
#10103=CARTESIAN_POINT ( 'NONE',  ( 72.99627843240752156, 2.793366809690255526, 78.95322653079809072 ) ) ;
#10111=ORIENTED_EDGE ( 'NONE', *, *, #22862, .F. ) ;
#10118=TOROIDAL_SURFACE ( 'NONE', #17973, 39.69941114636694834, 0.3000000000000000444 ) ;
#10125=ORIENTED_EDGE ( 'NONE', *, *, #20234, .T. ) ;
#10127=EDGE_CURVE ( 'NONE', #28880, #16169, #28563, .T. ) ;
#10128=CARTESIAN_POINT ( 'NONE',  ( -43.42571077420251413, -4.056638831137751922, 52.04930799450050216 ) ) ;
#10130=DIRECTION ( 'NONE',  ( -0.000000000000000000, 1.000000000000000000, -0.000000000000000000 ) ) ;
#10136=CARTESIAN_POINT ( 'NONE',  ( 80.69365197279370250, -5.938447472589718501, 16.00391517297267185 ) ) ;
#10139=CARTESIAN_POINT ( 'NONE',  ( 21.09785597605719332, 13.06454579224779877, 47.04930799450051637 ) ) ;
#10146=CIRCLE ( 'NONE', #19561, 65.75844861871132707 ) ;
#10149=VERTEX_POINT ( 'NONE', #4272 ) ;
#10153=EDGE_LOOP ( 'NONE', ( #4529, #24495 ) ) ;
#10165=EDGE_CURVE ( 'NONE', #4564, #5895, #19648, .T. ) ;
#10166=EDGE_CURVE ( 'NONE', #4643, #15925, #259, .T. ) ;
#10167=EDGE_CURVE ( 'NONE', #29811, #10189, #22790, .T. ) ;
#10170=CARTESIAN_POINT ( 'NONE',  ( -9.884435415115211399, -5.935653941159259261, -13.43318508042229098 ) ) ;
#10171=ADVANCED_FACE ( 'NONE', ( #31363, #11491, #29056, #4098, #29381, #11829 ), #11664, .F. ) ;
#10179=FACE_OUTER_BOUND ( 'NONE', #14129, .T. ) ;
#10180=CARTESIAN_POINT ( 'NONE',  ( 51.92400919103565116, -5.935454207752198563, -12.64839579672098679 ) ) ;
#10181=CARTESIAN_POINT ( 'NONE',  ( 52.46847310473540915, -5.884593569754288822, -12.16357552036296141 ) ) ;
#10188=CARTESIAN_POINT ( 'NONE',  ( -9.728297238921257417, -5.935454207752202116, 107.6607613508313648 ) ) ;
#10189=VERTEX_POINT ( 'NONE', #8711 ) ;
#10193=LINE ( 'NONE', #12668, #12530 ) ;
#10196=EDGE_CURVE ( 'NONE', #2614, #30294, #2837, .T. ) ;
#10197=ORIENTED_EDGE ( 'NONE', *, *, #11653, .F. ) ;
#10199=ORIENTED_EDGE ( 'NONE', *, *, #12260, .F. ) ;
#10202=CARTESIAN_POINT ( 'NONE',  ( 21.09785597605719687, 24.86454579224780304, 27.04930799450051637 ) ) ;
#10203=AXIS2_PLACEMENT_3D ( 'NONE', #20047, #5117, #24976 ) ;
#10207=CARTESIAN_POINT ( 'NONE',  ( -38.65545646816406133, 11.92829597396328012, 69.12115383893792853 ) ) ;
#10211=FACE_OUTER_BOUND ( 'NONE', #379, .T. ) ;
#10225=CARTESIAN_POINT ( 'NONE',  ( 49.10800547237058566, 8.510833471476312084, 97.55326967204440791 ) ) ;
#10232=ORIENTED_EDGE ( 'NONE', *, *, #24192, .T. ) ;
#10243=CARTESIAN_POINT ( 'NONE',  ( 21.09785597605719332, -9.935454207752199451, -20.95069200549946231 ) ) ;
#10256=AXIS2_PLACEMENT_3D ( 'NONE', #4799, #31283, #11411 ) ;
#10261=CARTESIAN_POINT ( 'NONE',  ( 80.79555976727768041, -5.935454207752198563, 77.87546120947919803 ) ) ;
#10268=CARTESIAN_POINT ( 'NONE',  ( 81.65601105638101842, -5.935667572904986145, 77.88056461575189360 ) ) ;
#10271=ORIENTED_EDGE ( 'NONE', *, *, #3520, .T. ) ;
#10275=EDGE_LOOP ( 'NONE', ( #8691, #2686, #8339, #9957, #23919, #28231 ) ) ;
#10282=ORIENTED_EDGE ( 'NONE', *, *, #15268, .F. ) ;
#10284=STYLED_ITEM ( 'NONE', ( #16126 ), #11641 ) ;
#10288=CIRCLE ( 'NONE', #30714, 84.21005050633887379 ) ;
#10289=DIRECTION ( 'NONE',  ( 0.000000000000000000, 0.000000000000000000, -1.000000000000000000 ) ) ;
#10290=CARTESIAN_POINT ( 'NONE',  ( 21.09785597605719332, 24.86454579224779948, 21.04930799450051282 ) ) ;
#10291=ORIENTED_EDGE ( 'NONE', *, *, #22667, .T. ) ;
#10295=CARTESIAN_POINT ( 'NONE',  ( -30.86343899296553417, 11.58330661098384695, 70.11433744979635208 ) ) ;
#10313=VERTEX_POINT ( 'NONE', #2619 ) ;
#10333=CARTESIAN_POINT ( 'NONE',  ( 47.09785597605719687, 25.56454579224779877, 47.04930799450042400 ) ) ;
#10336=CARTESIAN_POINT ( 'NONE',  ( 48.12516263684333495, 9.438446991585321300, 98.40972204454067196 ) ) ;
#10343=CIRCLE ( 'NONE', #27100, 2.500000000000002220 ) ;
#10345=CARTESIAN_POINT ( 'NONE',  ( -9.880269301913145341, -5.935454207809699234, 107.5832060159989965 ) ) ;
#10354=ADVANCED_FACE ( 'NONE', ( #10179 ), #30200, .F. ) ;
#10360=CARTESIAN_POINT ( 'NONE',  ( -44.16105795751995799, -3.935454207752183020, 52.04930799450050927 ) ) ;
#10363=EDGE_LOOP ( 'NONE', ( #27836, #12744 ) ) ;
#10371=FACE_BOUND ( 'NONE', #11053, .T. ) ;
#10378=ORIENTED_EDGE ( 'NONE', *, *, #10404, .T. ) ;
#10382=CARTESIAN_POINT ( 'NONE',  ( -36.59584142669144313, -5.867400066089301980, 15.57347139224829213 ) ) ;
#10390=DIRECTION ( 'NONE',  ( 0.000000000000000000, 0.000000000000000000, -1.000000000000000000 ) ) ;
#10395=DIRECTION ( 'NONE',  ( 0.000000000000000000, -1.000000000000000000, 0.000000000000000000 ) ) ;
#10404=EDGE_CURVE ( 'NONE', #16051, #10149, #27340, .T. ) ;
#10405=CARTESIAN_POINT ( 'NONE',  ( 21.09785597605720397, -19.93545420775220123, -37.25069200549950210 ) ) ;
#10417=CARTESIAN_POINT ( 'NONE',  ( -4.667471018111241321, 10.39302479005550239, -3.469166095471690969 ) ) ;
#10421=CARTESIAN_POINT ( 'NONE',  ( 72.06126861588310817, 6.094407115496644600, 76.95590581573344480 ) ) ;
#10430=CARTESIAN_POINT ( 'NONE',  ( 21.09785597605719332, 13.74476430820393347, 101.3493079945005064 ) ) ;
#10438=VERTEX_POINT ( 'NONE', #25431 ) ;
#10446=CARTESIAN_POINT ( 'NONE',  ( 21.09785597605719687, 25.56454579224779877, 7.349896848133565364 ) ) ;
#10457=CARTESIAN_POINT ( 'NONE',  ( -12.51953758373980463, -1.428409478025985280, 100.6377223385756565 ) ) ;
#10460=CARTESIAN_POINT ( 'NONE',  ( -6.912293520256177715, 8.510833471476315637, -3.454653683043350743 ) ) ;
#10466=CARTESIAN_POINT ( 'NONE',  ( 81.63177831856063449, -5.935454207752202116, 16.07118271501079576 ) ) ;
#10467=DIRECTION ( 'NONE',  ( 0.000000000000000000, 0.000000000000000000, -1.000000000000000000 ) ) ;
#10468=CARTESIAN_POINT ( 'NONE',  ( 21.09785597605719332, -15.93545420775219945, 47.04930799450051637 ) ) ;
#10478=LINE ( 'NONE', #22929, #13772 ) ;
#10488=CARTESIAN_POINT ( 'NONE',  ( 71.49893360114316465, -5.935454207752202116, 16.07118271501076734 ) ) ;
#10490=TOROIDAL_SURFACE ( 'NONE', #13116, 56.00000000000000000, 1.000000000000000000 ) ;
#10491=ORIENTED_EDGE ( 'NONE', *, *, #15523, .F. ) ;
#10505=CARTESIAN_POINT ( 'NONE',  ( 50.12193823907599466, 7.326690775934355138, 98.65510655449794797 ) ) ;
#10510=ORIENTED_EDGE ( 'NONE', *, *, #3887, .T. ) ;
#10511=FACE_OUTER_BOUND ( 'NONE', #8066, .T. ) ;
#10533=DIRECTION ( 'NONE',  ( 0.000000000000000000, 0.000000000000000000, -1.000000000000000000 ) ) ;
#10539=DIRECTION ( 'NONE',  ( 0.000000000000000000, -1.000000000000000000, 0.000000000000000000 ) ) ;
#10548=AXIS2_PLACEMENT_3D ( 'NONE', #23158, #25464, #15602 ) ;
#10553=EDGE_LOOP ( 'NONE', ( #10094, #6881, #20984, #3043 ) ) ;
#10559=CARTESIAN_POINT ( 'NONE',  ( -39.46038060626020894, -5.935454093830753841, 77.98462090466851748 ) ) ;
#10563=DIRECTION ( 'NONE',  ( 0.000000000000000000, -1.000000000000000000, 0.000000000000000000 ) ) ;
#10567=CARTESIAN_POINT ( 'NONE',  ( -39.40755539011571784, -5.935795008504334724, 77.96850645159442195 ) ) ;
#10579=VERTEX_POINT ( 'NONE', #26060 ) ;
#10583=CYLINDRICAL_SURFACE ( 'NONE', #18844, 2.000000000000001776 ) ;
#10601=CARTESIAN_POINT ( 'NONE',  ( 21.09785597605719332, 15.06454579224778456, 47.04930799450051637 ) ) ;
#10603=CARTESIAN_POINT ( 'NONE',  ( 80.79555976727768041, -5.935454207752198563, 77.87546120947919803 ) ) ;
#10608=LINE ( 'NONE', #7809, #18288 ) ;
#10609=VERTEX_POINT ( 'NONE', #14089 ) ;
#10613=ADVANCED_FACE ( 'NONE', ( #1603 ), #11624, .F. ) ;
#10619=CYLINDRICAL_SURFACE ( 'NONE', #418, 2.500000000000002220 ) ;
#10623=CARTESIAN_POINT ( 'NONE',  ( -10.97410526921440521, -5.983766253076979069, 106.8025418868326284 ) ) ;
#10624=CARTESIAN_POINT ( 'NONE',  ( 21.09785597605719332, 25.56454579224780232, 128.7593585008393973 ) ) ;
#10625=CARTESIAN_POINT ( 'NONE',  ( -30.29077459323982424, 10.19186367684678984, 73.11371490948231155 ) ) ;
#10627=EDGE_CURVE ( 'NONE', #23399, #7831, #19457, .T. ) ;
#10630=DIRECTION ( 'NONE',  ( -0.000000000000000000, -1.000000000000000000, -0.000000000000000000 ) ) ;
#10635=CARTESIAN_POINT ( 'NONE',  ( 81.61462554241957434, -5.935651417315360057, 15.94210079323268836 ) ) ;
#10636=DIRECTION ( 'NONE',  ( -0.000000000000000000, -1.000000000000000000, -0.000000000000000000 ) ) ;
#10651=CARTESIAN_POINT ( 'NONE',  ( -10.95189920273699613, 2.529769287487948048, 99.96717447621844599 ) ) ;
#10667=B_SPLINE_CURVE_WITH_KNOTS ( 'NONE', 3,
 ( #8473, #13082, #30963, #28172, #25380, #8154, #20450, #8308, #3212, #23077, #428, #13407, #30481, #18468, #12922, #23244, #28496, #20282, #17989, #598, #15210, #25223, #18144, #28336, #28010, #3373, #760, #20776, #2735, #22753, #5525, #5371, #12763, #10625, #18303, #5857, #15859, #10295, #23402, #30313, #20616, #7827 ),
 .UNSPECIFIED., .F., .F.,
 ( 4, 2, 2, 2, 2, 2, 2, 2, 2, 2, 2, 2, 2, 2, 2, 2, 2, 2, 2, 2, 4 ),
 ( 4.632855027873337708E-15, 0.0008474535421348709232, 0.001694907084265108834, 0.002542360626395347070, 0.003389814168525585088, 0.004237267710655822674, 0.005084721252786060693, 0.005932174794916298712, 0.006779628337046536730, 0.007627081879176774749, 0.008474535421307013636, 0.01016944250556750529, 0.01355925667408848338, 0.01525416375834898371, 0.01694907084260948230, 0.01864397792686998262, 0.02033888501113048294, 0.02203379209539098327, 0.02372869917965148012, 0.02542360626391198045, 0.02711851334817248771 ),
 .UNSPECIFIED. ) ;
#10674=CARTESIAN_POINT ( 'NONE',  ( 47.34391502529295082, 10.06999148276586808, 98.42128873206745254 ) ) ;
#10677=LINE ( 'NONE', #20663, #6337 ) ;
#10683=CONICAL_SURFACE ( 'NONE', #16411, 67.17122696227043832, 1.291543646476234874 ) ;
#10690=ADVANCED_FACE ( 'NONE', ( #2581 ), #29899, .T. ) ;
#10695=CIRCLE ( 'NONE', #16427, 47.39944366991822733 ) ;
#10698=ORIENTED_EDGE ( 'NONE', *, *, #1708, .F. ) ;
#10706=CARTESIAN_POINT ( 'NONE',  ( 52.67966335715245663, -5.832427868686510308, -10.56408697093867843 ) ) ;
#10709=CARTESIAN_POINT ( 'NONE',  ( 21.09785597605719332, 15.06454579224778456, -7.950692005499485404 ) ) ;
#10710=LINE ( 'NONE', #15456, #22553 ) ;
#10717=CARTESIAN_POINT ( 'NONE',  ( 48.14399279324437231, 9.423225080673427456, 97.50315973084107668 ) ) ;
#10718=VERTEX_POINT ( 'NONE', #12118 ) ;
#10721=ORIENTED_EDGE ( 'NONE', *, *, #13761, .T. ) ;
#10725=CARTESIAN_POINT ( 'NONE',  ( -34.42289002669387088, 11.86391215166791113, 53.48663982859374499 ) ) ;
#10731=CIRCLE ( 'NONE', #9137, 19.99999999999999645 ) ;
#10755=CIRCLE ( 'NONE', #14937, 65.75844861871138392 ) ;
#10758=CARTESIAN_POINT ( 'NONE',  ( 21.09785597605719332, 15.63322284159649556, 47.04930799450051637 ) ) ;
#10765=CARTESIAN_POINT ( 'NONE',  ( 48.12593217812826651, 9.437824910247671895, -4.311094662169014491 ) ) ;
#10777=CARTESIAN_POINT ( 'NONE',  ( 21.09785597605719332, 25.56454579224779877, 47.04930799450051637 ) ) ;
#10779=ORIENTED_EDGE ( 'NONE', *, *, #3108, .T. ) ;
#10782=CARTESIAN_POINT ( 'NONE',  ( -5.602943079677954685, 9.702389020015065313, 97.43646483284780402 ) ) ;
#10793=CARTESIAN_POINT ( 'NONE',  ( 81.68481246222317793, -5.935668478901866330, 16.06795581775006099 ) ) ;
#10818=ORIENTED_EDGE ( 'NONE', *, *, #19745, .F. ) ;
#10833=DIRECTION ( 'NONE',  ( 0.000000000000000000, -1.000000000000000000, 0.000000000000000000 ) ) ;
#10846=ORIENTED_EDGE ( 'NONE', *, *, #31465, .F. ) ;
#10856=FACE_OUTER_BOUND ( 'NONE', #9284, .T. ) ;
#10857=EDGE_CURVE ( 'NONE', #8335, #253, #532, .T. ) ;
#10862=CARTESIAN_POINT ( 'NONE',  ( -38.22595157131660670, -5.901281111979422178, 78.33466235588149118 ) ) ;
#10871=CARTESIAN_POINT ( 'NONE',  ( -63.90214402394282445, 9.925589859889722533, 42.04930799450051637 ) ) ;
#10872=ADVANCED_FACE ( 'NONE', ( #610 ), #3145, .T. ) ;
#10878=ORIENTED_EDGE ( 'NONE', *, *, #25498, .F. ) ;
#10882=CARTESIAN_POINT ( 'NONE',  ( -39.41803741763551017, -5.935648345809891424, 77.97613421639424303 ) ) ;
#10898=CARTESIAN_POINT ( 'NONE',  ( -2.055626032295933214, 11.55977609614115842, -4.009591101970203297 ) ) ;
#10903=CIRCLE ( 'NONE', #5145, 2.500000000000002220 ) ;
#10907=CARTESIAN_POINT ( 'NONE',  ( 78.06792761052983565, -4.708525186292313869, 80.13239438898611411 ) ) ;
#10911=DIRECTION ( 'NONE',  ( 0.000000000000000000, -1.000000000000000000, 0.000000000000000000 ) ) ;
#10915=B_SPLINE_CURVE_WITH_KNOTS ( 'NONE', 3,
 ( #30941, #10765, #18602, #28630, #3356, #23223, #13703, #739, #21224, #3188, #6142, #16143, #26161, #18282, #8760, #8452, #15669, #20756, #18130, #5836, #13387, #15839, #23704, #5509, #25841, #15514, #23054, #1208, #3027, #5990 ),
 .UNSPECIFIED., .F., .F.,
 ( 4, 2, 2, 2, 2, 2, 2, 2, 2, 2, 2, 2, 2, 2, 4 ),
 ( 0.000000000000000000, 0.001249755272498786519, 0.002499510544997573039, 0.003749265817496359558, 0.004999021089995146078, 0.007498531634992704371, 0.009998042179990264400, 0.01249755272498782183, 0.01374730799748660401, 0.01499706326998538446, 0.01562194090623477902, 0.01624681854248417184, 0.01749657381498295750, 0.01874632908748173968, 0.01999608435998052533 ),
 .UNSPECIFIED. ) ;
#10925=CIRCLE ( 'NONE', #4090, 66.44011198581388555 ) ;
#10932=CARTESIAN_POINT ( 'NONE',  ( -35.64882101543633297, 9.925589859889722533, 42.04930799450051637 ) ) ;
#10935=CARTESIAN_POINT ( 'NONE',  ( -34.31970563170440158, 11.92558985988973497, 54.04930799450052348 ) ) ;
#10957=CARTESIAN_POINT ( 'NONE',  ( 81.63177831856063449, -5.935454207752202116, 16.07118271501079576 ) ) ;
#10959=AXIS2_PLACEMENT_3D ( 'NONE', #487, #28073, #30214 ) ;
#10962=ORIENTED_EDGE ( 'NONE', *, *, #16376, .T. ) ;
#10964=CARTESIAN_POINT ( 'NONE',  ( -5.602943079677954685, 9.702389020015065313, 98.41455612196619995 ) ) ;
#10966=ORIENTED_EDGE ( 'NONE', *, *, #19284, .T. ) ;
#10970=EDGE_CURVE ( 'NONE', #18754, #30781, #21998, .T. ) ;
#10977=EDGE_LOOP ( 'NONE', ( #27871, #12803 ) ) ;
#10982=CARTESIAN_POINT ( 'NONE',  ( 54.73929935417030634, -1.580002914024320360, 101.6640897793760558 ) ) ;
#10986=CARTESIAN_POINT ( 'NONE',  ( -4.668528339753533984, 10.39233698702945752, -4.365831785235375406 ) ) ;
#10992=CARTESIAN_POINT ( 'NONE',  ( 21.09785597605719332, 25.56454579224779877, 73.04930799450052348 ) ) ;
#10999=CIRCLE ( 'NONE', #1535, 54.29999999999999716 ) ;
#11002=ADVANCED_FACE ( 'NONE', ( #16177 ), #19921, .F. ) ;
#11003=AXIS2_PLACEMENT_3D ( 'NONE', #15948, #20385, #3311 ) ;
#11006=ORIENTED_EDGE ( 'NONE', *, *, #6044, .F. ) ;
#11018=FACE_OUTER_BOUND ( 'NONE', #23719, .T. ) ;
#11044=CARTESIAN_POINT ( 'NONE',  ( -39.51039602574057596, -5.935454207752198563, 77.87546120947918382 ) ) ;
#11046=EDGE_CURVE ( 'NONE', #19298, #3553, #3162, .T. ) ;
#11053=EDGE_LOOP ( 'NONE', ( #22104, #25516 ) ) ;
#11061=ORIENTED_EDGE ( 'NONE', *, *, #14950, .T. ) ;
#11064=DIRECTION ( 'NONE',  ( 0.000000000000000000, 0.000000000000000000, -1.000000000000000000 ) ) ;
#11073=CARTESIAN_POINT ( 'NONE',  ( 77.52599780128986140, -4.161241697801461470, 80.45688245215025347 ) ) ;
#11082=CARTESIAN_POINT ( 'NONE',  ( 21.09785597605719332, 24.56454579224780232, 86.74871914086746472 ) ) ;
#11083=ORIENTED_EDGE ( 'NONE', *, *, #8305, .F. ) ;
#11084=CARTESIAN_POINT ( 'NONE',  ( 72.66245921547933051, 10.95084857405595535, 22.29041010318592697 ) ) ;
#11092=ORIENTED_EDGE ( 'NONE', *, *, #16249, .F. ) ;
#11100=CARTESIAN_POINT ( 'NONE',  ( 21.09785597605720042, 12.78350261226561280, 102.7736706386835408 ) ) ;
#11104=DIRECTION ( 'NONE',  ( -0.000000000000000000, -1.000000000000000000, -0.000000000000000000 ) ) ;
#11111=ORIENTED_EDGE ( 'NONE', *, *, #31947, .F. ) ;
#11114=DIRECTION ( 'NONE',  ( 0.000000000000000000, 0.000000000000000000, -1.000000000000000000 ) ) ;
#11128=ORIENTED_EDGE ( 'NONE', *, *, #2631, .F. ) ;
#11129=CIRCLE ( 'NONE', #23696, 1.700000000000007061 ) ;
#11130=EDGE_CURVE ( 'NONE', #8185, #11449, #27281, .T. ) ;
#11133=EDGE_LOOP ( 'NONE', ( #25821, #18214, #26039, #17630 ) ) ;
#11134=CARTESIAN_POINT ( 'NONE',  ( 80.77181806311268986, -3.295808585244882849, 11.79002343214943238 ) ) ;
#11135=AXIS2_PLACEMENT_3D ( 'NONE', #17476, #2388, #27496 ) ;
#11140=DIRECTION ( 'NONE',  ( -0.000000000000000000, 1.000000000000000000, -0.000000000000000000 ) ) ;
#11142=ORIENTED_EDGE ( 'NONE', *, *, #4254, .T. ) ;
#11149=DIRECTION ( 'NONE',  ( 0.000000000000000000, -1.000000000000000000, 0.000000000000000000 ) ) ;
#11150=CARTESIAN_POINT ( 'NONE',  ( -5.602943079677954685, 9.702389020015065313, -4.315940132965163656 ) ) ;
#11171=DIRECTION ( 'NONE',  ( -0.000000000000000000, -1.000000000000000000, -0.000000000000000000 ) ) ;
#11180=DIRECTION ( 'NONE',  ( 0.000000000000000000, 0.000000000000000000, 1.000000000000000000 ) ) ;
#11211=CARTESIAN_POINT ( 'NONE',  ( 71.63986567979446818, 8.190330151142699577, 18.74290927009450058 ) ) ;
#11226=VERTEX_POINT ( 'NONE', #13831 ) ;
#11234=ADVANCED_FACE ( 'NONE', ( #23676 ), #24149, .F. ) ;
#11237=CARTESIAN_POINT ( 'NONE',  ( 21.09785597605719332, -15.93545420775219945, 47.04930799450051637 ) ) ;
#11244=CIRCLE ( 'NONE', #4422, 85.00000000000001421 ) ;
#11258=CARTESIAN_POINT ( 'NONE',  ( -5.144846497709795408, 10.07270486929682107, 97.52097793833394235 ) ) ;
#11259=ORIENTED_EDGE ( 'NONE', *, *, #13950, .F. ) ;
#11262=PLANE ( 'NONE',  #1305 ) ;
#11271=CARTESIAN_POINT ( 'NONE',  ( 71.55936645880203173, 9.702389020015065313, 20.34850893876554423 ) ) ;
#11278=CONICAL_SURFACE ( 'NONE', #29616, 72.49999999999997158, 0.7853981633974482790 ) ;
#11284=ORIENTED_EDGE ( 'NONE', *, *, #22238, .T. ) ;
#11285=ORIENTED_EDGE ( 'NONE', *, *, #26756, .T. ) ;
#11286=DIRECTION ( 'NONE',  ( 0.000000000000000000, 0.000000000000000000, -1.000000000000000000 ) ) ;
#11289=AXIS2_PLACEMENT_3D ( 'NONE', #15087, #25099, #4578 ) ;
#11299=VERTEX_POINT ( 'NONE', #24564 ) ;
#11307=ORIENTED_EDGE ( 'NONE', *, *, #7272, .T. ) ;
#11313=CARTESIAN_POINT ( 'NONE',  ( 21.09785597605719332, 24.56454579224780232, 86.74871914086746472 ) ) ;
#11317=DIRECTION ( 'NONE',  ( -0.000000000000000000, 1.000000000000000000, -0.000000000000000000 ) ) ;
#11321=ORIENTED_EDGE ( 'NONE', *, *, #7381, .F. ) ;
#11341=CARTESIAN_POINT ( 'NONE',  ( -38.21956372845817640, 5.305745712741808617, 52.04930799450051637 ) ) ;
#11344=EDGE_CURVE ( 'NONE', #6305, #3624, #19962, .T. ) ;
#11357=DIRECTION ( 'NONE',  ( 0.000000000000000000, 0.000000000000000000, 1.000000000000000000 ) ) ;
#11360=CARTESIAN_POINT ( 'NONE',  ( -63.90214402394282445, 9.925589859889734967, 54.04930799450052348 ) ) ;
#11366=FACE_BOUND ( 'NONE', #9871, .T. ) ;
#11368=DIRECTION ( 'NONE',  ( -0.000000000000000000, 1.000000000000000000, -0.000000000000000000 ) ) ;
#11382=CARTESIAN_POINT ( 'NONE',  ( -44.78514533282907450, -5.110533499441238803, 41.67803216526434795 ) ) ;
#11383=DIRECTION ( 'NONE',  ( 0.000000000000000000, -1.000000000000000000, 0.000000000000000000 ) ) ;
#11386=EDGE_CURVE ( 'NONE', #23463, #2467, #12432, .T. ) ;
#11389=CARTESIAN_POINT ( 'NONE',  ( 51.66808379569695830, 5.388785998227650254, 97.45038561958638468 ) ) ;
#11405=CARTESIAN_POINT ( 'NONE',  ( 21.09785597605719332, 13.74476430820393347, 102.0493079945005093 ) ) ;
#11411=DIRECTION ( 'NONE',  ( 1.000000000000000000, 0.000000000000000000, 2.775557561562888984E-15 ) ) ;
#11417=CARTESIAN_POINT ( 'NONE',  ( 21.09785597605719332, 12.74140866975414887, 47.04930799450051637 ) ) ;
#11418=CARTESIAN_POINT ( 'NONE',  ( 21.09785597605719332, -6.659195188345857552, 47.04930799450051637 ) ) ;
#11426=ORIENTED_EDGE ( 'NONE', *, *, #337, .T. ) ;
#11438=ORIENTED_EDGE ( 'NONE', *, *, #31546, .T. ) ;
#11447=CARTESIAN_POINT ( 'NONE',  ( -12.16553382968505481, -0.1676091211930501867, -5.936183209767050606 ) ) ;
#11449=VERTEX_POINT ( 'NONE', #18470 ) ;
#11477=ORIENTED_EDGE ( 'NONE', *, *, #22194, .T. ) ;
#11487=CARTESIAN_POINT ( 'NONE',  ( 73.38268324366261197, 4.638969541771025717, 16.21882525954990228 ) ) ;
#11491=FACE_BOUND ( 'NONE', #7155, .T. ) ;
#11503=CARTESIAN_POINT ( 'NONE',  ( -12.61173037625193061, -3.171899563477257100, -8.558298061174587801 ) ) ;
#11512=CIRCLE ( 'NONE', #8378, 54.49999999999997868 ) ;
#11521=ORIENTED_EDGE ( 'NONE', *, *, #23468, .T. ) ;
#11557=ORIENTED_EDGE ( 'NONE', *, *, #2306, .F. ) ;
#11560=VERTEX_POINT ( 'NONE', #25381 ) ;
#11570=CARTESIAN_POINT ( 'NONE',  ( 81.63175399755476747, -5.935454207809698346, 78.02743327247107175 ) ) ;
#11584=DIRECTION ( 'NONE',  ( 0.000000000000000000, 1.000000000000000000, 0.000000000000000000 ) ) ;
#11587=DIRECTION ( 'NONE',  ( -0.000000000000000000, -1.000000000000000000, -0.000000000000000000 ) ) ;
#11590=TOROIDAL_SURFACE ( 'NONE', #3191, 56.00000000000000000, 1.700000000000000178 ) ;
#11595=CARTESIAN_POINT ( 'NONE',  ( -44.25477285282614304, -5.710200047292144809, 40.98160301053449928 ) ) ;
#11596=AXIS2_PLACEMENT_3D ( 'NONE', #2543, #27162, #24874 ) ;
#11598=ORIENTED_EDGE ( 'NONE', *, *, #13898, .F. ) ;
#11612=CARTESIAN_POINT ( 'NONE',  ( 47.09785597605719687, 25.56454579224779877, 47.04930799450042400 ) ) ;
#11617=ORIENTED_EDGE ( 'NONE', *, *, #32257, .T. ) ;
#11621=CARTESIAN_POINT ( 'NONE',  ( -36.45222641229887017, 9.925589859889722533, 42.04930799450051637 ) ) ;
#11622=DIRECTION ( 'NONE',  ( -1.000000000000000000, 0.000000000000000000, 0.000000000000000000 ) ) ;
#11624=CYLINDRICAL_SURFACE ( 'NONE', #1105, 10.00000000000000178 ) ;
#11628=DIRECTION ( 'NONE',  ( 3.534951791954965799E-15, 3.759183808608825436E-15, -1.000000000000000000 ) ) ;
#11635=AXIS2_PLACEMENT_3D ( 'NONE', #30203, #14941, #17712 ) ;
#11641=ADVANCED_BREP_SHAPE_REPRESENTATION ( '', ( #1464, #8172 ), #19670 ) ;
#11653=EDGE_CURVE ( 'NONE', #16169, #13013, #3697, .T. ) ;
#11660=CARTESIAN_POINT ( 'NONE',  ( 74.77803812839373165, 0.4256545730734913047, 14.01035497445585243 ) ) ;
#11664=PLANE ( 'NONE',  #5515 ) ;
#11673=EDGE_CURVE ( 'NONE', #3218, #3824, #5312, .T. ) ;
#11676=VERTEX_POINT ( 'NONE', #23722 ) ;
#11677=DIRECTION ( 'NONE',  ( 0.000000000000000000, -0.000000000000000000, 1.000000000000000000 ) ) ;
#11679=AXIS2_PLACEMENT_3D ( 'NONE', #17053, #2127, #27067 ) ;
#11680=ORIENTED_EDGE ( 'NONE', *, *, #19172, .T. ) ;
#11698=CARTESIAN_POINT ( 'NONE',  ( 54.83501011029174066, -2.946992577399113244, -7.456648316814940003 ) ) ;
#11704=CIRCLE ( 'NONE', #17462, 2.500000000000002220 ) ;
#11710=CARTESIAN_POINT ( 'NONE',  ( 21.09785597605720042, 11.78014697381582643, -8.546216316978195948 ) ) ;
#11713=CARTESIAN_POINT ( 'NONE',  ( 52.07598125554711999, -5.935454207752202116, 106.6682925056943958 ) ) ;
#11722=CARTESIAN_POINT ( 'NONE',  ( 73.84527214715876653, 11.92558985988973497, 26.36226255498455728 ) ) ;
#11733=CARTESIAN_POINT ( 'NONE',  ( 81.73634015752263338, -5.935454207752201228, 77.87546120947916961 ) ) ;
#11739=CARTESIAN_POINT ( 'NONE',  ( 73.09176707068564838, 11.92558985988973497, 67.46350265493038023 ) ) ;
#11758=ORIENTED_EDGE ( 'NONE', *, *, #20966, .T. ) ;
#11759=ADVANCED_FACE ( 'NONE', ( #22224 ), #17366, .F. ) ;
#11762=ORIENTED_EDGE ( 'NONE', *, *, #13503, .T. ) ;
#11765=VECTOR ( 'NONE', #25465, 1000.000000000000000 ) ;
#11776=EDGE_CURVE ( 'NONE', #11676, #8185, #8977, .T. ) ;
#11787=FACE_BOUND ( 'NONE', #30958, .T. ) ;
#11793=VERTEX_POINT ( 'NONE', #25188 ) ;
#11808=EDGE_LOOP ( 'NONE', ( #12340, #15765 ) ) ;
#11811=EDGE_CURVE ( 'NONE', #4643, #12963, #29467, .T. ) ;
#11814=CARTESIAN_POINT ( 'NONE',  ( 51.92400919103565116, -5.935454207752203004, -13.53511453669547215 ) ) ;
#11823=CARTESIAN_POINT ( 'NONE',  ( 72.70365453605475636, 7.326690775934352473, 18.02522573148189977 ) ) ;
#11829=FACE_OUTER_BOUND ( 'NONE', #10977, .T. ) ;
#11838=CARTESIAN_POINT ( 'NONE',  ( -12.08400064424376730, 0.05876815387848967343, -6.781675208179526848 ) ) ;
#11844=VECTOR ( 'NONE', #28300, 1000.000000000000000 ) ;
#11846=DIRECTION ( 'NONE',  ( 1.000000000000000000, -0.000000000000000000, -0.000000000000000000 ) ) ;
#11855=DIRECTION ( 'NONE',  ( -0.000000000000000000, 1.000000000000000000, -0.000000000000000000 ) ) ;
#11861=EDGE_CURVE ( 'NONE', #1224, #9654, #17447, .T. ) ;
#11893=EDGE_CURVE ( 'NONE', #20681, #2165, #28774, .T. ) ;
#11894=ORIENTED_EDGE ( 'NONE', *, *, #32219, .T. ) ;
#11896=ORIENTED_EDGE ( 'NONE', *, *, #31220, .F. ) ;
#11899=CARTESIAN_POINT ( 'NONE',  ( 71.56952591989053758, 10.07270486929681930, 73.29201046826767652 ) ) ;
#11921=CONICAL_SURFACE ( 'NONE', #9832, 39.63553620740810857, 0.6632251157578421541 ) ;
#11929=CARTESIAN_POINT ( 'NONE',  ( -39.45773241730296377, -5.935454212835550969, 77.98461610899785512 ) ) ;
#11936=CARTESIAN_POINT ( 'NONE',  ( -5.950449876020693196, 9.421471677506305653, 97.50311162695551559 ) ) ;
#11939=CARTESIAN_POINT ( 'NONE',  ( -12.52393922272763227, -3.543532154952163893, -7.915647480175222128 ) ) ;
#11940=ORIENTED_EDGE ( 'NONE', *, *, #31947, .T. ) ;
#11943=DIRECTION ( 'NONE',  ( 0.000000000000000000, 0.000000000000000000, -1.000000000000000000 ) ) ;
#11956=CARTESIAN_POINT ( 'NONE',  ( -38.57628410747783221, 11.92829594627139933, 24.97746215641624090 ) ) ;
#11957=AXIS2_PLACEMENT_3D ( 'NONE', #23528, #25830, #13375 ) ;
#11962=CARTESIAN_POINT ( 'NONE',  ( 21.09785597605719332, 11.78014697381582643, 47.04930799450051637 ) ) ;
#12016=CARTESIAN_POINT ( 'NONE',  ( 53.16699371189685053, -5.614579432636292111, -10.15581503676737185 ) ) ;
#12022=CARTESIAN_POINT ( 'NONE',  ( 47.09785597605719687, 25.56454579224779877, 49.54930799450042400 ) ) ;
#12029=VECTOR ( 'NONE', #9585, 1000.000000000000000 ) ;
#12030=CARTESIAN_POINT ( 'NONE',  ( 54.14309329449467612, -4.768257113790710378, 103.1530495731739592 ) ) ;
#12037=ORIENTED_EDGE ( 'NONE', *, *, #20850, .F. ) ;
#12041=FACE_OUTER_BOUND ( 'NONE', #9601, .T. ) ;
#12045=CARTESIAN_POINT ( 'NONE',  ( 72.58709125692084285, 11.83483724345210142, 25.26238199259950079 ) ) ;
#12052=ADVANCED_FACE ( 'NONE', ( #21049 ), #3658, .F. ) ;
#12057=CARTESIAN_POINT ( 'NONE',  ( -30.88776582636845092, 11.92558985988972786, 67.48460561594581009 ) ) ;
#12058=CARTESIAN_POINT ( 'NONE',  ( -29.85004370764308490, 6.158867040949189686, 76.91207085872912330 ) ) ;
#12059=CARTESIAN_POINT ( 'NONE',  ( -29.27613032885505007, 11.92829597396328012, 69.12115383893792853 ) ) ;
#12064=CARTESIAN_POINT ( 'NONE',  ( 51.97542764375435809, -5.937448199248382075, -13.65255231306078798 ) ) ;
#12080=DIRECTION ( 'NONE',  ( 0.000000000000000000, 0.000000000000000000, -1.000000000000000000 ) ) ;
#12094=EDGE_CURVE ( 'NONE', #18864, #26491, #1135, .T. ) ;
#12112=CARTESIAN_POINT ( 'NONE',  ( -11.17519415121370763, 2.112486173643649767, -5.064473702997324800 ) ) ;
#12117=CARTESIAN_POINT ( 'NONE',  ( 52.13943755312613604, -5.936969727347465309, 107.6745679524140229 ) ) ;
#12118=CARTESIAN_POINT ( 'NONE',  ( 47.09785597605719687, 24.86454579224779948, 44.54930799450042400 ) ) ;
#12123=EDGE_LOOP ( 'NONE', ( #21594, #2381 ) ) ;
#12127=CARTESIAN_POINT ( 'NONE',  ( 100.3079064823960493, -16.63545420775219696, 47.04930799450134771 ) ) ;
#12130=VERTEX_POINT ( 'NONE', #29425 ) ;
#12141=CARTESIAN_POINT ( 'NONE',  ( 51.94765923753424630, -5.936248947737084336, -13.45830144247714344 ) ) ;
#12155=TOROIDAL_SURFACE ( 'NONE', #18941, 48.97546517713167447, 2.000000000000000000 ) ;
#12167=DIRECTION ( 'NONE',  ( 0.000000000000000000, 1.000000000000000000, 0.000000000000000000 ) ) ;
#12172=EDGE_CURVE ( 'NONE', #26169, #26256, #32218, .T. ) ;
#12174=AXIS2_PLACEMENT_3D ( 'NONE', #10333, #4921, #17550 ) ;
#12178=ORIENTED_EDGE ( 'NONE', *, *, #3336, .T. ) ;
#12181=ORIENTED_EDGE ( 'NONE', *, *, #15677, .F. ) ;
#12184=DIRECTION ( 'NONE',  ( 0.000000000000000000, 0.000000000000000000, -1.000000000000000000 ) ) ;
#12189=CARTESIAN_POINT ( 'NONE',  ( 0.6836613156275053171, 11.92558985988973497, -5.803495753465989893 ) ) ;
#12192=DIRECTION ( 'NONE',  ( 0.000000000000000000, 0.000000000000000000, -1.000000000000000000 ) ) ;
#12194=VERTEX_POINT ( 'NONE', #21857 ) ;
#12205=CARTESIAN_POINT ( 'NONE',  ( -39.52299075669071016, -5.935454207752198563, 77.87546120947918382 ) ) ;
#12209=LINE ( 'NONE', #32233, #6313 ) ;
#12219=CIRCLE ( 'NONE', #17458, 55.87116166729571631 ) ;
#12227=ADVANCED_FACE ( 'NONE', ( #20861 ), #6838, .F. ) ;
#12230=ORIENTED_EDGE ( 'NONE', *, *, #15620, .T. ) ;
#12232=DIRECTION ( 'NONE',  ( 0.000000000000000000, 0.000000000000000000, 1.000000000000000000 ) ) ;
#12233=DIRECTION ( 'NONE',  ( 0.000000000000000000, 1.000000000000000000, 0.000000000000000000 ) ) ;
#12246=CARTESIAN_POINT ( 'NONE',  ( 21.09785597605719332, 24.86454579224780304, 47.04930799450051637 ) ) ;
#12259=CIRCLE ( 'NONE', #3860, 47.05803085792211249 ) ;
#12260=EDGE_CURVE ( 'NONE', #26491, #18864, #15763, .T. ) ;
#12265=CARTESIAN_POINT ( 'NONE',  ( 78.48781352222600560, -5.738638231773887100, 15.17031821407819514 ) ) ;
#12271=CARTESIAN_POINT ( 'NONE',  ( -8.808741845175550367, 6.094407115496628613, 98.01272063432647030 ) ) ;
#12273=CARTESIAN_POINT ( 'NONE',  ( -30.40389907987879070, 7.914959306551518026, 18.50712902613415167 ) ) ;
#12279=CARTESIAN_POINT ( 'NONE',  ( 52.10136161249906195, -5.936382080411357620, 107.6680807723975164 ) ) ;
#12280=DIRECTION ( 'NONE',  ( -0.000000000000000000, -0.000000000000000000, 1.000000000000000000 ) ) ;
#12308=VERTEX_POINT ( 'NONE', #23169 ) ;
#12322=ORIENTED_EDGE ( 'NONE', *, *, #14053, .F. ) ;
#12328=EDGE_LOOP ( 'NONE', ( #26659, #16354, #19937, #23781 ) ) ;
#12340=ORIENTED_EDGE ( 'NONE', *, *, #1291, .T. ) ;
#12343=CARTESIAN_POINT ( 'NONE',  ( 72.77125109260951774, 11.18949478403749787, 71.27148623857269172 ) ) ;
#12348=CARTESIAN_POINT ( 'NONE',  ( 51.47386758732231016, 5.370505999354205251, -4.102960719301439241 ) ) ;
#12369=VECTOR ( 'NONE', #28605, 1000.000000000000000 ) ;
#12370=CARTESIAN_POINT ( 'NONE',  ( 52.27789684966019479, -5.944439029104267469, 104.9516812706435758 ) ) ;
#12385=DIRECTION ( 'NONE',  ( 0.000000000000000000, 3.756723415560144304E-15, -1.000000000000000000 ) ) ;
#12397=DIRECTION ( 'NONE',  ( 1.000000000000000000, 0.000000000000000000, 1.224646799147353207E-16 ) ) ;
#12403=CARTESIAN_POINT ( 'NONE',  ( 74.89817579486182808, -1.820484904611762156, 80.73796779739511464 ) ) ;
#12405=CARTESIAN_POINT ( 'NONE',  ( -31.75494777190936802, 11.92558985988973674, 26.63511333407100778 ) ) ;
#12425=B_SPLINE_CURVE_WITH_KNOTS ( 'NONE', 3,
 ( #2426, #30804, #2903, #279, #8317, #17838, #3383, #18154, #13416, #18314, #3224, #5869 ),
 .UNSPECIFIED., .F., .F.,
 ( 4, 2, 2, 2, 2, 4 ),
 ( 0.0001999864807696098657, 0.001053893586900949038, 0.001480847139966614233, 0.001907800693032279428, 0.002761707799163610252, 0.003615614905294941075 ),
 .UNSPECIFIED. ) ;
#12432=LINE ( 'NONE', #2569, #28357 ) ;
#12435=CARTESIAN_POINT ( 'NONE',  ( -10.97128175978245324, -5.614579432636300993, 104.2544310257684117 ) ) ;
#12437=CARTESIAN_POINT ( 'NONE',  ( -37.21204910874187988, -5.721341737285086992, 15.20211895544695757 ) ) ;
#12444=DIRECTION ( 'NONE',  ( -0.000000000000000000, -0.000000000000000000, 1.000000000000000000 ) ) ;
#12448=DIRECTION ( 'NONE',  ( -0.000000000000000000, 1.000000000000000000, -0.000000000000000000 ) ) ;
#12456=EDGE_CURVE ( 'NONE', #21280, #2467, #10003, .T. ) ;
#12457=ORIENTED_EDGE ( 'NONE', *, *, #27637, .T. ) ;
#12461=B_SPLINE_CURVE_WITH_KNOTS ( 'NONE', 3,
 ( #4035, #22074, #19117, #21586 ),
 .UNSPECIFIED., .F., .F.,
 ( 4, 4 ),
 ( 0.000000000000000000, 1.000000000000000000 ),
 .UNSPECIFIED. ) ;
#12468=CARTESIAN_POINT ( 'NONE',  ( 79.40776106085759523, -5.721341737285999152, 78.89649703355206611 ) ) ;
#12480=DIRECTION ( 'NONE',  ( 0.000000000000000000, 0.000000000000000000, 1.000000000000000000 ) ) ;
#12484=CARTESIAN_POINT ( 'NONE',  ( 52.06562842487888787, -5.940946157296536967, -12.59682317512997685 ) ) ;
#12487=VERTEX_POINT ( 'NONE', #1563 ) ;
#12498=CARTESIAN_POINT ( 'NONE',  ( 21.09785597605719332, 16.86454579224779948, 47.04930799450051637 ) ) ;
#12504=ADVANCED_FACE ( 'NONE', ( #4850 ), #24160, .F. ) ;
#12522=FACE_OUTER_BOUND ( 'NONE', #23286, .T. ) ;
#12529=CARTESIAN_POINT ( 'NONE',  ( -31.47697969167641219, 0.8211122444364866713, 14.16255949990320318 ) ) ;
#12530=VECTOR ( 'NONE', #22653, 1000.000000000000000 ) ;
#12532=EDGE_LOOP ( 'NONE', ( #28377, #22189, #20689, #7851 ) ) ;
#12535=DIRECTION ( 'NONE',  ( 0.000000000000000000, 0.000000000000000000, -1.000000000000000000 ) ) ;
#12542=FACE_OUTER_BOUND ( 'NONE', #7134, .T. ) ;
#12560=CARTESIAN_POINT ( 'NONE',  ( 21.09785597605719332, 25.56454579224780232, 123.7593585008393831 ) ) ;
#12564=CARTESIAN_POINT ( 'NONE',  ( -9.883496200693420164, -5.935668478901861000, -13.53764849166516271 ) ) ;
#12567=CARTESIAN_POINT ( 'NONE',  ( 72.46539012849335393, 9.161285963347369332, 74.39120288609333898 ) ) ;
#12575=VECTOR ( 'NONE', #20263, 1000.000000000000000 ) ;
#12578=DIRECTION ( 'NONE',  ( 0.000000000000000000, 0.000000000000000000, 1.000000000000000000 ) ) ;
#12579=ORIENTED_EDGE ( 'NONE', *, *, #19632, .F. ) ;
#12583=B_SPLINE_CURVE_WITH_KNOTS ( 'NONE', 3,
 ( #27108, #14487, #9389, #2169, #4305, #16929, #22179, #26947, #14322, #12348, #32206, #9723, #19716, #24159, #22342, #9879, #19878, #29418, #29912, #26620, #9231, #1675, #11698, #21690, #24479, #19220, #6926, #1999, #32043, #29245, #12016, #22009, #10706, #13161, #2812, #10051 ),
 .UNSPECIFIED., .F., .F.,
 ( 4, 2, 2, 2, 2, 2, 2, 2, 2, 2, 2, 2, 2, 2, 2, 2, 2, 4 ),
 ( 0.000000000000000000, 0.001327013081135470672, 0.002654026162270941343, 0.003981039243406411798, 0.005308052324541882687, 0.006635065405677354443, 0.007962078486812823597, 0.01061610464908375670, 0.01194311773021922325, 0.01327013081135468633, 0.01459714389249015289, 0.01592415697362561944, 0.01725117005476108772, 0.01857818313589655254, 0.01924168967646429015, 0.01990519621703202777, 0.02056870275759976538, 0.02123220929816750299 ),
 .UNSPECIFIED. ) ;
#12584=ADVANCED_FACE ( 'NONE', ( #2708 ), #4256, .T. ) ;
#12588=EDGE_CURVE ( 'NONE', #20217, #7822, #19754, .T. ) ;
#12590=CARTESIAN_POINT ( 'NONE',  ( -9.880269301913145341, -5.935454207809699234, 107.5832060159989965 ) ) ;
#12595=CARTESIAN_POINT ( 'NONE',  ( 73.21163767355515972, 2.112486173643641774, 14.77625786722979839 ) ) ;
#12600=CARTESIAN_POINT ( 'NONE',  ( -11.74161162749063081, 0.8961463385898310596, 99.60459568951398523 ) ) ;
#12602=CARTESIAN_POINT ( 'NONE',  ( -30.25345129064801242, 9.506884710854171416, 20.08466430870300101 ) ) ;
#12618=CARTESIAN_POINT ( 'NONE',  ( -41.59221410450253842, 0.6853199587562655015, 52.04930799450050927 ) ) ;
#12620=EDGE_LOOP ( 'NONE', ( #5254, #31849, #3100, #25226, #24234, #2151 ) ) ;
#12623=EDGE_LOOP ( 'NONE', ( #24069, #6878, #4717, #14691, #27054, #11894, #2240, #25693 ) ) ;
#12638=DIRECTION ( 'NONE',  ( 1.000000000000000000, 0.000000000000000000, 0.000000000000000000 ) ) ;
#12648=CARTESIAN_POINT ( 'NONE',  ( 21.09785597605807439, -5.935454207752083988, 47.04930799450051637 ) ) ;
#12657=EDGE_CURVE ( 'NONE', #22918, #1340, #22596, .T. ) ;
#12668=CARTESIAN_POINT ( 'NONE',  ( 21.09785597605720042, -6.659195188345857552, 114.2205349567709476 ) ) ;
#12674=CARTESIAN_POINT ( 'NONE',  ( -37.69242682074983719, -5.812585053298397142, 15.41977583216693226 ) ) ;
#12679=CARTESIAN_POINT ( 'NONE',  ( -38.65545646816406133, 8.768497436727981764, 75.00977582921336762 ) ) ;
#12682=DIRECTION ( 'NONE',  ( 0.000000000000000000, -1.000000000000000000, 0.000000000000000000 ) ) ;
#12696=ORIENTED_EDGE ( 'NONE', *, *, #5406, .T. ) ;
#12700=EDGE_CURVE ( 'NONE', #27012, #8335, #28949, .T. ) ;
#12703=CARTESIAN_POINT ( 'NONE',  ( 71.48501281440437083, 5.388785998227653806, 77.62194537253989779 ) ) ;
#12716=VECTOR ( 'NONE', #4153, 1000.000000000000000 ) ;
#12725=ORIENTED_EDGE ( 'NONE', *, *, #4262, .T. ) ;
#12726=CARTESIAN_POINT ( 'NONE',  ( 21.09785597605720042, 13.06454579224779877, -7.250692005499486115 ) ) ;
#12733=CARTESIAN_POINT ( 'NONE',  ( 79.08111791895156273, -5.943281723642246384, 78.07730698287811322 ) ) ;
#12741=EDGE_LOOP ( 'NONE', ( #19665, #25519, #29067, #17368, #11557, #30242, #16098, #20246, #21812, #15264, #28703, #25499, #6368, #17562, #10779, #4550 ) ) ;
#12743=CARTESIAN_POINT ( 'NONE',  ( 0.6836613156275018754, 11.92558985988973497, 99.04321908912905315 ) ) ;
#12744=ORIENTED_EDGE ( 'NONE', *, *, #19664, .F. ) ;
#12745=CYLINDRICAL_SURFACE ( 'NONE', #28806, 2.500000000000002220 ) ;
#12750=B_SPLINE_SURFACE_WITH_KNOTS ( 'NONE', 3, 1, ( 
 ( #14524, #2043 ),
 ( #12064, #29134 ),
 ( #9600, #28970 ),
 ( #26661, #16489 ) ),
 .UNSPECIFIED., .F., .F., .F.,
 ( 4, 4 ),
 ( 2, 2 ),
 ( 0.1800733115436725096, 0.1889470565094409915 ),
 ( 0.000000000000000000, 1.000000000000000000 ),
 .UNSPECIFIED. ) ;
#12756=CARTESIAN_POINT ( 'NONE',  ( -9.880269303432738681, -5.935454207752202116, -37.95069200549950494 ) ) ;
#12757=DIRECTION ( 'NONE',  ( 0.000000000000000000, 0.000000000000000000, -1.000000000000000000 ) ) ;
#12758=VERTEX_POINT ( 'NONE', #16300 ) ;
#12760=VECTOR ( 'NONE', #29019, 1000.000000000000000 ) ;
#12761=CARTESIAN_POINT ( 'NONE',  ( 21.09785597605719332, 14.86454579224779948, -7.160742511838298796 ) ) ;
#12763=CARTESIAN_POINT ( 'NONE',  ( -30.25373303598937369, 9.514306310867874927, 74.00447224759949449 ) ) ;
#12769=CARTESIAN_POINT ( 'NONE',  ( -36.31984027485262345, -5.100301982865893535, 14.30915805386189454 ) ) ;
#12793=AXIS2_PLACEMENT_3D ( 'NONE', #15871, #25552, #23257 ) ;
#12795=VECTOR ( 'NONE', #15478, 1000.000000000000000 ) ;
#12803=ORIENTED_EDGE ( 'NONE', *, *, #7398, .T. ) ;
#12807=CARTESIAN_POINT ( 'NONE',  ( 42.88580625581234074, 11.83469976691315928, 99.40613855222599682 ) ) ;
#12808=CARTESIAN_POINT ( 'NONE',  ( 54.84005179923816797, -2.833757427854255884, 102.4175021926326536 ) ) ;
#12826=EDGE_CURVE ( 'NONE', #20059, #9364, #3721, .T. ) ;
#12828=CIRCLE ( 'NONE', #15434, 55.85791022362053582 ) ;
#12830=EDGE_LOOP ( 'NONE', ( #29412, #8024 ) ) ;
#12833=CARTESIAN_POINT ( 'NONE',  ( -44.25806916964057791, -4.109955628810420869, 52.04930799449938661 ) ) ;
#12846=DIRECTION ( 'NONE',  ( 0.000000000000000000, 1.000000000000000000, 0.000000000000000000 ) ) ;
#12852=CARTESIAN_POINT ( 'NONE',  ( 21.09785597605719332, 25.18020726757345429, 47.04930799450051637 ) ) ;
#12853=DIRECTION ( 'NONE',  ( 0.000000000000000000, -0.7071067811865474617, -0.7071067811865474617 ) ) ;
#12854=CARTESIAN_POINT ( 'NONE',  ( -32.13107803565643650, -0.7131008658029172054, 13.60503564500631057 ) ) ;
#12864=AXIS2_PLACEMENT_3D ( 'NONE', #13968, #9360, #21165 ) ;
#12875=B_SPLINE_CURVE_WITH_KNOTS ( 'NONE', 3,
 ( #872, #20894, #18425, #28455, #17752, #28103, #2972, #20699, #199, #20540, #7592, #2662 ),
 .UNSPECIFIED., .F., .F.,
 ( 4, 2, 2, 2, 2, 4 ),
 ( 0.0003422200191418629670, 0.002082436906217386297, 0.003822653793292909736, 0.005562870680368433608, 0.006432979123906195328, 0.007303087567443957047 ),
 .UNSPECIFIED. ) ;
#12877=ADVANCED_FACE ( 'NONE', ( #22518 ), #24487, .F. ) ;
#12891=DIRECTION ( 'NONE',  ( 1.000000000000000000, -0.000000000000000000, -0.000000000000000000 ) ) ;
#12892=CARTESIAN_POINT ( 'NONE',  ( -0.4122223024762697863, 11.86918370369814113, -4.535591127112307497 ) ) ;
#12896=DIRECTION ( 'NONE',  ( 0.000000000000000000, 0.000000000000000000, -1.000000000000000000 ) ) ;
#12898=FACE_OUTER_BOUND ( 'NONE', #4803, .T. ) ;
#12911=EDGE_CURVE ( 'NONE', #5110, #10609, #17371, .T. ) ;
#12914=EDGE_CURVE ( 'NONE', #27037, #14564, #4124, .T. ) ;
#12917=CARTESIAN_POINT ( 'NONE',  ( 51.92400919103563695, -5.935454207752202116, -13.56214536183033381 ) ) ;
#12920=CARTESIAN_POINT ( 'NONE',  ( -43.49202504458321528, -4.177434381965055010, 52.06022946855918576 ) ) ;
#12922=CARTESIAN_POINT ( 'NONE',  ( -33.74072439236259413, -1.979772501351858782, 80.74990046129943266 ) ) ;
#12935=B_SPLINE_CURVE_WITH_KNOTS ( 'NONE', 3,
 ( #24244, #17009, #26547, #26391, #27036, #4549, #1918, #21446, #3900, #13925, #14565, #11939, #1763, #31800, #21774, #19308, #6531, #29333, #2085, #16855, #11447, #23920, #26875, #12112, #1431, #4387, #31961, #9483, #19479, #24568, #31481, #22102, #10460, #15380, #24905, #276 ),
 .UNSPECIFIED., .F., .F.,
 ( 4, 2, 2, 2, 2, 2, 2, 2, 2, 2, 2, 2, 2, 2, 2, 2, 2, 4 ),
 ( 0.000000000000000000, 0.0006656200208596486576, 0.001331240041719297315, 0.002662480083438598967, 0.003993720125157899752, 0.004659340146017551879, 0.005324960166877204006, 0.005990580187736854398, 0.006656200208596505657, 0.007987440250315808177, 0.009318680292035112431, 0.01064992033375441495, 0.01331240041719302172, 0.01464364045891232077, 0.01597488050063161982, 0.01863736058407022139, 0.01996860062578952391, 0.02129984066750881949 ),
 .UNSPECIFIED. ) ;
#12944=ORIENTED_EDGE ( 'NONE', *, *, #21005, .T. ) ;
#12945=ORIENTED_EDGE ( 'NONE', *, *, #6930, .F. ) ;
#12950=EDGE_CURVE ( 'NONE', #26, #4564, #9379, .T. ) ;
#12955=CARTESIAN_POINT ( 'NONE',  ( 21.09785597605719332, -5.935454207752198563, 47.04930799450051637 ) ) ;
#12962=ORIENTED_EDGE ( 'NONE', *, *, #31546, .F. ) ;
#12963=VERTEX_POINT ( 'NONE', #3137 ) ;
#12966=CARTESIAN_POINT ( 'NONE',  ( 46.86424029186792950, 10.39233698702945929, 98.46444777423641881 ) ) ;
#12994=ORIENTED_EDGE ( 'NONE', *, *, #24297, .F. ) ;
#12997=DIRECTION ( 'NONE',  ( -0.000000000000000000, -1.000000000000000000, -0.000000000000000000 ) ) ;
#13003=CARTESIAN_POINT ( 'NONE',  ( 21.09785597605719332, -16.63545420775219696, 126.2593585008393831 ) ) ;
#13012=CARTESIAN_POINT ( 'NONE',  ( 52.96898779464280693, 2.854128177266950672, 98.92834977772137961 ) ) ;
#13013=VERTEX_POINT ( 'NONE', #26763 ) ;
#13025=CARTESIAN_POINT ( 'NONE',  ( -34.35545778780984705, 11.92558985988975806, 53.76626552113134494 ) ) ;
#13028=VECTOR ( 'NONE', #23455, 1000.000000000000000 ) ;
#13033=DIRECTION ( 'NONE',  ( 0.000000000000000000, -1.000000000000000000, 0.000000000000000000 ) ) ;
#13046=CARTESIAN_POINT ( 'NONE',  ( 0.1396058544580265071, 11.92558985988972964, 99.69197238745105949 ) ) ;
#13048=ORIENTED_EDGE ( 'NONE', *, *, #29820, .T. ) ;
#13049=CARTESIAN_POINT ( 'NONE',  ( 77.00054885935878701, -4.576799740321065180, 80.22553795869546889 ) ) ;
#13053=CARTESIAN_POINT ( 'NONE',  ( 21.09785597605719332, 12.39166260509097484, -7.501994455397703376 ) ) ;
#13062=EDGE_CURVE ( 'NONE', #18205, #16844, #23993, .T. ) ;
#13077=CARTESIAN_POINT ( 'NONE',  ( 81.46980107077142463, -5.935454207752202116, 16.07118271501079576 ) ) ;
#13079=ORIENTED_EDGE ( 'NONE', *, *, #17750, .T. ) ;
#13080=CARTESIAN_POINT ( 'NONE',  ( -9.474781401982005136, 5.388785998227653806, 97.43646483284780402 ) ) ;
#13082=CARTESIAN_POINT ( 'NONE',  ( -37.03881032980826404, -5.627210490873816084, 79.10483057741561197 ) ) ;
#13086=CARTESIAN_POINT ( 'NONE',  ( -11.12022268173655526, -5.523138741469210800, 104.1124227880728768 ) ) ;
#13088=CARTESIAN_POINT ( 'NONE',  ( 21.09785597605720042, 13.06454579224780055, 101.7935565934706261 ) ) ;
#13103=ADVANCED_FACE ( 'NONE', ( #21497, #24134, #6097, #1652 ), #24035, .T. ) ;
#13110=ORIENTED_EDGE ( 'NONE', *, *, #31465, .T. ) ;
#13113=EDGE_LOOP ( 'NONE', ( #13981, #31197, #11758, #11762 ) ) ;
#13114=CARTESIAN_POINT ( 'NONE',  ( 71.49893360114315044, 9.702389020015065313, 20.34850893876554778 ) ) ;
#13116=AXIS2_PLACEMENT_3D ( 'NONE', #25616, #28567, #18211 ) ;
#13124=CIRCLE ( 'NONE', #22543, 48.97546517713167447 ) ;
#13130=CARTESIAN_POINT ( 'NONE',  ( 54.82846636219741754, -2.304636120132642407, 102.0807631826289565 ) ) ;
#13142=DIRECTION ( 'NONE',  ( 0.000000000000000000, -1.000000000000000000, 0.000000000000000000 ) ) ;
#13149=AXIS2_PLACEMENT_3D ( 'NONE', #29727, #12167, #14794 ) ;
#13153=CYLINDRICAL_SURFACE ( 'NONE', #7581, 2.500000000000002220 ) ;
#13155=DIRECTION ( 'NONE',  ( -0.000000000000000000, -1.000000000000000000, -0.000000000000000000 ) ) ;
#13157=VERTEX_POINT ( 'NONE', #26927 ) ;
#13158=CARTESIAN_POINT ( 'NONE',  ( -38.65545646816406133, 11.23353054871637013, 71.85461326257689052 ) ) ;
#13161=CARTESIAN_POINT ( 'NONE',  ( 52.31884008669100439, -5.919445383190008236, -10.81522751587263720 ) ) ;
#13163=DIRECTION ( 'NONE',  ( 0.000000000000000000, 0.000000000000000000, -1.000000000000000000 ) ) ;
#13179=EDGE_CURVE ( 'NONE', #5971, #30781, #7067, .T. ) ;
#13194=CARTESIAN_POINT ( 'NONE',  ( -34.60695214214126736, 11.63096289306646902, 52.99612787234249822 ) ) ;
#13204=DIRECTION ( 'NONE',  ( 0.000000000000000000, 0.000000000000000000, -1.000000000000000000 ) ) ;
#13217=DIRECTION ( 'NONE',  ( 0.000000000000000000, -1.000000000000000000, 0.000000000000000000 ) ) ;
#13236=AXIS2_PLACEMENT_3D ( 'NONE', #23889, #11584, #28656 ) ;
#13249=CARTESIAN_POINT ( 'NONE',  ( -34.95900968110382223, 11.10530621426302034, 41.68526607318150212 ) ) ;
#13267=DIRECTION ( 'NONE',  ( 0.000000000000000000, 0.000000000000000000, -1.000000000000000000 ) ) ;
#13269=VERTEX_POINT ( 'NONE', #4600 ) ;
#13270=EDGE_CURVE ( 'NONE', #26491, #30456, #20023, .T. ) ;
#13272=AXIS2_PLACEMENT_3D ( 'NONE', #28687, #6202, #18983 ) ;
#13273=VERTEX_POINT ( 'NONE', #24625 ) ;
#13276=CARTESIAN_POINT ( 'NONE',  ( -8.419250967200506253, 6.662067023026856383, 98.79925651794950170 ) ) ;
#13281=PRODUCT ( 'Frame', 'Frame', '', ( #162 ) ) ;
#13283=DIRECTION ( 'NONE',  ( 8.969280666154383504E-16, 0.000000000000000000, -1.000000000000000000 ) ) ;
#13310=CARTESIAN_POINT ( 'NONE',  ( 100.3079064823960493, -15.93545420775219945, 44.54930799450134771 ) ) ;
#13315=EDGE_CURVE ( 'NONE', #27037, #31589, #26150, .T. ) ;
#13317=ORIENTED_EDGE ( 'NONE', *, *, #32117, .F. ) ;
#13320=FACE_OUTER_BOUND ( 'NONE', #9110, .T. ) ;
#13324=EDGE_CURVE ( 'NONE', #22091, #22386, #19283, .T. ) ;
#13326=CARTESIAN_POINT ( 'NONE',  ( 81.63177831856063449, -5.935454207752202116, 16.07118271501079576 ) ) ;
#13329=CARTESIAN_POINT ( 'NONE',  ( -63.90214402394282445, -5.935454207752198563, 54.04930799450053058 ) ) ;
#13339=CARTESIAN_POINT ( 'NONE',  ( 54.06624571392757161, 0.6013300790671899376, 99.71667309011171199 ) ) ;
#13343=VERTEX_POINT ( 'NONE', #2945 ) ;
#13347=CARTESIAN_POINT ( 'NONE',  ( -39.42933158985913877, -5.935956174194163104, 77.90091477773695772 ) ) ;
#13357=ADVANCED_FACE ( 'NONE', ( #25284 ), #30699, .F. ) ;
#13361=CARTESIAN_POINT ( 'NONE',  ( -63.90214402394282445, 9.925589859889720756, 42.04930799450051637 ) ) ;
#13363=FACE_OUTER_BOUND ( 'NONE', #24367, .T. ) ;
#13367=AXIS2_PLACEMENT_3D ( 'NONE', #23156, #15599, #5443 ) ;
#13368=CARTESIAN_POINT ( 'NONE',  ( -3.659396493201523270, 10.95165879486606997, -3.626357375625654633 ) ) ;
#13372=CARTESIAN_POINT ( 'NONE',  ( 0.6836613156275053171, 11.92558985988973497, -4.944603100128008855 ) ) ;
#13375=DIRECTION ( 'NONE',  ( 0.000000000000000000, 0.000000000000000000, 1.000000000000000000 ) ) ;
#13378=CARTESIAN_POINT ( 'NONE',  ( 78.34648107337082479, -4.961365878511911909, 79.93084625785569131 ) ) ;
#13385=FACE_OUTER_BOUND ( 'NONE', #21897, .T. ) ;
#13387=CARTESIAN_POINT ( 'NONE',  ( 54.82593361024983381, -2.878806504921699094, -8.356670642478869482 ) ) ;
#13396=AXIS2_PLACEMENT_3D ( 'NONE', #32091, #14210, #19267 ) ;
#13399=CARTESIAN_POINT ( 'NONE',  ( -36.84960911689896079, -5.942107891656587704, 78.14337069435562455 ) ) ;
#13403=CARTESIAN_POINT ( 'NONE',  ( -35.09136543214532367, 10.88994114954489234, 41.81952777619033412 ) ) ;
#13405=CARTESIAN_POINT ( 'NONE',  ( -5.602943079677954685, 9.702389020015065313, 106.8025418868326284 ) ) ;
#13407=CARTESIAN_POINT ( 'NONE',  ( -34.34753876910989590, -2.938577454171012349, 80.77644560816827379 ) ) ;
#13416=CARTESIAN_POINT ( 'NONE',  ( -35.89491889087902621, 10.89025382816431531, 52.27940093726513737 ) ) ;
#13425=CIRCLE ( 'NONE', #7657, 71.29999999999996874 ) ;
#13433=UNCERTAINTY_MEASURE_WITH_UNIT (LENGTH_MEASURE( 1.000000000000000082E-05 ), #3258, 'distance_accuracy_value', 'NONE');
#13436=EDGE_LOOP ( 'NONE', ( #11111, #14539, #11617, #17943 ) ) ;
#13444=CARTESIAN_POINT ( 'NONE',  ( 52.57325962015784171, -5.881344816830202049, 106.1937027734941523 ) ) ;
#13448=FACE_OUTER_BOUND ( 'NONE', #8845, .T. ) ;
#13451=CARTESIAN_POINT ( 'NONE',  ( 45.85675386737194259, 10.95084857405596068, 98.61391123392256475 ) ) ;
#13452=CARTESIAN_POINT ( 'NONE',  ( 54.00540614691084329, -4.922489993312315626, 104.2573514652678739 ) ) ;
#13458=FACE_OUTER_BOUND ( 'NONE', #13113, .T. ) ;
#13459=CARTESIAN_POINT ( 'NONE',  ( 52.07598125554711999, -5.935454207752202116, 105.0538709090500333 ) ) ;
#13473=EDGE_LOOP ( 'NONE', ( #8795, #14830 ) ) ;
#13489=ADVANCED_FACE ( 'NONE', ( #23773, #1285 ), #23622, .T. ) ;
#13503=EDGE_CURVE ( 'NONE', #8733, #8315, #6777, .T. ) ;
#13504=CARTESIAN_POINT ( 'NONE',  ( -39.41060154113746705, -5.935741391424327773, 77.97157130629763344 ) ) ;
#13506=VECTOR ( 'NONE', #6434, 1000.000000000000000 ) ;
#13511=DIRECTION ( 'NONE',  ( 0.000000000000000000, -1.000000000000000000, 0.000000000000000000 ) ) ;
#13516=CARTESIAN_POINT ( 'NONE',  ( 71.55763488011925233, 9.127627432390726270, 19.66944483935173338 ) ) ;
#13540=ADVANCED_FACE ( 'NONE', ( #21796 ), #19504, .F. ) ;
#13541=CARTESIAN_POINT ( 'NONE',  ( 73.03377152639730241, 11.55930814891847191, 23.89416354099248707 ) ) ;
#13547=CIRCLE ( 'NONE', #24006, 67.18681090792816235 ) ;
#13553=CARTESIAN_POINT ( 'NONE',  ( -35.51007442658541180, 10.17492932633761171, 42.04930799450051637 ) ) ;
#13557=DIRECTION ( 'NONE',  ( 0.000000000000000000, 0.000000000000000000, -1.000000000000000000 ) ) ;
#13578=CARTESIAN_POINT ( 'NONE',  ( -9.925114359954182675, -5.937449718911893548, -13.57859485750651629 ) ) ;
#13585=CARTESIAN_POINT ( 'NONE',  ( -7.928239498742526870, 7.324825086315946976, 98.65516431386642182 ) ) ;
#13588=EDGE_LOOP ( 'NONE', ( #208, #17754, #4586, #8304 ) ) ;
#13590=CARTESIAN_POINT ( 'NONE',  ( 71.49893360114316465, 5.388785998227650254, 16.47908017486093257 ) ) ;
#13595=CARTESIAN_POINT ( 'NONE',  ( 52.89687679232817175, -5.771419034597327524, 105.5847057727601026 ) ) ;
#13613=CARTESIAN_POINT ( 'NONE',  ( -30.63875195204110469, 3.314680658590930751, 15.43500191121110809 ) ) ;
#13617=DIRECTION ( 'NONE',  ( -1.000000000000000000, 0.000000000000000000, 2.775557561562888984E-15 ) ) ;
#13619=CARTESIAN_POINT ( 'NONE',  ( 21.09785597605719332, -5.721341737285094098, 47.04930799450051637 ) ) ;
#13625=CIRCLE ( 'NONE', #17812, 84.30000000000001137 ) ;
#13639=VERTEX_POINT ( 'NONE', #5989 ) ;
#13643=ORIENTED_EDGE ( 'NONE', *, *, #2449, .F. ) ;
#13653=CARTESIAN_POINT ( 'NONE',  ( 106.0978559760576161, -5.935454207751966749, 16.07118271501087747 ) ) ;
#13655=DIRECTION ( 'NONE',  ( 0.000000000000000000, 0.000000000000000000, -1.000000000000000000 ) ) ;
#13656=EDGE_LOOP ( 'NONE', ( #17193, #17623, #4096, #18341, #9831 ) ) ;
#13666=CARTESIAN_POINT ( 'NONE',  ( -39.40038788600242015, -5.936129073955724422, 77.93577773595035296 ) ) ;
#13672=DIRECTION ( 'NONE',  ( 1.775451498209539969E-15, 0.000000000000000000, -1.000000000000000000 ) ) ;
#13679=CARTESIAN_POINT ( 'NONE',  ( -58.11219453028166981, -16.63545420775219696, 49.54930799450023926 ) ) ;
#13694=DIRECTION ( 'NONE',  ( -1.000000000000000000, -0.000000000000000000, -3.491481338843133355E-15 ) ) ;
#13703=CARTESIAN_POINT ( 'NONE',  ( 50.12395145085690729, 7.324825086315956746, -4.556548324865391741 ) ) ;
#13711=B_SPLINE_CURVE_WITH_KNOTS ( 'NONE', 3,
 ( #9553, #14807, #29410, #2324, #32363, #12343, #9873, #22493, #31869, #4951 ),
 .UNSPECIFIED., .F., .F.,
 ( 4, 2, 2, 2, 4 ),
 ( 0.0006716755660531790973, 0.002413276598758981421, 0.004154877631464783637, 0.005896478664170586720, 0.007638079696876388935 ),
 .UNSPECIFIED. ) ;
#13712=AXIS2_PLACEMENT_3D ( 'NONE', #27931, #2494, #22506 ) ;
#13715=CARTESIAN_POINT ( 'NONE',  ( 81.76548788166886084, -5.935709855254037493, 77.87985502756478695 ) ) ;
#13716=EDGE_CURVE ( 'NONE', #16751, #14290, #1056, .T. ) ;
#13724=CARTESIAN_POINT ( 'NONE',  ( 21.09785597605720397, -15.93545420775219945, -24.95069200549946586 ) ) ;
#13731=ORIENTED_EDGE ( 'NONE', *, *, #12700, .T. ) ;
#13744=ORIENTED_EDGE ( 'NONE', *, *, #632, .F. ) ;
#13759=LINE ( 'NONE', #31157, #16394 ) ;
#13761=EDGE_CURVE ( 'NONE', #23976, #24923, #14144, .T. ) ;
#13769=DIRECTION ( 'NONE',  ( 0.000000000000000000, 0.000000000000000000, -1.000000000000000000 ) ) ;
#13771=CARTESIAN_POINT ( 'NONE',  ( 21.09785597605720042, -5.935454207752331790, 112.8077566132119927 ) ) ;
#13772=VECTOR ( 'NONE', #28028, 1000.000000000000000 ) ;
#13773=CARTESIAN_POINT ( 'NONE',  ( -0.4130478171086108263, 11.86909835304794569, -5.401369334345301532 ) ) ;
#13782=ORIENTED_EDGE ( 'NONE', *, *, #23423, .F. ) ;
#13797=CARTESIAN_POINT ( 'NONE',  ( 77.62364571523254142, -4.258649047046835889, 13.70170648863429896 ) ) ;
#13799=ORIENTED_EDGE ( 'NONE', *, *, #15397, .T. ) ;
#13831=CARTESIAN_POINT ( 'NONE',  ( 21.09785597605719332, -16.63545420775219696, -37.16074251183835031 ) ) ;
#13838=CARTESIAN_POINT ( 'NONE',  ( 71.79669559076680230, 7.198184577528758510, 17.90250836569788007 ) ) ;
#13839=ORIENTED_EDGE ( 'NONE', *, *, #28636, .T. ) ;
#13844=ORIENTED_EDGE ( 'NONE', *, *, #25855, .F. ) ;
#13852=CYLINDRICAL_SURFACE ( 'NONE', #9011, 2.000000000000001776 ) ;
#13861=DIRECTION ( 'NONE',  ( 0.000000000000000000, -1.000000000000000000, -0.000000000000000000 ) ) ;
#13864=EDGE_LOOP ( 'NONE', ( #2201, #15634, #20976, #2105 ) ) ;
#13865=EDGE_CURVE ( 'NONE', #12758, #5905, #7849, .T. ) ;
#13878=CARTESIAN_POINT ( 'NONE',  ( 21.09785597605719332, 16.33322284159648063, 47.04930799450051637 ) ) ;
#13884=ORIENTED_EDGE ( 'NONE', *, *, #27912, .F. ) ;
#13889=VERTEX_POINT ( 'NONE', #1864 ) ;
#13898=EDGE_CURVE ( 'NONE', #31626, #23399, #24179, .T. ) ;
#13901=EDGE_CURVE ( 'NONE', #28492, #31580, #8373, .T. ) ;
#13905=EDGE_LOOP ( 'NONE', ( #26203, #12178 ) ) ;
#13908=CIRCLE ( 'NONE', #13396, 40.48742189997368257 ) ;
#13912=EDGE_CURVE ( 'NONE', #29041, #20681, #18757, .T. ) ;
#13924=CIRCLE ( 'NONE', #14472, 40.48742189997368257 ) ;
#13925=CARTESIAN_POINT ( 'NONE',  ( -12.35638036371648774, -4.032327822094595504, -8.334620977867299274 ) ) ;
#13932=PLANE ( 'NONE',  #2243 ) ;
#13950=EDGE_CURVE ( 'NONE', #25630, #16490, #22701, .T. ) ;
#13964=B_SPLINE_CURVE_WITH_KNOTS ( 'NONE', 3,
 ( #19685, #19524, #29383, #1809, #29058, #31846, #14615, #6578 ),
 .UNSPECIFIED., .F., .F.,
 ( 4, 2, 2, 4 ),
 ( 8.560449982191426041E-05, 0.0006851562598348886557, 0.0009849321398413680810, 0.001284708019847847615 ),
 .UNSPECIFIED. ) ;
#13968=CARTESIAN_POINT ( 'NONE',  ( 21.09785597605719332, 11.92558985988973497, 47.04930799450051637 ) ) ;
#13979=CARTESIAN_POINT ( 'NONE',  ( -12.63275441008301669, -2.304636120132624644, -7.982147193627917581 ) ) ;
#13981=ORIENTED_EDGE ( 'NONE', *, *, #9949, .F. ) ;
#13986=ADVANCED_FACE ( 'NONE', ( #12041 ), #8026, .F. ) ;
#13999=DIRECTION ( 'NONE',  ( 0.000000000000000000, -0.000000000000000000, 1.000000000000000000 ) ) ;
#14012=EDGE_LOOP ( 'NONE', ( #6632, #302, #21720, #31603 ) ) ;
#14013=CARTESIAN_POINT ( 'NONE',  ( -39.57165970433088376, -5.936116385392971040, 77.92184100968836447 ) ) ;
#14014=FACE_OUTER_BOUND ( 'NONE', #13864, .T. ) ;
#14022=ORIENTED_EDGE ( 'NONE', *, *, #6625, .T. ) ;
#14023=CARTESIAN_POINT ( 'NONE',  ( 73.18954489356450210, 11.69686719848734313, 24.43675172218812008 ) ) ;
#14030=CARTESIAN_POINT ( 'NONE',  ( -29.74268752149416173, 11.25807467393579309, 71.06788596905158784 ) ) ;
#14044=DIRECTION ( 'NONE',  ( -0.000000000000000000, -1.000000000000000000, -0.000000000000000000 ) ) ;
#14053=EDGE_CURVE ( 'NONE', #26270, #649, #15000, .T. ) ;
#14064=AXIS2_PLACEMENT_3D ( 'NONE', #30427, #378, #12385 ) ;
#14066=CIRCLE ( 'NONE', #29782, 48.63405236513555963 ) ;
#14089=CARTESIAN_POINT ( 'NONE',  ( 47.79865503179234310, 9.702389020015065313, 97.51081847724526597 ) ) ;
#14090=FACE_BOUND ( 'NONE', #23411, .T. ) ;
#14097=DIRECTION ( 'NONE',  ( 1.000000000000000000, -0.000000000000000000, -0.000000000000000000 ) ) ;
#14098=CARTESIAN_POINT ( 'NONE',  ( 71.55936645880184699, 9.702389020015065313, 73.75010705023584023 ) ) ;
#14099=DIRECTION ( 'NONE',  ( -1.000000000000000000, 0.000000000000000000, -1.110223024625155594E-14 ) ) ;
#14101=CARTESIAN_POINT ( 'NONE',  ( 21.09785597605719332, 24.56454579224780232, 47.04930799450051637 ) ) ;
#14106=LINE ( 'NONE', #24760, #494 ) ;
#14112=DIRECTION ( 'NONE',  ( 0.000000000000000000, -0.7071067811865378028, -0.7071067811865573427 ) ) ;
#14117=AXIS2_PLACEMENT_3D ( 'NONE', #12498, #22481, #11 ) ;
#14124=DIRECTION ( 'NONE',  ( 0.000000000000000000, 0.000000000000000000, -1.000000000000000000 ) ) ;
#14126=ADVANCED_FACE ( 'NONE', ( #13320 ), #10490, .F. ) ;
#14129=EDGE_LOOP ( 'NONE', ( #23575, #17191, #27055, #16174 ) ) ;
#14132=CARTESIAN_POINT ( 'NONE',  ( -43.35833523721896654, -3.935454207752183020, 52.04930799450050927 ) ) ;
#14133=CIRCLE ( 'NONE', #7834, 55.53141649511111666 ) ;
#14135=AXIS2_PLACEMENT_3D ( 'NONE', #5660, #251, #15666 ) ;
#14138=CARTESIAN_POINT ( 'NONE',  ( -5.929450684728940324, 9.438446991585315970, -4.311106055539630333 ) ) ;
#14144=CIRCLE ( 'NONE', #3654, 2.500000000000002220 ) ;
#14148=ORIENTED_EDGE ( 'NONE', *, *, #3336, .F. ) ;
#14149=CARTESIAN_POINT ( 'NONE',  ( 21.09785597605720397, -16.63545420775219696, 119.2593585008392978 ) ) ;
#14157=DIRECTION ( 'NONE',  ( 0.000000000000000000, 0.000000000000000000, 1.000000000000000000 ) ) ;
#14162=DIRECTION ( 'NONE',  ( 0.000000000000000000, 0.000000000000000000, -1.000000000000000000 ) ) ;
#14171=AXIS2_PLACEMENT_3D ( 'NONE', #11360, #1178, #31554 ) ;
#14185=CIRCLE ( 'NONE', #17821, 55.85791022362053582 ) ;
#14186=DIRECTION ( 'NONE',  ( -0.000000000000000000, 1.000000000000000000, -0.000000000000000000 ) ) ;
#14196=AXIS2_PLACEMENT_3D ( 'NONE', #2152, #9704, #1822 ) ;
#14197=DIRECTION ( 'NONE',  ( 0.000000000000000000, 0.000000000000000000, -1.000000000000000000 ) ) ;
#14199=ADVANCED_FACE ( 'NONE', ( #499 ), #22825, .F. ) ;
#14208=DIRECTION ( 'NONE',  ( -0.000000000000000000, 1.000000000000000000, -0.000000000000000000 ) ) ;
#14210=DIRECTION ( 'NONE',  ( -0.000000000000000000, -1.000000000000000000, -0.000000000000000000 ) ) ;
#14215=DIRECTION ( 'NONE',  ( -0.000000000000000000, -1.000000000000000000, -0.000000000000000000 ) ) ;
#14216=DIRECTION ( 'NONE',  ( -0.000000000000000000, -1.000000000000000000, -0.000000000000000000 ) ) ;
#14230=CIRCLE ( 'NONE', #13712, 67.18681090792816235 ) ;
#14232=ORIENTED_EDGE ( 'NONE', *, *, #16193, .T. ) ;
#14234=EDGE_CURVE ( 'NONE', #21709, #21280, #20524, .T. ) ;
#14265=CARTESIAN_POINT ( 'NONE',  ( -29.27337757263006424, -5.935454207752202116, 16.07118271501078866 ) ) ;
#14287=CARTESIAN_POINT ( 'NONE',  ( 76.46605017418944783, -2.833757427854269206, 13.30711217131973356 ) ) ;
#14290=VERTEX_POINT ( 'NONE', #29370 ) ;
#14294=VERTEX_POINT ( 'NONE', #6398 ) ;
#14300=ORIENTED_EDGE ( 'NONE', *, *, #31498, .T. ) ;
#14301=CARTESIAN_POINT ( 'NONE',  ( -11.70362862524498304, -5.043292969097927347, -10.29680806063067067 ) ) ;
#14322=CARTESIAN_POINT ( 'NONE',  ( 51.00445379728992634, 6.094407115496624172, -3.914104645325461540 ) ) ;
#14323=DIRECTION ( 'NONE',  ( 0.000000000000000000, 0.000000000000000000, -1.000000000000000000 ) ) ;
#14327=AXIS2_PLACEMENT_3D ( 'NONE', #31261, #28317, #21069 ) ;
#14332=VERTEX_POINT ( 'NONE', #23637 ) ;
#14338=CARTESIAN_POINT ( 'NONE',  ( -39.57293394879278026, -5.936033350080357707, 77.90897538353701179 ) ) ;
#14347=VECTOR ( 'NONE', #12444, 1000.000000000000000 ) ;
#14349=CARTESIAN_POINT ( 'NONE',  ( 21.09785597605719332, 15.56454579224779877, 47.04930799450051637 ) ) ;
#14353=CIRCLE ( 'NONE', #19587, 55.00000000000000000 ) ;
#14362=DIRECTION ( 'NONE',  ( 0.000000000000000000, -1.000000000000000000, 0.000000000000000000 ) ) ;
#14364=EDGE_LOOP ( 'NONE', ( #10271, #2960, #28672, #29435, #15347, #16657, #6669, #10232, #2823, #13799, #310, #24391 ) ) ;
#14365=CARTESIAN_POINT ( 'NONE',  ( -9.880269303432738681, -5.935454207752202116, -13.48461434800281289 ) ) ;
#14375=CARTESIAN_POINT ( 'NONE',  ( 21.09785597605719332, -15.93545420775219945, 123.7593585008393831 ) ) ;
#14387=ORIENTED_EDGE ( 'NONE', *, *, #11861, .T. ) ;
#14396=B_SPLINE_CURVE_WITH_KNOTS ( 'NONE', 3,
 ( #5732, #10674, #12966, #13451, #28059, #25907, #20978, #12807, #23290, #23446, #803, #18186 ),
 .UNSPECIFIED., .F., .F.,
 ( 4, 2, 2, 2, 2, 4 ),
 ( 0.0003422370341462309374, 0.002080102550335785096, 0.003817968066525339200, 0.005555833582714892437, 0.006424766340809669705, 0.007293699098904446974 ),
 .UNSPECIFIED. ) ;
#14416=DIRECTION ( 'NONE',  ( -1.313185983435984691E-29, 1.000000000000000000, 3.761114140369702165E-15 ) ) ;
#14418=ORIENTED_EDGE ( 'NONE', *, *, #31143, .T. ) ;
#14435=ADVANCED_FACE ( 'NONE', ( #7987 ), #28846, .F. ) ;
#14440=CARTESIAN_POINT ( 'NONE',  ( 51.96080742951041742, -5.936631694656545832, -13.43417697512268916 ) ) ;
#14442=DIRECTION ( 'NONE',  ( -0.000000000000000000, -0.000000000000000000, 1.000000000000000000 ) ) ;
#14444=CIRCLE ( 'NONE', #30689, 66.44011198581388555 ) ;
#14448=CARTESIAN_POINT ( 'NONE',  ( 76.70546203173246624, -3.171899563477270867, 13.33972164219158607 ) ) ;
#14451=ORIENTED_EDGE ( 'NONE', *, *, #3108, .F. ) ;
#14452=CYLINDRICAL_SURFACE ( 'NONE', #3908, 10.00000000000000533 ) ;
#14456=DIRECTION ( 'NONE',  ( 0.000000000000000000, 1.000000000000000000, 0.000000000000000000 ) ) ;
#14459=ORIENTED_EDGE ( 'NONE', *, *, #21922, .F. ) ;
#14464=EDGE_CURVE ( 'NONE', #8721, #29191, #15522, .T. ) ;
#14465=EDGE_CURVE ( 'NONE', #22386, #22091, #2882, .T. ) ;
#14466=ORIENTED_EDGE ( 'NONE', *, *, #18227, .T. ) ;
#14467=CARTESIAN_POINT ( 'NONE',  ( -8.414270849481495063, 6.668192824305379851, -4.699568316320720918 ) ) ;
#14468=LINE ( 'NONE', #24792, #13 ) ;
#14472=AXIS2_PLACEMENT_3D ( 'NONE', #12852, #17921, #30406 ) ;
#14487=CARTESIAN_POINT ( 'NONE',  ( 48.14616182813506384, 9.421471677506305653, -3.404495637954462417 ) ) ;
#14494=DIRECTION ( 'NONE',  ( -0.000000000000000000, -1.000000000000000000, -0.000000000000000000 ) ) ;
#14495=EDGE_LOOP ( 'NONE', ( #5367, #27976, #20306, #31148 ) ) ;
#14499=CARTESIAN_POINT ( 'NONE',  ( -29.36860851563585584, 8.903991466124205445, 19.42204177740639892 ) ) ;
#14513=DIRECTION ( 'NONE',  ( 0.000000000000000000, -1.000000000000000000, 0.000000000000000000 ) ) ;
#14521=CARTESIAN_POINT ( 'NONE',  ( -29.47038852791792962, 8.010743491677633443, 75.51333467491832607 ) ) ;
#14524=CARTESIAN_POINT ( 'NONE',  ( 51.92400919103563695, -5.935454207752202116, -13.65255231306078798 ) ) ;
#14529=ORIENTED_EDGE ( 'NONE', *, *, #27674, .F. ) ;
#14531=DIRECTION ( 'NONE',  ( 0.000000000000000000, 0.000000000000000000, -1.000000000000000000 ) ) ;
#14539=ORIENTED_EDGE ( 'NONE', *, *, #7256, .T. ) ;
#14558=DIRECTION ( 'NONE',  ( 0.000000000000000000, -1.000000000000000000, 0.000000000000000000 ) ) ;
#14563=CARTESIAN_POINT ( 'NONE',  ( -8.565981920724627940, 6.453333540778367627, 97.92432209181883707 ) ) ;
#14564=VERTEX_POINT ( 'NONE', #2886 ) ;
#14565=CARTESIAN_POINT ( 'NONE',  ( -12.42032014790552807, -3.872051342217444070, -8.192007789466410728 ) ) ;
#14585=CARTESIAN_POINT ( 'NONE',  ( -29.27337757263006424, -0.7885452029232787874, 13.38511290719907798 ) ) ;
#14591=VERTEX_POINT ( 'NONE', #6153 ) ;
#14595=CIRCLE ( 'NONE', #16664, 56.65825807113184709 ) ;
#14597=CARTESIAN_POINT ( 'NONE',  ( 21.09785597605719332, 25.13358275951983956, 47.04930799450051637 ) ) ;
#14598=EDGE_CURVE ( 'NONE', #3624, #649, #19274, .T. ) ;
#14615=CARTESIAN_POINT ( 'NONE',  ( -45.73387052288833132, -5.935454207752206557, 40.15016479612525302 ) ) ;
#14623=CARTESIAN_POINT ( 'NONE',  ( -7.668010133714219023, 7.652955895019252885, -4.493996600949651032 ) ) ;
#14626=CARTESIAN_POINT ( 'NONE',  ( 21.09785597605719332, -5.935454207752198563, 47.04930799450051637 ) ) ;
#14629=AXIS2_PLACEMENT_3D ( 'NONE', #14349, #14513, #9752 ) ;
#14632=EDGE_CURVE ( 'NONE', #22873, #7835, #7232, .T. ) ;
#14635=EDGE_LOOP ( 'NONE', ( #22033, #1818, #10510, #5529 ) ) ;
#14643=EDGE_CURVE ( 'NONE', #11793, #17109, #23273, .T. ) ;
#14644=DIRECTION ( 'NONE',  ( -0.000000000000000000, 1.000000000000000000, -0.000000000000000000 ) ) ;
#14654=CARTESIAN_POINT ( 'NONE',  ( 21.09785597605719332, 11.92558985988973497, 47.04930799450051637 ) ) ;
#14660=CARTESIAN_POINT ( 'NONE',  ( -29.83711070102105012, 6.212614032769436356, 17.22340695172378844 ) ) ;
#14663=CARTESIAN_POINT ( 'NONE',  ( 71.48501281440437083, 8.310461108307681144, 75.47198155259907537 ) ) ;
#14679=EDGE_CURVE ( 'NONE', #12963, #13273, #4081, .T. ) ;
#14680=ORIENTED_EDGE ( 'NONE', *, *, #29239, .T. ) ;
#14681=DIRECTION ( 'NONE',  ( -0.000000000000000000, -1.000000000000000000, -0.000000000000000000 ) ) ;
#14689=CARTESIAN_POINT ( 'NONE',  ( -29.54697681637456697, 7.561619403635258863, 75.88267709390528637 ) ) ;
#14691=ORIENTED_EDGE ( 'NONE', *, *, #8418, .T. ) ;
#14696=CARTESIAN_POINT ( 'NONE',  ( 71.77671131497349677, 10.95964320463250807, 71.78996344180542621 ) ) ;
#14697=ORIENTED_EDGE ( 'NONE', *, *, #17652, .T. ) ;
#14709=VECTOR ( 'NONE', #14442, 1000.000000000000000 ) ;
#14718=TOROIDAL_SURFACE ( 'NONE', #20478, 39.69941114636694834, 1.000000000000000000 ) ;
#14725=CARTESIAN_POINT ( 'NONE',  ( 21.09785597605719332, 13.74476430820393347, 47.04930799450051637 ) ) ;
#14733=CARTESIAN_POINT ( 'NONE',  ( -7.783295380925389750, 7.511668073839847359, 97.69862240222212790 ) ) ;
#14745=DIRECTION ( 'NONE',  ( -1.000000000000000000, -0.000000000000000000, -3.491481338843133355E-15 ) ) ;
#14766=DIRECTION ( 'NONE',  ( 0.000000000000000000, 0.000000000000000000, 1.000000000000000000 ) ) ;
#14777=DIRECTION ( 'NONE',  ( 0.000000000000000000, 0.000000000000000000, -1.000000000000000000 ) ) ;
#14793=VERTEX_POINT ( 'NONE', #27635 ) ;
#14794=DIRECTION ( 'NONE',  ( 0.000000000000000000, 0.000000000000000000, -1.000000000000000000 ) ) ;
#14798=FACE_OUTER_BOUND ( 'NONE', #17926, .T. ) ;
#14802=EDGE_CURVE ( 'NONE', #16982, #7700, #4998, .T. ) ;
#14805=ADVANCED_FACE ( 'NONE', ( #25179 ), #27664, .F. ) ;
#14807=CARTESIAN_POINT ( 'NONE',  ( 73.74052036900765472, 11.92558985988972964, 68.00755811609985813 ) ) ;
#14830=ORIENTED_EDGE ( 'NONE', *, *, #17656, .T. ) ;
#14836=VERTEX_POINT ( 'NONE', #22541 ) ;
#14844=ORIENTED_EDGE ( 'NONE', *, *, #20222, .F. ) ;
#14866=AXIS2_PLACEMENT_3D ( 'NONE', #26676, #8791, #6499 ) ;
#14881=ORIENTED_EDGE ( 'NONE', *, *, #16376, .F. ) ;
#14886=CARTESIAN_POINT ( 'NONE',  ( 75.17570804623589709, -2.284241381456150410, 13.31978822362705195 ) ) ;
#14888=CARTESIAN_POINT ( 'NONE',  ( 42.60151274628839246, 11.88152873911358753, -5.399210173220353681 ) ) ;
#14894=CARTESIAN_POINT ( 'NONE',  ( -10.80606256024020873, 2.793366809690227992, 98.94773045085101160 ) ) ;
#14897=CARTESIAN_POINT ( 'NONE',  ( 80.24225075505094651, -5.881344816830196720, 15.57390435040008114 ) ) ;
#14899=CARTESIAN_POINT ( 'NONE',  ( 81.79971628361815306, -5.935454207752202116, 77.87546120947918382 ) ) ;
#14901=EDGE_CURVE ( 'NONE', #5070, #313, #18102, .T. ) ;
#14908=ORIENTED_EDGE ( 'NONE', *, *, #22117, .T. ) ;
#14913=CARTESIAN_POINT ( 'NONE',  ( -4.902144023942810236, 25.56454579224779877, 47.04930799450078638 ) ) ;
#14937=AXIS2_PLACEMENT_3D ( 'NONE', #12955, #18021, #13283 ) ;
#14941=DIRECTION ( 'NONE',  ( -0.000000000000000000, -1.000000000000000000, -0.000000000000000000 ) ) ;
#14945=DIRECTION ( 'NONE',  ( 0.000000000000000000, -1.000000000000000000, 0.000000000000000000 ) ) ;
#14947=EDGE_CURVE ( 'NONE', #26256, #32220, #18246, .T. ) ;
#14950=EDGE_CURVE ( 'NONE', #26169, #13889, #31362, .T. ) ;
#14952=EDGE_LOOP ( 'NONE', ( #23379, #21174, #16722, #3309 ) ) ;
#14955=FACE_OUTER_BOUND ( 'NONE', #17119, .T. ) ;
#14958=CIRCLE ( 'NONE', #7095, 2.500000000000003553 ) ;
#14965=CARTESIAN_POINT ( 'NONE',  ( -38.44253683272001609, -5.930168697284449841, 15.95990681549819534 ) ) ;
#14970=CARTESIAN_POINT ( 'NONE',  ( 21.09785597605719332, 24.74924423484549507, 47.04930799450051637 ) ) ;
#14989=ADVANCED_FACE ( 'NONE', ( #18254 ), #3330, .F. ) ;
#14994=CARTESIAN_POINT ( 'NONE',  ( 45.31840898497604542, 11.19016079752309167, -3.739202734180806953 ) ) ;
#15000=LINE ( 'NONE', #25004, #22011 ) ;
#15015=ORIENTED_EDGE ( 'NONE', *, *, #17375, .F. ) ;
#15023=CARTESIAN_POINT ( 'NONE',  ( 78.16097076962940093, -5.523138741469189483, 79.26738665229451897 ) ) ;
#15028=ORIENTED_EDGE ( 'NONE', *, *, #13270, .F. ) ;
#15048=CARTESIAN_POINT ( 'NONE',  ( 74.25710670715862705, -0.5585041340025438394, 13.65520570039996429 ) ) ;
#15054=CARTESIAN_POINT ( 'NONE',  ( -12.63929815817735758, -2.946992577399104807, 101.5552643058159248 ) ) ;
#15056=CARTESIAN_POINT ( 'NONE',  ( -35.95057207277420019, -4.776692292720859712, 14.02650114813283366 ) ) ;
#15059=CARTESIAN_POINT ( 'NONE',  ( 81.54161849434414933, -5.935345006353228925, 78.03023866733708758 ) ) ;
#15062=CARTESIAN_POINT ( 'NONE',  ( 21.09785597605719332, -16.43545420775217281, 47.04930799450051637 ) ) ;
#15070=DIRECTION ( 'NONE',  ( -1.000000000000000000, -0.000000000000000000, -3.491481338843133355E-15 ) ) ;
#15072=ORIENTED_EDGE ( 'NONE', *, *, #27431, .F. ) ;
#15087=CARTESIAN_POINT ( 'NONE',  ( 100.3079064823960493, -15.93545420775219945, 47.04930799450134771 ) ) ;
#15088=CARTESIAN_POINT ( 'NONE',  ( -10.01019957330261256, -5.935668773294352718, -13.36321184671484552 ) ) ;
#15092=ORIENTED_EDGE ( 'NONE', *, *, #14464, .F. ) ;
#15093=CARTESIAN_POINT ( 'NONE',  ( 0.6836613156275053171, 11.92558985988973497, 99.90211174246701376 ) ) ;
#15094=TOROIDAL_SURFACE ( 'NONE', #3035, 48.63405236513555963, 2.000000000000000000 ) ;
#15097=CARTESIAN_POINT ( 'NONE',  ( 52.99971320245913375, -5.721341737285090545, 105.3293216028873616 ) ) ;
#15107=CARTESIAN_POINT ( 'NONE',  ( -9.875810886335083083, -5.935708903123432911, 107.5270801035856039 ) ) ;
#15111=DIRECTION ( 'NONE',  ( 0.000000000000000000, 0.000000000000000000, -1.000000000000000000 ) ) ;
#15117=ORIENTED_EDGE ( 'NONE', *, *, #12657, .F. ) ;
#15126=AXIS2_PLACEMENT_3D ( 'NONE', #13361, #23358, #1029 ) ;
#15137=FACE_OUTER_BOUND ( 'NONE', #12741, .T. ) ;
#15147=CARTESIAN_POINT ( 'NONE',  ( 54.61603210001991471, -3.872051342217452508, 102.2906237784674204 ) ) ;
#15151=CARTESIAN_POINT ( 'NONE',  ( 47.34055844982418648, 10.07270486929681752, -3.422361949332906939 ) ) ;
#15159=DIRECTION ( 'NONE',  ( 0.000000000000000000, 0.000000000000000000, 1.000000000000000000 ) ) ;
#15163=ADVANCED_FACE ( 'NONE', ( #17089 ), #29244, .T. ) ;
#15167=CARTESIAN_POINT ( 'NONE',  ( -9.728297238921257417, -5.935454207752202116, 107.4930705127871420 ) ) ;
#15174=CARTESIAN_POINT ( 'NONE',  ( 21.09785597605720042, 11.78014697381582643, -8.546216316978195948 ) ) ;
#15179=CARTESIAN_POINT ( 'NONE',  ( 73.80326597356666696, 0.5083845707908861700, 80.05401455079878303 ) ) ;
#15189=DIRECTION ( 'NONE',  ( 0.000000000000000000, 0.000000000000000000, 1.000000000000000000 ) ) ;
#15208=CARTESIAN_POINT ( 'NONE',  ( -43.86699113690139740, -4.883519073094417351, 52.28371130614638673 ) ) ;
#15210=CARTESIAN_POINT ( 'NONE',  ( -32.65337990276172775, 0.2376265079274789416, 80.17160938599175779 ) ) ;
#15213=CARTESIAN_POINT ( 'NONE',  ( -10.48395140503805756, -5.832427868686518302, 104.6627029599396792 ) ) ;
#15215=CARTESIAN_POINT ( 'NONE',  ( -30.33993856030302894, 8.336148451382289437, 18.87414756954700934 ) ) ;
#15216=CARTESIAN_POINT ( 'NONE',  ( 80.56633024382773556, -5.928581419070738434, 15.83468436991982919 ) ) ;
#15222=LINE ( 'NONE', #19975, #14347 ) ;
#15241=EDGE_LOOP ( 'NONE', ( #23444, #26994 ) ) ;
#15251=CARTESIAN_POINT ( 'NONE',  ( -9.880269303432736905, -5.935454207752200340, -13.45870566634170018 ) ) ;
#15264=ORIENTED_EDGE ( 'NONE', *, *, #7123, .T. ) ;
#15268=EDGE_CURVE ( 'NONE', #26, #6039, #24019, .T. ) ;
#15269=DIRECTION ( 'NONE',  ( 0.000000000000000000, 0.000000000000000000, 1.000000000000000000 ) ) ;
#15273=ORIENTED_EDGE ( 'NONE', *, *, #11386, .T. ) ;
#15285=CARTESIAN_POINT ( 'NONE',  ( 21.09785597605719332, 25.56454579224779877, 47.04930799450051637 ) ) ;
#15286=ORIENTED_EDGE ( 'NONE', *, *, #28012, .T. ) ;
#15288=CARTESIAN_POINT ( 'NONE',  ( -38.65545646816406133, -0.7885532610349046401, 80.71350123316483405 ) ) ;
#15308=CARTESIAN_POINT ( 'NONE',  ( -35.68407394989286985, -5.326758346624735019, 14.55639542095637751 ) ) ;
#15309=DIRECTION ( 'NONE',  ( 1.000000000000000000, 0.000000000000000000, -1.224646799147353207E-16 ) ) ;
#15311=CARTESIAN_POINT ( 'NONE',  ( -39.48078212898874995, -5.935481998376881840, 77.98349214134881890 ) ) ;
#15317=CARTESIAN_POINT ( 'NONE',  ( -9.472371843582571671, 5.388785998227650254, -3.351769630585352377 ) ) ;
#15336=CIRCLE ( 'NONE', #30531, 1.000000000000000888 ) ;
#15341=CARTESIAN_POINT ( 'NONE',  ( -9.943725601011752957, -5.936969727347462644, -13.57595196341301858 ) ) ;
#15344=CARTESIAN_POINT ( 'NONE',  ( 21.09785597605719332, 17.56454579224779877, -1.926157182631158093 ) ) ;
#15347=ORIENTED_EDGE ( 'NONE', *, *, #24297, .T. ) ;
#15350=CARTESIAN_POINT ( 'NONE',  ( -29.27337757263006424, -5.906256089375805374, 15.45647446568822225 ) ) ;
#15357=B_SPLINE_SURFACE_WITH_KNOTS ( 'NONE', 3, 1, ( 
 ( #24342, #28787 ),
 ( #6954, #6469 ),
 ( #1372, #11389 ),
 ( #29275, #24505 ),
 ( #24180, #6789 ),
 ( #16949, #26973 ) ),
 .UNSPECIFIED., .F., .F., .F.,
 ( 4, 1, 1, 4 ),
 ( 2, 2 ),
 ( 0.1800733115436725096, 0.4989925988945991819, 0.7849997004460342875, 1.000000000000000000 ),
 ( 0.000000000000000000, 1.000000000000000000 ),
 .UNSPECIFIED. ) ;
#15360=ORIENTED_EDGE ( 'NONE', *, *, #30020, .F. ) ;
#15362=VECTOR ( 'NONE', #22628, 1000.000000000000000 ) ;
#15365=CARTESIAN_POINT ( 'NONE',  ( -9.875059786958400920, -5.935668157269682332, 107.6366642019984567 ) ) ;
#15367=ORIENTED_EDGE ( 'NONE', *, *, #15849, .F. ) ;
#15377=CARTESIAN_POINT ( 'NONE',  ( -11.87686653301373241, -4.853532562205602474, 103.2493967191210373 ) ) ;
#15379=CARTESIAN_POINT ( 'NONE',  ( -32.97970629999527858, -0.5268592320365600434, 13.64887994798114512 ) ) ;
#15380=CARTESIAN_POINT ( 'NONE',  ( -6.282007179091762872, 9.127627432390735152, -3.410470909561460928 ) ) ;
#15381=ORIENTED_EDGE ( 'NONE', *, *, #15814, .T. ) ;
#15391=ORIENTED_EDGE ( 'NONE', *, *, #18490, .F. ) ;
#15397=EDGE_CURVE ( 'NONE', #27983, #16490, #20570, .T. ) ;
#15398=EDGE_LOOP ( 'NONE', ( #4735, #11940, #15381, #2519 ) ) ;
#15403=AXIS2_PLACEMENT_3D ( 'NONE', #20260, #17963, #30288 ) ;
#15424=ORIENTED_EDGE ( 'NONE', *, *, #30522, .T. ) ;
#15426=CARTESIAN_POINT ( 'NONE',  ( 21.09785597605719332, -6.704410789454799513, 47.04930799450051637 ) ) ;
#15434=AXIS2_PLACEMENT_3D ( 'NONE', #23194, #28286, #5806 ) ;
#15442=CARTESIAN_POINT ( 'NONE',  ( -58.11219453028166981, 25.56454579224780232, 47.04930799450023926 ) ) ;
#15447=CARTESIAN_POINT ( 'NONE',  ( -38.65545646816406133, -5.952175616702188421, 78.54874598263256757 ) ) ;
#15448=DIRECTION ( 'NONE',  ( 3.551608010268815105E-15, 0.000000000000000000, 1.000000000000000000 ) ) ;
#15452=ADVANCED_FACE ( 'NONE', ( #10856 ), #10118, .F. ) ;
#15456=CARTESIAN_POINT ( 'NONE',  ( 52.07598125554711999, -5.935454207752202116, 132.0493079945005377 ) ) ;
#15466=EDGE_LOOP ( 'NONE', ( #16493, #2617, #18514, #14466 ) ) ;
#15467=CARTESIAN_POINT ( 'NONE',  ( -39.52346957204299827, -5.935776016422421364, 77.96988935039777857 ) ) ;
#15471=CARTESIAN_POINT ( 'NONE',  ( 21.09785597605719332, -5.986312001188950127, -20.31486511684154550 ) ) ;
#15478=DIRECTION ( 'NONE',  ( -0.000000000000000000, -0.000000000000000000, 1.000000000000000000 ) ) ;
#15480=VERTEX_POINT ( 'NONE', #25621 ) ;
#15483=EDGE_CURVE ( 'NONE', #32242, #27103, #29492, .T. ) ;
#15498=CARTESIAN_POINT ( 'NONE',  ( 0.6836613156275053171, 11.92558985988973497, -4.944603100128008855 ) ) ;
#15501=CARTESIAN_POINT ( 'NONE',  ( 74.68627032013220912, -1.428409478025942425, 80.66670155429770261 ) ) ;
#15509=DIRECTION ( 'NONE',  ( 0.000000000000000000, 0.000000000000000000, -1.000000000000000000 ) ) ;
#15514=CARTESIAN_POINT ( 'NONE',  ( 54.18094237054272355, -4.708525186292121134, -9.920763639972056680 ) ) ;
#15518=CIRCLE ( 'NONE', #3465, 2.500000000000002220 ) ;
#15522=LINE ( 'NONE', #12756, #14709 ) ;
#15523=EDGE_CURVE ( 'NONE', #30456, #1224, #27394, .T. ) ;
#15532=CARTESIAN_POINT ( 'NONE',  ( -12.19700416223893313, -0.2653311271195798460, 100.0789975867371169 ) ) ;
#15534=DIRECTION ( 'NONE',  ( 0.000000000000000000, 1.000000000000000000, -0.000000000000000000 ) ) ;
#15541=CYLINDRICAL_SURFACE ( 'NONE', #9090, 84.30000000000001137 ) ;
#15546=FACE_OUTER_BOUND ( 'NONE', #957, .T. ) ;
#15548=DIRECTION ( 'NONE',  ( 1.000000000000000000, -0.000000000000000000, -0.000000000000000000 ) ) ;
#15553=AXIS2_PLACEMENT_3D ( 'NONE', #2268, #15070, #28150 ) ;
#15566=ORIENTED_EDGE ( 'NONE', *, *, #20202, .F. ) ;
#15581=ORIENTED_EDGE ( 'NONE', *, *, #7357, .F. ) ;
#15591=DIRECTION ( 'NONE',  ( 0.000000000000000000, 0.000000000000000000, 1.000000000000000000 ) ) ;
#15593=CARTESIAN_POINT ( 'NONE',  ( -44.78404486970123344, -5.108345900017423169, 52.41914759286123626 ) ) ;
#15597=CARTESIAN_POINT ( 'NONE',  ( -29.27613032885505007, -5.952175616702188421, 78.54874598263256757 ) ) ;
#15599=DIRECTION ( 'NONE',  ( 0.000000000000000000, -1.000000000000000000, 0.000000000000000000 ) ) ;
#15600=DIRECTION ( 'NONE',  ( 0.000000000000000000, 1.000000000000000000, 0.000000000000000000 ) ) ;
#15601=EDGE_CURVE ( 'NONE', #10149, #10609, #32331, .T. ) ;
#15602=DIRECTION ( 'NONE',  ( 0.000000000000000000, 0.000000000000000000, -1.000000000000000000 ) ) ;
#15603=CARTESIAN_POINT ( 'NONE',  ( -37.47960991055109758, -5.772969811237893545, 78.78223253563916728 ) ) ;
#15609=B_SPLINE_SURFACE_WITH_KNOTS ( 'NONE', 3, 1, ( 
 ( #24598, #24934 ),
 ( #21808, #27061 ),
 ( #7205, #9513 ),
 ( #4913, #19507 ),
 ( #31826, #421 ),
 ( #31994, #29539 ) ),
 .UNSPECIFIED., .F., .F., .F.,
 ( 4, 1, 1, 4 ),
 ( 2, 2 ),
 ( 0.1800733115436725096, 0.3950736110976382220, 0.6810807126490734387, 1.000000000000000000 ),
 ( 0.000000000000000000, 1.000000000000000000 ),
 .UNSPECIFIED. ) ;
#15613=ORIENTED_EDGE ( 'NONE', *, *, #2846, .T. ) ;
#15620=EDGE_CURVE ( 'NONE', #12130, #17686, #16101, .T. ) ;
#15630=VECTOR ( 'NONE', #12853, 1000.000000000000114 ) ;
#15633=AXIS2_PLACEMENT_3D ( 'NONE', #546, #8109, #5967 ) ;
#15634=ORIENTED_EDGE ( 'NONE', *, *, #31643, .T. ) ;
#15641=ADVANCED_FACE ( 'NONE', ( #25261 ), #19675, .F. ) ;
#15642=CARTESIAN_POINT ( 'NONE',  ( 76.33917176002422877, -3.872051342217440517, 13.53113187053797972 ) ) ;
#15665=CARTESIAN_POINT ( 'NONE',  ( -10.16620058928556780, -5.922252862938464091, -12.36825037132245697 ) ) ;
#15666=DIRECTION ( 'NONE',  ( 0.000000000000000000, 0.000000000000000000, 1.000000000000000000 ) ) ;
#15669=CARTESIAN_POINT ( 'NONE',  ( 54.63929679171693721, -1.094061166256825812, -7.310699946633206103 ) ) ;
#15676=B_SPLINE_CURVE_WITH_KNOTS ( 'NONE', 3,
 ( #6956, #16952, #26976, #27303, #4822, #24507, #2028, #12045, #32072, #9587, #9912, #7455 ),
 .UNSPECIFIED., .F., .F.,
 ( 4, 2, 2, 2, 2, 4 ),
 ( 0.0003422200191418649728, 0.002082436906217386297, 0.003822653793292908001, 0.005562870680368429271, 0.006432979123906190123, 0.007303087567443950975 ),
 .UNSPECIFIED. ) ;
#15677=EDGE_CURVE ( 'NONE', #16051, #30056, #3198, .T. ) ;
#15686=CARTESIAN_POINT ( 'NONE',  ( -10.97410526921440521, -5.983766253076979069, 97.43646483284780402 ) ) ;
#15715=CARTESIAN_POINT ( 'NONE',  ( -9.745345167868416425, 4.618558202237278643, 99.33977322240662033 ) ) ;
#15716=EDGE_CURVE ( 'NONE', #7248, #28192, #19535, .T. ) ;
#15738=CARTESIAN_POINT ( 'NONE',  ( 53.30244988830531838, -5.573920848077356993, 105.0704484403068619 ) ) ;
#15749=DIRECTION ( 'NONE',  ( 0.000000000000000000, -1.000000000000000000, -0.000000000000000000 ) ) ;
#15763=CIRCLE ( 'NONE', #19403, 56.47014401861810029 ) ;
#15765=ORIENTED_EDGE ( 'NONE', *, *, #28038, .T. ) ;
#15772=CARTESIAN_POINT ( 'NONE',  ( 81.51037581727311476, -5.935668773294344724, 15.94125244514089523 ) ) ;
#15790=CARTESIAN_POINT ( 'NONE',  ( 54.49195827015791593, -0.5585041340025316270, 100.2085587256018471 ) ) ;
#15800=CARTESIAN_POINT ( 'NONE',  ( -39.39937829020581006, -5.936106920828554401, 77.94045110924388098 ) ) ;
#15804=AXIS2_PLACEMENT_3D ( 'NONE', #28342, #25713, #5531 ) ;
#15814=EDGE_CURVE ( 'NONE', #3553, #19298, #12219, .T. ) ;
#15817=CARTESIAN_POINT ( 'NONE',  ( 21.09785597605720042, 14.86454579224779771, 95.68336035963606889 ) ) ;
#15833=CARTESIAN_POINT ( 'NONE',  ( -4.902144023942810236, 25.56454579224779877, 49.54930799450078638 ) ) ;
#15836=CARTESIAN_POINT ( 'NONE',  ( -9.947536845470862588, -5.938447472589721166, -12.54648800223589333 ) ) ;
#15839=CARTESIAN_POINT ( 'NONE',  ( 54.78750462725908932, -3.218976025668799146, -8.600583132619711080 ) ) ;
#15849=EDGE_CURVE ( 'NONE', #26, #21967, #13759, .T. ) ;
#15851=CARTESIAN_POINT ( 'NONE',  ( -35.59135993922510721, -5.255974443259752604, 79.62489112376373157 ) ) ;
#15856=ORIENTED_EDGE ( 'NONE', *, *, #30659, .F. ) ;
#15859=CARTESIAN_POINT ( 'NONE',  ( -30.60184210043303921, 11.23625233873419305, 71.15371187152176446 ) ) ;
#15867=ORIENTED_EDGE ( 'NONE', *, *, #2113, .T. ) ;
#15870=DIRECTION ( 'NONE',  ( 3.534951791954965799E-15, 3.759183808608825436E-15, -1.000000000000000000 ) ) ;
#15871=CARTESIAN_POINT ( 'NONE',  ( 21.09785597605719332, -15.72540370141337007, 47.04930799450051637 ) ) ;
#15877=DIRECTION ( 'NONE',  ( 1.000000000000000000, 0.000000000000000000, -1.224646799147353207E-16 ) ) ;
#15886=CARTESIAN_POINT ( 'NONE',  ( -10.56084922076344235, 3.230235421722207345, 99.74989852988510108 ) ) ;
#15894=CARTESIAN_POINT ( 'NONE',  ( 81.70930933238793159, -5.935454207752202116, 77.87546120947918382 ) ) ;
#15906=CARTESIAN_POINT ( 'NONE',  ( 53.89934057735932527, -5.043292969097945111, 104.3954240496316714 ) ) ;
#15921=ORIENTED_EDGE ( 'NONE', *, *, #7538, .T. ) ;
#15924=CARTESIAN_POINT ( 'NONE',  ( -44.85780503240869876, -5.258343014327087062, 52.53743480612791217 ) ) ;
#15925=VERTEX_POINT ( 'NONE', #26385 ) ;
#15945=CARTESIAN_POINT ( 'NONE',  ( 52.33191709358631272, 3.957035103101695928, 98.60043611252098117 ) ) ;
#15948=CARTESIAN_POINT ( 'NONE',  ( 21.09785597605719332, 11.92558985988973497, 47.04930799450051637 ) ) ;
#15951=CARTESIAN_POINT ( 'NONE',  ( -39.39870728729693639, -5.936092197299768891, 77.94355715136961749 ) ) ;
#15963=CARTESIAN_POINT ( 'NONE',  ( 72.33761410512941836, 5.053071141216427975, 16.47634976544295782 ) ) ;
#15969=ADVANCED_FACE ( 'NONE', ( #7169 ), #16927, .T. ) ;
#15974=TOROIDAL_SURFACE ( 'NONE', #17545, 67.99999999999997158, 4.000000000000000000 ) ;
#15985=ORIENTED_EDGE ( 'NONE', *, *, #30320, .T. ) ;
#16000=AXIS2_PLACEMENT_3D ( 'NONE', #1230, #18627, #18782 ) ;
#16005=CARTESIAN_POINT ( 'NONE',  ( -35.00907444222341525, -4.763445661495945060, 80.08276038674898700 ) ) ;
#16011=FACE_OUTER_BOUND ( 'NONE', #916, .T. ) ;
#16016=CARTESIAN_POINT ( 'NONE',  ( -36.90670693849242667, -5.935454207752202116, 16.07118271501078510 ) ) ;
#16017=ORIENTED_EDGE ( 'NONE', *, *, #2806, .T. ) ;
#16031=DIRECTION ( 'NONE',  ( 0.000000000000000000, 0.000000000000000000, -1.000000000000000000 ) ) ;
#16035=CARTESIAN_POINT ( 'NONE',  ( -12.58835873576790121, -1.823725651226728584, 101.7951854207034614 ) ) ;
#16043=DIRECTION ( 'NONE',  ( 0.000000000000000000, 0.000000000000000000, -1.000000000000000000 ) ) ;
#16051=VERTEX_POINT ( 'NONE', #27681 ) ;
#16054=ORIENTED_EDGE ( 'NONE', *, *, #5799, .F. ) ;
#16065=CARTESIAN_POINT ( 'NONE',  ( 21.09785597605719332, 14.86454579224779948, 47.04930799450051637 ) ) ;
#16069=DIRECTION ( 'NONE',  ( 0.000000000000000000, -1.000000000000000000, -0.000000000000000000 ) ) ;
#16073=ORIENTED_EDGE ( 'NONE', *, *, #29076, .T. ) ;
#16075=CIRCLE ( 'NONE', #24467, 67.18681090792816235 ) ;
#16089=FACE_OUTER_BOUND ( 'NONE', #5047, .T. ) ;
#16090=DIRECTION ( 'NONE',  ( 0.000000000000000000, 1.000000000000000000, 0.000000000000000000 ) ) ;
#16094=ORIENTED_EDGE ( 'NONE', *, *, #23271, .T. ) ;
#16097=CARTESIAN_POINT ( 'NONE',  ( 21.09785597605719332, -9.935454207752199451, 47.04930799450051637 ) ) ;
#16098=ORIENTED_EDGE ( 'NONE', *, *, #19053, .T. ) ;
#16101=B_SPLINE_CURVE_WITH_KNOTS ( 'NONE', 3,
 ( #308, #19514, #15088, #17211, #20004, #7548, #30034, #151, #27402, #10170, #15251, #29546 ),
 .UNSPECIFIED., .F., .F.,
 ( 4, 2, 2, 2, 2, 4 ),
 ( 0.0003078418816934435655, 0.0003848023521168015431, 0.0004232825873284805319, 0.0004617628225401594665, 0.0005387232929635211304, 0.0006156837633868826858 ),
 .UNSPECIFIED. ) ;
#16103=CARTESIAN_POINT ( 'NONE',  ( 47.09785597605719687, 24.86454579224779948, 49.54930799450042400 ) ) ;
#16112=EDGE_CURVE ( 'NONE', #1878, #5045, #10667, .T. ) ;
#16123=CARTESIAN_POINT ( 'NONE',  ( -4.902144023942810236, 25.56454579224779877, 47.04930799450078638 ) ) ;
#16126=PRESENTATION_STYLE_ASSIGNMENT (( #6126 ) ) ;
#16134=CARTESIAN_POINT ( 'NONE',  ( 106.0978559760573887, -5.935454207752198563, 77.87546120947926909 ) ) ;
#16143=CARTESIAN_POINT ( 'NONE',  ( 52.75656117287782365, 3.230235421722231326, -5.651282540884040806 ) ) ;
#16152=CIRCLE ( 'NONE', #14064, 67.18681090792816235 ) ;
#16153=CIRCLE ( 'NONE', #9347, 85.00000000000001421 ) ;
#16164=ORIENTED_EDGE ( 'NONE', *, *, #5002, .T. ) ;
#16169=VERTEX_POINT ( 'NONE', #1841 ) ;
#16174=ORIENTED_EDGE ( 'NONE', *, *, #20234, .F. ) ;
#16177=FACE_OUTER_BOUND ( 'NONE', #21362, .T. ) ;
#16179=ORIENTED_EDGE ( 'NONE', *, *, #27387, .T. ) ;
#16193=EDGE_CURVE ( 'NONE', #32110, #7566, #30073, .T. ) ;
#16200=CARTESIAN_POINT ( 'NONE',  ( -4.902144023942810236, 24.86454579224779948, 47.04930799450078638 ) ) ;
#16202=ADVANCED_FACE ( 'NONE', ( #6766 ), #20029, .T. ) ;
#16207=ORIENTED_EDGE ( 'NONE', *, *, #27458, .T. ) ;
#16213=DIRECTION ( 'NONE',  ( 0.000000000000000000, 1.000000000000000000, 0.000000000000000000 ) ) ;
#16215=CARTESIAN_POINT ( 'NONE',  ( -5.148203073178546418, 10.06999148276586808, -4.322672743066429568 ) ) ;
#16227=CARTESIAN_POINT ( 'NONE',  ( 21.09785597605719332, 25.56454579224779877, 18.54930799450050927 ) ) ;
#16236=ORIENTED_EDGE ( 'NONE', *, *, #20814, .F. ) ;
#16249=EDGE_CURVE ( 'NONE', #313, #6650, #10089, .T. ) ;
#16250=DIRECTION ( 'NONE',  ( 1.000000000000000000, 0.000000000000000000, 1.224646799147353207E-16 ) ) ;
#16258=CONICAL_SURFACE ( 'NONE', #27251, 67.36417311134205477, 1.291543646476234874 ) ;
#16261=CARTESIAN_POINT ( 'NONE',  ( -10.27276115262104561, -5.884593569754286158, 106.2621915093639871 ) ) ;
#16281=CONICAL_SURFACE ( 'NONE', #10548, 72.00502525316939284, 0.7853981633974482790 ) ;
#16287=AXIS2_PLACEMENT_3D ( 'NONE', #15344, #8442, #3347 ) ;
#16300=CARTESIAN_POINT ( 'NONE',  ( 21.09785597605719332, 11.92558985988973497, 102.9072182181210451 ) ) ;
#16303=CARTESIAN_POINT ( 'NONE',  ( -44.85737707344571135, -5.257416160756734236, 41.56220475672508741 ) ) ;
#16311=CARTESIAN_POINT ( 'NONE',  ( 73.54853330490307428, 11.86909835304794392, 25.53840420133489175 ) ) ;
#16314=AXIS2_PLACEMENT_3D ( 'NONE', #1924, #20137, #32302 ) ;
#16317=DIRECTION ( 'NONE',  ( 0.000000000000000000, 0.000000000000000000, 1.000000000000000000 ) ) ;
#16318=CARTESIAN_POINT ( 'NONE',  ( -33.51206715926824842, -3.083556648223061192, 80.76191266582368655 ) ) ;
#16319=DIRECTION ( 'NONE',  ( -0.000000000000000000, -1.000000000000000000, -0.000000000000000000 ) ) ;
#16326=CARTESIAN_POINT ( 'NONE',  ( -4.652357239589691495, 10.40257568944043243, 97.56955547902282433 ) ) ;
#16328=DIRECTION ( 'NONE',  ( 0.000000000000000000, 1.000000000000000000, 0.000000000000000000 ) ) ;
#16332=ORIENTED_EDGE ( 'NONE', *, *, #23391, .F. ) ;
#16351=MECHANICAL_DESIGN_GEOMETRIC_PRESENTATION_REPRESENTATION('',(#29488),#9098);
#16354=ORIENTED_EDGE ( 'NONE', *, *, #18490, .T. ) ;
#16376=EDGE_CURVE ( 'NONE', #13273, #12963, #6474, .T. ) ;
#16391=B_SPLINE_CURVE_WITH_KNOTS ( 'NONE', 3,
 ( #32421, #5173, #12564, #7143, #20254, #15341, #32264, #17307, #30281, #22066, #22552, #22389 ),
 .UNSPECIFIED., .F., .F.,
 ( 4, 2, 2, 2, 2, 4 ),
 ( 0.000000000000000000, 7.696047042336268032E-05, 0.0001154407056350440679, 0.0001539209408467254419, 0.0002308814112700844766, 0.0003078418816934435655 ),
 .UNSPECIFIED. ) ;
#16394=VECTOR ( 'NONE', #8670, 1000.000000000000114 ) ;
#16411=AXIS2_PLACEMENT_3D ( 'NONE', #11418, #11587, #26519 ) ;
#16419=LINE ( 'NONE', #10871, #27174 ) ;
#16420=B_SPLINE_CURVE_WITH_KNOTS ( 'NONE', 3,
 ( #17046, #11814, #7986, #12141, #14440, #20440, #24434, #32162, #17981, #24767, #9671, #17370 ),
 .UNSPECIFIED., .F., .F.,
 ( 4, 2, 2, 2, 2, 4 ),
 ( 0.000000000000000000, 7.988424390471597321E-05, 0.0001597684878094319464, 0.0001997106097617916745, 0.0002396527317141514026, 0.0003195369756188888837 ),
 .UNSPECIFIED. ) ;
#16425=CARTESIAN_POINT ( 'NONE',  ( -5.602943079677954685, 9.702389020015065313, -4.315940132965163656 ) ) ;
#16427=AXIS2_PLACEMENT_3D ( 'NONE', #25396, #12448, #5057 ) ;
#16437=CARTESIAN_POINT ( 'NONE',  ( 52.00918302503911406, -5.936918610400973684, -13.64030521451139677 ) ) ;
#16447=CARTESIAN_POINT ( 'NONE',  ( 72.23777473803548332, 5.417291301124342873, 16.70329581060054380 ) ) ;
#16463=CARTESIAN_POINT ( 'NONE',  ( 73.09176707068579049, 11.92558985988973497, 26.63511333407100778 ) ) ;
#16481=CARTESIAN_POINT ( 'NONE',  ( -30.89605511857125464, 11.92558985988973497, 67.46350265493038023 ) ) ;
#16482=CARTESIAN_POINT ( 'NONE',  ( 21.09785597605719332, -16.63545420775219696, 126.2593585008393831 ) ) ;
#16489=CARTESIAN_POINT ( 'NONE',  ( 52.07878664889356912, -5.935345006353229813, -13.39445452378610568 ) ) ;
#16490=VERTEX_POINT ( 'NONE', #8393 ) ;
#16493=ORIENTED_EDGE ( 'NONE', *, *, #27255, .F. ) ;
#16496=FACE_BOUND ( 'NONE', #18793, .T. ) ;
#16501=DIRECTION ( 'NONE',  ( -0.000000000000000000, 1.000000000000000000, -0.000000000000000000 ) ) ;
#16506=ORIENTED_EDGE ( 'NONE', *, *, #15483, .T. ) ;
#16507=CARTESIAN_POINT ( 'NONE',  ( 21.09785597605719332, -16.43042895458278352, -24.95571725866887292 ) ) ;
#16528=CARTESIAN_POINT ( 'NONE',  ( 21.09785597605719332, -15.93545420775219945, 118.3493079945004922 ) ) ;
#16529=MECHANICAL_DESIGN_GEOMETRIC_PRESENTATION_REPRESENTATION('',(#10284),#21775);
#16531=CARTESIAN_POINT ( 'NONE',  ( -39.02270517653035853, 5.305726650763236130, 42.04930799450051637 ) ) ;
#16539=FACE_OUTER_BOUND ( 'NONE', #19305, .T. ) ;
#16542=DIRECTION ( 'NONE',  ( 0.000000000000000000, 0.000000000000000000, 1.000000000000000000 ) ) ;
#16543=DIRECTION ( 'NONE',  ( 0.000000000000000000, -0.000000000000000000, -1.000000000000000000 ) ) ;
#16546=VERTEX_POINT ( 'NONE', #18544 ) ;
#16563=CARTESIAN_POINT ( 'NONE',  ( -35.12632216515690686, 11.92558985988973674, 40.04930799450050216 ) ) ;
#16564=CARTESIAN_POINT ( 'NONE',  ( 75.42722807921533956, -1.035104995754000834, 13.52045531812380474 ) ) ;
#16578=CARTESIAN_POINT ( 'NONE',  ( -9.985300507345989729, -5.931148802125862929, 106.5968259136538023 ) ) ;
#16580=CARTESIAN_POINT ( 'NONE',  ( -11.36318842908626081, -5.379633064793121200, -10.70487703641348354 ) ) ;
#16588=CARTESIAN_POINT ( 'NONE',  ( -35.64882101543633297, 9.925589859889724309, 52.04930799450051637 ) ) ;
#16611=DIRECTION ( 'NONE',  ( -0.000000000000000000, 1.000000000000000000, -0.000000000000000000 ) ) ;
#16612=DIRECTION ( 'NONE',  ( 1.000000000000000000, 0.000000000000000000, 1.224646799147353207E-16 ) ) ;
#16630=ORIENTED_EDGE ( 'NONE', *, *, #31643, .F. ) ;
#16635=CARTESIAN_POINT ( 'NONE',  ( 81.79525877758869967, -5.936960083300406588, 77.94871473493923020 ) ) ;
#16650=FACE_OUTER_BOUND ( 'NONE', #8908, .T. ) ;
#16657=ORIENTED_EDGE ( 'NONE', *, *, #23459, .T. ) ;
#16664=AXIS2_PLACEMENT_3D ( 'NONE', #20560, #25173, #539 ) ;
#16675=DIRECTION ( 'NONE',  ( 0.000000000000000000, -1.000000000000000000, 0.000000000000000000 ) ) ;
#16694=LINE ( 'NONE', #4065, #23754 ) ;
#16699=EDGE_CURVE ( 'NONE', #14290, #17233, #30021, .T. ) ;
#16702=CARTESIAN_POINT ( 'NONE',  ( -29.27337757263006424, 5.786705267067572933, 16.84970013494222840 ) ) ;
#16704=DIRECTION ( 'NONE',  ( 0.000000000000000000, -1.000000000000000000, 0.000000000000000000 ) ) ;
#16717=TOROIDAL_SURFACE ( 'NONE', #14117, 48.63405236513555963, 2.000000000000000000 ) ;
#16720=ORIENTED_EDGE ( 'NONE', *, *, #14234, .T. ) ;
#16722=ORIENTED_EDGE ( 'NONE', *, *, #13315, .T. ) ;
#16739=CARTESIAN_POINT ( 'NONE',  ( -12.00369637303955450, -4.668720686625170480, -9.884046729306300350 ) ) ;
#16748=CARTESIAN_POINT ( 'NONE',  ( 21.09785597605719332, 14.86454579224779771, -1.584744370635042587 ) ) ;
#16751=VERTEX_POINT ( 'NONE', #10180 ) ;
#16769=DIRECTION ( 'NONE',  ( 0.000000000000000000, 0.000000000000000000, -1.000000000000000000 ) ) ;
#16773=( NAMED_UNIT ( * ) PLANE_ANGLE_UNIT ( ) SI_UNIT ( $, .RADIAN. ) );
#16782=ORIENTED_EDGE ( 'NONE', *, *, #15601, .T. ) ;
#16784=LINE ( 'NONE', #18751, #30510 ) ;
#16791=CARTESIAN_POINT ( 'NONE',  ( 21.09785597605719332, 14.86454579224779771, 47.04930799450051637 ) ) ;
#16794=CARTESIAN_POINT ( 'NONE',  ( 73.45468653378273416, 11.83469976691315928, 25.26135771474555369 ) ) ;
#16807=AXIS2_PLACEMENT_3D ( 'NONE', #28102, #16859, #11622 ) ;
#16831=DIRECTION ( 'NONE',  ( 0.000000000000000000, -9.698999007525318993E-17, 1.000000000000000000 ) ) ;
#16844=VERTEX_POINT ( 'NONE', #30530 ) ;
#16848=CARTESIAN_POINT ( 'NONE',  ( 21.09785597605720042, 13.74476430820393347, -8.950692005499485404 ) ) ;
#16855=CARTESIAN_POINT ( 'NONE',  ( -12.29624631804354706, -0.5585041340025408418, -6.109942736600796565 ) ) ;
#16859=DIRECTION ( 'NONE',  ( -0.000000000000000000, -0.000000000000000000, -1.000000000000000000 ) ) ;
#16864=DIRECTION ( 'NONE',  ( 0.000000000000000000, 0.000000000000000000, -1.000000000000000000 ) ) ;
#16873=CARTESIAN_POINT ( 'NONE',  ( 21.09785597605719332, -19.93545420775220123, 132.0493079945005377 ) ) ;
#16892=AXIS2_PLACEMENT_3D ( 'NONE', #7691, #1096, #16031 ) ;
#16909=CARTESIAN_POINT ( 'NONE',  ( -11.10673793619094241, -5.573920848077346335, -10.97183245130580254 ) ) ;
#16913=CYLINDRICAL_SURFACE ( 'NONE', #14196, 2.500000000000002220 ) ;
#16927=CONICAL_SURFACE ( 'NONE', #5427, 54.74424859897010975, 1.291543646475813212 ) ;
#16929=CARTESIAN_POINT ( 'NONE',  ( 49.97900733303978882, 7.511668073839842030, -3.600006413221115587 ) ) ;
#16939=CARTESIAN_POINT ( 'NONE',  ( -30.66771913184581777, 11.92469184102449908, 26.05320424947958458 ) ) ;
#16949=CARTESIAN_POINT ( 'NONE',  ( 52.07598125554711999, -5.935454207752202116, 106.7232700815558957 ) ) ;
#16952=CARTESIAN_POINT ( 'NONE',  ( 71.56946472858759023, 10.07047442526145531, 20.80384636583699987 ) ) ;
#16958=ORIENTED_EDGE ( 'NONE', *, *, #3928, .F. ) ;
#16959=EDGE_CURVE ( 'NONE', #28042, #23355, #22705, .T. ) ;
#16961=EDGE_CURVE ( 'NONE', #9654, #3824, #19487, .T. ) ;
#16982=VERTEX_POINT ( 'NONE', #13771 ) ;
#16983=CARTESIAN_POINT ( 'NONE',  ( -45.06166779280743384, -5.721341737285086992, 53.14897153969102561 ) ) ;
#16994=CONICAL_SURFACE ( 'NONE', #26970, 85.00000000000001421, 0.7853981633974621568 ) ;
#16999=ORIENTED_EDGE ( 'NONE', *, *, #28355, .F. ) ;
#17009=CARTESIAN_POINT ( 'NONE',  ( -10.08218489754580638, -5.944439029104265693, -10.85306528164251993 ) ) ;
#17013=CARTESIAN_POINT ( 'NONE',  ( 52.11354816884804819, -5.936701049740607417, 107.6763359263316602 ) ) ;
#17014=DIRECTION ( 'NONE',  ( 1.000000000000000000, 0.000000000000000000, 0.000000000000000000 ) ) ;
#17019=CARTESIAN_POINT ( 'NONE',  ( -58.11219453028166981, 25.56454579224780232, 47.04930799450023926 ) ) ;
#17021=ADVANCED_FACE ( 'NONE', ( #29341, #11787, #28864, #8829, #14090, #24086 ), #13932, .F. ) ;
#17023=ORIENTED_EDGE ( 'NONE', *, *, #4701, .F. ) ;
#17046=CARTESIAN_POINT ( 'NONE',  ( 51.92400919103563695, -5.935454207752202116, -13.56214536183033381 ) ) ;
#17049=CIRCLE ( 'NONE', #7105, 72.49999999999997158 ) ;
#17052=FACE_OUTER_BOUND ( 'NONE', #7392, .T. ) ;
#17053=CARTESIAN_POINT ( 'NONE',  ( -63.90214402394282445, 9.925589859889722533, 52.04930799450051637 ) ) ;
#17056=CARTESIAN_POINT ( 'NONE',  ( -9.728297238921268075, -5.935454207752198563, 105.1347781458764103 ) ) ;
#17059=DIRECTION ( 'NONE',  ( 1.000000000000000000, -3.756723415560144304E-15, 0.000000000000000000 ) ) ;
#17071=DIRECTION ( 'NONE',  ( 0.000000000000000000, 0.000000000000000000, -1.000000000000000000 ) ) ;
#17089=FACE_OUTER_BOUND ( 'NONE', #23898, .T. ) ;
#17092=CARTESIAN_POINT ( 'NONE',  ( 21.09785597605719332, -16.63545420775219696, -32.16074251183835031 ) ) ;
#17096=PLANE ( 'NONE',  #24645 ) ;
#17102=CARTESIAN_POINT ( 'NONE',  ( -29.72578043774887391, 6.684485874209331158, 17.55139590643513614 ) ) ;
#17106=CARTESIAN_POINT ( 'NONE',  ( -39.56610103014499202, -5.935834405102645484, 77.89388049883636711 ) ) ;
#17109=VERTEX_POINT ( 'NONE', #17179 ) ;
#17119=EDGE_LOOP ( 'NONE', ( #4569, #11284, #6484, #5131 ) ) ;
#17122=CARTESIAN_POINT ( 'NONE',  ( 21.09785597605719332, 15.06454579224778456, 47.04930799450051637 ) ) ;
#17126=CARTESIAN_POINT ( 'NONE',  ( -29.37097840176921792, 10.01373725922364599, 73.36819798580265228 ) ) ;
#17132=CARTESIAN_POINT ( 'NONE',  ( 72.87831073108154101, 11.92558985988973141, 68.00716504909145499 ) ) ;
#17143=FACE_OUTER_BOUND ( 'NONE', #9245, .T. ) ;
#17144=ORIENTED_EDGE ( 'NONE', *, *, #9949, .T. ) ;
#17147=FACE_OUTER_BOUND ( 'NONE', #12328, .T. ) ;
#17152=VERTEX_POINT ( 'NONE', #4555 ) ;
#17153=EDGE_CURVE ( 'NONE', #24330, #2165, #15222, .T. ) ;
#17159=DIRECTION ( 'NONE',  ( 0.000000000000000000, 0.000000000000000000, 1.000000000000000000 ) ) ;
#17162=ORIENTED_EDGE ( 'NONE', *, *, #23572, .T. ) ;
#17163=CARTESIAN_POINT ( 'NONE',  ( 75.92816826855421652, -3.374355247260707014, 13.38734790222314075 ) ) ;
#17171=ORIENTED_EDGE ( 'NONE', *, *, #14465, .F. ) ;
#17177=CARTESIAN_POINT ( 'NONE',  ( 52.17809377605063048, -5.936602078651307401, 107.6389665681752348 ) ) ;
#17179=CARTESIAN_POINT ( 'NONE',  ( -30.88361636257000598, 11.92558985988973141, 67.49515520264003499 ) ) ;
#17188=DIRECTION ( 'NONE',  ( 0.000000000000000000, 1.000000000000000000, 0.000000000000000000 ) ) ;
#17189=CARTESIAN_POINT ( 'NONE',  ( -38.57628410747783221, -3.086620340690746644, 13.27411520529475020 ) ) ;
#17191=ORIENTED_EDGE ( 'NONE', *, *, #10970, .F. ) ;
#17193=ORIENTED_EDGE ( 'NONE', *, *, #30063, .T. ) ;
#17201=LINE ( 'NONE', #4260, #21241 ) ;
#17209=AXIS2_PLACEMENT_3D ( 'NONE', #17848, #30331, #22927 ) ;
#17211=CARTESIAN_POINT ( 'NONE',  ( -9.987729244453721122, -5.936379232154282981, -13.33170860045786910 ) ) ;
#17214=ORIENTED_EDGE ( 'NONE', *, *, #2591, .T. ) ;
#17233=VERTEX_POINT ( 'NONE', #923 ) ;
#17236=EDGE_CURVE ( 'NONE', #20563, #5070, #31120, .T. ) ;
#17246=CARTESIAN_POINT ( 'NONE',  ( -38.34716389643126178, -5.918128512222508242, 15.86828009547534890 ) ) ;
#17261=CARTESIAN_POINT ( 'NONE',  ( 21.09785597605719332, 24.86454579224779948, 70.54930799450050927 ) ) ;
#17264=ORIENTED_EDGE ( 'NONE', *, *, #22238, .F. ) ;
#17272=CARTESIAN_POINT ( 'NONE',  ( 21.09785597605720397, -15.72540370141337007, -24.25069200549945947 ) ) ;
#17276=ORIENTED_EDGE ( 'NONE', *, *, #21922, .T. ) ;
#17279=CARTESIAN_POINT ( 'NONE',  ( -63.90214402394282445, 11.92558985988973497, 26.63511333407100778 ) ) ;
#17282=EDGE_LOOP ( 'NONE', ( #27584, #7002, #31493, #5090 ) ) ;
#17291=VERTEX_POINT ( 'NONE', #5696 ) ;
#17303=CARTESIAN_POINT ( 'NONE',  ( 71.88636670473840695, 11.19016079752308634, 71.26986100341954966 ) ) ;
#17307=CARTESIAN_POINT ( 'NONE',  ( -9.982381823936176346, -5.936602078651308290, -13.54035057917421270 ) ) ;
#17317=ORIENTED_EDGE ( 'NONE', *, *, #25011, .F. ) ;
#17322=AXIS2_PLACEMENT_3D ( 'NONE', #3303, #8831, #5775 ) ;
#17324=DIRECTION ( 'NONE',  ( 0.000000000000000000, -1.000000000000000000, 0.000000000000000000 ) ) ;
#17325=ADVANCED_FACE ( 'NONE', ( #18156 ), #15541, .F. ) ;
#17338=DIRECTION ( 'NONE',  ( 0.000000000000000000, -0.7071067811865426878, -0.7071067811865524577 ) ) ;
#17344=CARTESIAN_POINT ( 'NONE',  ( -10.80400125034478087, -5.721341737285083440, -11.23070561388631816 ) ) ;
#17362=ORIENTED_EDGE ( 'NONE', *, *, #18608, .F. ) ;
#17363=DIRECTION ( 'NONE',  ( 0.000000000000000000, -1.000000000000000000, 0.000000000000000000 ) ) ;
#17365=CIRCLE ( 'NONE', #3210, 85.00000000000001421 ) ;
#17366=TOROIDAL_SURFACE ( 'NONE', #18394, 55.59552431147871232, 0.3000000000000000444 ) ;
#17368=ORIENTED_EDGE ( 'NONE', *, *, #28610, .T. ) ;
#17370=CARTESIAN_POINT ( 'NONE',  ( 52.07598125402753197, -5.935454207809698346, -13.48459002699794063 ) ) ;
#17371=B_SPLINE_CURVE_WITH_KNOTS ( 'NONE', 3,
 ( #30093, #12370, #32059, #2014, #19406, #22357, #25155, #12030, #6943, #27615, #15147, #9897, #29930, #7600, #17601, #22027, #2672, #7106, #30738, #15790, #7929, #13339, #23496, #2826, #13012, #15945, #28112, #690, #5944, #849, #20224, #30575, #10225, #27780, #10717, #30249 ),
 .UNSPECIFIED., .F., .F.,
 ( 4, 2, 2, 2, 2, 2, 2, 2, 2, 2, 2, 2, 2, 2, 2, 2, 2, 4 ),
 ( 0.000000000000000000, 0.0006656200208596437786, 0.001331240041719287557, 0.002662480083438588125, 0.003993720125157888476, 0.004659340146017538868, 0.005324960166877188393, 0.005990580187736837051, 0.006656200208596487443, 0.007987440250315787360, 0.009318680292035086410, 0.01064992033375438546, 0.01331240041719299570, 0.01464364045891230169, 0.01597488050063160941, 0.01863736058407022139, 0.01996860062578953085, 0.02129984066750884725 ),
 .UNSPECIFIED. ) ;
#17375=EDGE_CURVE ( 'NONE', #21481, #14836, #20100, .T. ) ;
#17380=ADVANCED_FACE ( 'NONE', ( #26191 ), #10683, .F. ) ;
#17383=ORIENTED_EDGE ( 'NONE', *, *, #12914, .T. ) ;
#17421=CYLINDRICAL_SURFACE ( 'NONE', #30465, 54.29999999999999716 ) ;
#17427=DIRECTION ( 'NONE',  ( -0.000000000000000000, 1.000000000000000000, -0.000000000000000000 ) ) ;
#17437=CARTESIAN_POINT ( 'NONE',  ( 71.48501281440437083, 9.702389020015065313, 73.75010705023585444 ) ) ;
#17447=B_SPLINE_CURVE_WITH_KNOTS ( 'NONE', 3,
 ( #388, #13046, #2855, #30444, #3338, #20738, #22721, #30923, #3493, #874 ),
 .UNSPECIFIED., .F., .F.,
 ( 4, 2, 2, 2, 4 ),
 ( 0.0006716755660530363079, 0.002413276598758840909, 0.004154877631464645726, 0.005896478664170449677, 0.007638079696876254494 ),
 .UNSPECIFIED. ) ;
#17458=AXIS2_PLACEMENT_3D ( 'NONE', #21441, #11140, #28682 ) ;
#17462=AXIS2_PLACEMENT_3D ( 'NONE', #23766, #10833, #20824 ) ;
#17465=EDGE_CURVE ( 'NONE', #16982, #5110, #3319, .T. ) ;
#17476=CARTESIAN_POINT ( 'NONE',  ( 21.09785597605719332, 25.56454579224779877, 21.04930799450051282 ) ) ;
#17479=CARTESIAN_POINT ( 'NONE',  ( 74.51022843571014675, 1.102830191788943592, 79.80751175580223844 ) ) ;
#17498=B_SPLINE_CURVE_WITH_KNOTS ( 'NONE', 3,
 ( #11739, #17132, #26836, #29630, #6975, #17303, #14696, #2047, #11899, #24863 ),
 .UNSPECIFIED., .F., .F.,
 ( 4, 2, 2, 2, 4 ),
 ( 0.0006731324393516282178, 0.002417216000136556808, 0.004161299560921485723, 0.005905383121706414204, 0.007649466682491342685 ),
 .UNSPECIFIED. ) ;
#17499=B_SPLINE_CURVE_WITH_KNOTS ( 'NONE', 3,
 ( #11150, #16215, #10986, #3748, #18827, #23131, #21132, #8683, #13773, #28866, #18354, #1273 ),
 .UNSPECIFIED., .F., .F.,
 ( 4, 2, 2, 2, 2, 4 ),
 ( 0.0003422370341462293653, 0.002080102550335782494, 0.003817968066525336598, 0.005555833582714891569, 0.006424766340809668838, 0.007293699098904446107 ),
 .UNSPECIFIED. ) ;
#17505=CARTESIAN_POINT ( 'NONE',  ( -44.30175744945091054, -5.935454207752202116, 53.91104711115070813 ) ) ;
#17512=CARTESIAN_POINT ( 'NONE',  ( -33.48165330108982118, -1.516555287492495463, 13.41764155437908457 ) ) ;
#17536=B_SPLINE_CURVE_WITH_KNOTS ( 'NONE', 3,
 ( #2508, #32386, #32230, #19734, #27464, #14994, #10072, #20069, #15151, #25160 ),
 .UNSPECIFIED., .F., .F.,
 ( 4, 2, 2, 2, 4 ),
 ( 0.0006731324393514880305, 0.002417216000136414994, 0.004161299560921341741, 0.005905383121706269355, 0.007649466682491196101 ),
 .UNSPECIFIED. ) ;
#17545=AXIS2_PLACEMENT_3D ( 'NONE', #22676, #24653, #2815 ) ;
#17547=EDGE_LOOP ( 'NONE', ( #14387, #29489, #5788, #11006 ) ) ;
#17550=DIRECTION ( 'NONE',  ( -1.000000000000000000, 0.000000000000000000, 2.775557561562888984E-15 ) ) ;
#17559=ORIENTED_EDGE ( 'NONE', *, *, #32405, .T. ) ;
#17561=CARTESIAN_POINT ( 'NONE',  ( -63.90214402394282445, -5.935454207752205669, 40.04930799450050216 ) ) ;
#17562=ORIENTED_EDGE ( 'NONE', *, *, #16699, .T. ) ;
#17563=CARTESIAN_POINT ( 'NONE',  ( 52.09557426805990588, -5.936215030417558935, 107.4832098830738829 ) ) ;
#17570=EDGE_CURVE ( 'NONE', #8138, #21967, #12259, .T. ) ;
#17576=AXIS2_PLACEMENT_3D ( 'NONE', #13878, #26993, #21397 ) ;
#17580=ORIENTED_EDGE ( 'NONE', *, *, #20490, .T. ) ;
#17586=LINE ( 'NONE', #22504, #23839 ) ;
#17589=DIRECTION ( 'NONE',  ( 0.000000000000000000, 1.000000000000000000, -0.000000000000000000 ) ) ;
#17595=DIRECTION ( 'NONE',  ( 0.000000000000000000, 0.000000000000000000, -1.000000000000000000 ) ) ;
#17598=VECTOR ( 'NONE', #27975, 1000.000000000000000 ) ;
#17600=CARTESIAN_POINT ( 'NONE',  ( -32.01200205328026982, -0.4574755010172156799, 13.68185562056011406 ) ) ;
#17601=CARTESIAN_POINT ( 'NONE',  ( 54.82962069436126029, -2.844921901652548879, 101.4917363106557247 ) ) ;
#17623=ORIENTED_EDGE ( 'NONE', *, *, #5126, .T. ) ;
#17626=CARTESIAN_POINT ( 'NONE',  ( 79.93903702853120308, -5.822320178461996676, 78.65606980742406051 ) ) ;
#17630=ORIENTED_EDGE ( 'NONE', *, *, #22036, .F. ) ;
#17635=CARTESIAN_POINT ( 'NONE',  ( 81.68227850725321559, -5.935454207752203004, 77.87546120947916961 ) ) ;
#17641=ORIENTED_EDGE ( 'NONE', *, *, #9635, .F. ) ;
#17647=DIRECTION ( 'NONE',  ( -0.000000000000000000, 1.000000000000000000, -0.000000000000000000 ) ) ;
#17652=EDGE_CURVE ( 'NONE', #32242, #29171, #14444, .T. ) ;
#17656=EDGE_CURVE ( 'NONE', #14836, #21481, #17049, .T. ) ;
#17659=CARTESIAN_POINT ( 'NONE',  ( -44.15922173408817031, -5.483165097835474455, 52.77548294416367725 ) ) ;
#17666=CARTESIAN_POINT ( 'NONE',  ( -32.37019670470567689, 0.9468387599394830767, 14.21691100150221132 ) ) ;
#17684=ORIENTED_EDGE ( 'NONE', *, *, #2806, .F. ) ;
#17686=VERTEX_POINT ( 'NONE', #14365 ) ;
#17691=VECTOR ( 'NONE', #25014, 1000.000000000000000 ) ;
#17712=DIRECTION ( 'NONE',  ( 0.000000000000000000, 0.000000000000000000, -1.000000000000000000 ) ) ;
#17718=AXIS2_PLACEMENT_3D ( 'NONE', #4132, #11855, #14157 ) ;
#17736=AXIS2_PLACEMENT_3D ( 'NONE', #7758, #28265, #23007 ) ;
#17738=CARTESIAN_POINT ( 'NONE',  ( -38.65545646816406133, -5.935454207752198563, 77.87546120947918382 ) ) ;
#17748=FACE_OUTER_BOUND ( 'NONE', #3022, .T. ) ;
#17750=EDGE_CURVE ( 'NONE', #8773, #1340, #29106, .T. ) ;
#17752=CARTESIAN_POINT ( 'NONE',  ( 45.32239087082389517, 11.18855628041951711, 97.83690911057082928 ) ) ;
#17754=ORIENTED_EDGE ( 'NONE', *, *, #19375, .F. ) ;
#17769=DIRECTION ( 'NONE',  ( -0.000000000000000000, -1.000000000000000000, -0.000000000000000000 ) ) ;
#17771=CARTESIAN_POINT ( 'NONE',  ( -10.96598430569368432, -5.983766253076982622, -3.351769630585352377 ) ) ;
#17780=CARTESIAN_POINT ( 'NONE',  ( 21.09785597605719332, -15.93545420775219945, -29.66074251183834676 ) ) ;
#17782=EDGE_LOOP ( 'NONE', ( #1430, #9958, #20399, #18028 ) ) ;
#17789=ADVANCED_FACE ( 'NONE', ( #18937 ), #12750, .F. ) ;
#17797=CARTESIAN_POINT ( 'NONE',  ( 81.58134094568082162, -5.936631694656539615, 77.91225944795358771 ) ) ;
#17802=CARTESIAN_POINT ( 'NONE',  ( 21.09785597605719332, -8.874820941924726370, -20.33845821050190494 ) ) ;
#17805=CARTESIAN_POINT ( 'NONE',  ( 21.09785597605719332, -15.93545420775219945, 47.04930799450051637 ) ) ;
#17812=AXIS2_PLACEMENT_3D ( 'NONE', #1367, #11383, #21868 ) ;
#17821=AXIS2_PLACEMENT_3D ( 'NONE', #3656, #24164, #16769 ) ;
#17824=CARTESIAN_POINT ( 'NONE',  ( -43.62245103011230185, -4.418230934988281788, 52.10459351193185285 ) ) ;
#17833=CARTESIAN_POINT ( 'NONE',  ( 80.35715816181534876, -5.900224301042253927, 15.64986376169293791 ) ) ;
#17836=CONICAL_SURFACE ( 'NONE', #23059, 85.00000000000001421, 0.7853981633974621568 ) ;
#17838=CARTESIAN_POINT ( 'NONE',  ( -35.51959509086647415, 11.47739873925888077, 52.78069526241495879 ) ) ;
#17845=EDGE_LOOP ( 'NONE', ( #24202, #25484, #5298, #8580 ) ) ;
#17846=AXIS2_PLACEMENT_3D ( 'NONE', #11417, #16501, #8956 ) ;
#17848=CARTESIAN_POINT ( 'NONE',  ( 100.3079064823960493, 25.56454579224780232, 47.04930799450134771 ) ) ;
#17851=DIRECTION ( 'NONE',  ( 1.000000000000000000, 0.000000000000000000, -1.110223024625154963E-14 ) ) ;
#17862=EDGE_CURVE ( 'NONE', #2614, #2467, #30439, .T. ) ;
#17887=CYLINDRICAL_SURFACE ( 'NONE', #1907, 85.00000000000001421 ) ;
#17889=CARTESIAN_POINT ( 'NONE',  ( 52.13393605659406660, -5.936921830459686689, 107.4316605894145624 ) ) ;
#17893=CARTESIAN_POINT ( 'NONE',  ( 21.09785597605719332, 25.56454579224779877, 47.04930799450051637 ) ) ;
#17897=CARTESIAN_POINT ( 'NONE',  ( -30.60166825031904025, 11.23651971625239021, 22.94476225488443433 ) ) ;
#17912=CARTESIAN_POINT ( 'NONE',  ( 21.09785597605719332, -16.43545420775217281, 47.04930799450051637 ) ) ;
#17913=FACE_OUTER_BOUND ( 'NONE', #4487, .T. ) ;
#17918=CARTESIAN_POINT ( 'NONE',  ( 21.09785597605719332, 12.26495659406217342, 47.04930799450051637 ) ) ;
#17921=DIRECTION ( 'NONE',  ( -0.000000000000000000, -1.000000000000000000, -0.000000000000000000 ) ) ;
#17924=CARTESIAN_POINT ( 'NONE',  ( -32.94875189376105595, -2.247009719175835141, 13.30861947577388271 ) ) ;
#17926=EDGE_LOOP ( 'NONE', ( #2563, #31953, #6963, #16630 ) ) ;
#17928=CARTESIAN_POINT ( 'NONE',  ( 21.09785597605719332, 12.11061942510878886, -8.482108500610603841 ) ) ;
#17935=CARTESIAN_POINT ( 'NONE',  ( -39.40299142976220281, -5.935884043940212962, 77.96317429586483172 ) ) ;
#17939=EDGE_LOOP ( 'NONE', ( #23939, #28005, #28076, #8661, #11307, #16073, #3318, #5930, #9436, #30205, #2999, #24425 ) ) ;
#17943=ORIENTED_EDGE ( 'NONE', *, *, #11046, .T. ) ;
#17952=VECTOR ( 'NONE', #15548, 1000.000000000000000 ) ;
#17954=CARTESIAN_POINT ( 'NONE',  ( 21.09785597605719332, -6.659195188345857552, -20.12191896776992905 ) ) ;
#17959=CARTESIAN_POINT ( 'NONE',  ( -43.35833523721898075, -3.935454207752190126, 42.04930799450051637 ) ) ;
#17963=DIRECTION ( 'NONE',  ( -0.000000000000000000, -1.000000000000000000, -0.000000000000000000 ) ) ;
#17966=CARTESIAN_POINT ( 'NONE',  ( 21.09785597605720042, 12.06852548259731961, 102.7275235127243320 ) ) ;
#17973=AXIS2_PLACEMENT_3D ( 'NONE', #6085, #15600, #28414 ) ;
#17981=CARTESIAN_POINT ( 'NONE',  ( 52.04314975454045111, -5.936463391119990440, -13.39944846985862981 ) ) ;
#17983=CARTESIAN_POINT ( 'NONE',  ( 81.72575882806418690, -5.935454207752202116, 16.07118271501079576 ) ) ;
#17989=CARTESIAN_POINT ( 'NONE',  ( -32.97738962991574851, -0.5062580946980150820, 80.43174492715770896 ) ) ;
#17992=ORIENTED_EDGE ( 'NONE', *, *, #6408, .T. ) ;
#17996=FACE_OUTER_BOUND ( 'NONE', #1299, .T. ) ;
#17999=CARTESIAN_POINT ( 'NONE',  ( 81.65768700022189819, -5.935454207752202116, 16.07118271501079931 ) ) ;
#18003=CIRCLE ( 'NONE', #2280, 19.99999999999999645 ) ;
#18008=ORIENTED_EDGE ( 'NONE', *, *, #32352, .T. ) ;
#18019=CONICAL_SURFACE ( 'NONE', #27992, 67.17122696227043832, 1.291543646476234874 ) ;
#18021=DIRECTION ( 'NONE',  ( -0.000000000000000000, 1.000000000000000000, -0.000000000000000000 ) ) ;
#18028=ORIENTED_EDGE ( 'NONE', *, *, #370, .F. ) ;
#18033=CARTESIAN_POINT ( 'NONE',  ( 48.43849231507899589, 9.162376348828955130, 98.41682639182559456 ) ) ;
#18043=EDGE_CURVE ( 'NONE', #29979, #22618, #32200, .T. ) ;
#18045=EDGE_CURVE ( 'NONE', #5045, #8696, #25661, .T. ) ;
#18050=LINE ( 'NONE', #7892, #2013 ) ;
#18053=ADVANCED_FACE ( 'NONE', ( #27971 ), #4430, .F. ) ;
#18055=AXIS2_PLACEMENT_3D ( 'NONE', #18537, #30717, #15448 ) ;
#18094=CARTESIAN_POINT ( 'NONE',  ( -39.45284321493671342, -5.935743718174008698, 77.88873351080283669 ) ) ;
#18101=LINE ( 'NONE', #10405, #28543 ) ;
#18102=LINE ( 'NONE', #26301, #21903 ) ;
#18109=CARTESIAN_POINT ( 'NONE',  ( 79.67628629021933762, -5.773219817368594242, 78.78228565784779391 ) ) ;
#18119=EDGE_CURVE ( 'NONE', #9364, #5905, #6514, .T. ) ;
#18120=EDGE_CURVE ( 'NONE', #29942, #26412, #26499, .T. ) ;
#18127=CARTESIAN_POINT ( 'NONE',  ( -10.58731244131463178, -5.819500620027731941, -11.73843591528525110 ) ) ;
#18128=LINE ( 'NONE', #3185, #12575 ) ;
#18130=CARTESIAN_POINT ( 'NONE',  ( 54.82722624670270051, -2.181906231262848106, -7.903189434301322258 ) ) ;
#18138=CARTESIAN_POINT ( 'NONE',  ( 100.3079064823960493, 25.56454579224780232, 47.04930799450134771 ) ) ;
#18141=EDGE_LOOP ( 'NONE', ( #13317, #10282, #9044, #7476 ) ) ;
#18142=DIRECTION ( 'NONE',  ( 0.000000000000000000, 0.000000000000000000, -1.000000000000000000 ) ) ;
#18143=LINE ( 'NONE', #10624, #20150 ) ;
#18144=CARTESIAN_POINT ( 'NONE',  ( -32.18821136934754179, 1.455588635105943274, 79.63912307355188602 ) ) ;
#18147=CARTESIAN_POINT ( 'NONE',  ( -11.39532592801639410, -5.321843574075690420, 103.8276984696742034 ) ) ;
#18149=DIRECTION ( 'NONE',  ( -0.000000000000000000, 1.000000000000000000, -0.000000000000000000 ) ) ;
#18150=PRODUCT_DEFINITION_FORMATION_WITH_SPECIFIED_SOURCE ( 'ANY', '', #13281, .NOT_KNOWN. ) ;
#18154=CARTESIAN_POINT ( 'NONE',  ( -35.76183559804942291, 11.10708444000149342, 52.41472866846790168 ) ) ;
#18156=FACE_OUTER_BOUND ( 'NONE', #4814, .T. ) ;
#18171=CARTESIAN_POINT ( 'NONE',  ( -11.98039162717269868, 0.3723237022605148661, 100.7399880312177345 ) ) ;
#18173=VECTOR ( 'NONE', #20588, 1000.000000000000000 ) ;
#18174=ORIENTED_EDGE ( 'NONE', *, *, #30320, .F. ) ;
#18183=ORIENTED_EDGE ( 'NONE', *, *, #11893, .F. ) ;
#18186=CARTESIAN_POINT ( 'NONE',  ( 41.51205063648687599, 11.92558985988973497, 99.90211174246701376 ) ) ;
#18187=CARTESIAN_POINT ( 'NONE',  ( 51.51172421616634978, 5.323792735596120096, 99.13876058871011310 ) ) ;
#18189=EDGE_CURVE ( 'NONE', #3078, #21280, #19060, .T. ) ;
#18197=CARTESIAN_POINT ( 'NONE',  ( 21.09785597605719332, 13.06454579224779877, 47.04930799450051637 ) ) ;
#18200=ORIENTED_EDGE ( 'NONE', *, *, #23422, .F. ) ;
#18203=ORIENTED_EDGE ( 'NONE', *, *, #7573, .F. ) ;
#18205=VERTEX_POINT ( 'NONE', #21692 ) ;
#18206=VERTEX_POINT ( 'NONE', #31719 ) ;
#18208=ADVANCED_FACE ( 'NONE', ( #29246, #4466 ), #22833, .T. ) ;
#18209=CIRCLE ( 'NONE', #22947, 2.500000000000002220 ) ;
#18210=CARTESIAN_POINT ( 'NONE',  ( 21.09785597605719332, 25.56454579224779877, 6.862164259567697933 ) ) ;
#18211=DIRECTION ( 'NONE',  ( 0.000000000000000000, 0.000000000000000000, 1.000000000000000000 ) ) ;
#18213=AXIS2_PLACEMENT_3D ( 'NONE', #12127, #31661, #14099 ) ;
#18214=ORIENTED_EDGE ( 'NONE', *, *, #4492, .T. ) ;
#18219=CYLINDRICAL_SURFACE ( 'NONE', #25405, 2.500000000000002220 ) ;
#18224=B_SPLINE_SURFACE_WITH_KNOTS ( 'NONE', 3, 1, ( 
 ( #3209, #6009 ),
 ( #10623, #15686 ),
 ( #595, #426 ),
 ( #28008, #13080 ),
 ( #23400, #8470 ),
 ( #13405, #10782 ) ),
 .UNSPECIFIED., .F., .F., .F.,
 ( 4, 1, 1, 4 ),
 ( 2, 2 ),
 ( 0.1800733115436725096, 0.3950736110976382220, 0.6810807126490734387, 1.000000000000000000 ),
 ( 0.000000000000000000, 1.000000000000000000 ),
 .UNSPECIFIED. ) ;
#18227=EDGE_CURVE ( 'NONE', #24923, #23976, #24936, .T. ) ;
#18237=DIRECTION ( 'NONE',  ( 0.000000000000000000, 0.000000000000000000, -1.000000000000000000 ) ) ;
#18241=CARTESIAN_POINT ( 'NONE',  ( -35.36827084435264368, 10.42249571538224906, 52.09578328476275288 ) ) ;
#18243=VECTOR ( 'NONE', #24714, 1000.000000000000000 ) ;
#18246=CIRCLE ( 'NONE', #21380, 2.500000000000002220 ) ;
#18254=FACE_OUTER_BOUND ( 'NONE', #20674, .T. ) ;
#18257=TOROIDAL_SURFACE ( 'NONE', #4120, 55.59552431147871232, 0.3000000000000000444 ) ;
#18258=EDGE_LOOP ( 'NONE', ( #3724, #24989 ) ) ;
#18265=CARTESIAN_POINT ( 'NONE',  ( -0.6890700258440008996, 11.83483724345209787, -4.439927286363037240 ) ) ;
#18266=( LENGTH_UNIT ( ) NAMED_UNIT ( * ) SI_UNIT ( .MILLI., .METRE. ) );
#18282=CARTESIAN_POINT ( 'NONE',  ( 53.85605973735868446, 1.102830191789100578, -6.363064465152523219 ) ) ;
#18288=VECTOR ( 'NONE', #26000, 1000.000000000000000 ) ;
#18301=DIRECTION ( 'NONE',  ( 0.000000000000000000, 0.000000000000000000, -1.000000000000000000 ) ) ;
#18303=CARTESIAN_POINT ( 'NONE',  ( -30.33793827003903232, 10.49391138527215084, 72.64809877684305661 ) ) ;
#18308=DIRECTION ( 'NONE',  ( 0.000000000000000000, 0.000000000000000000, 1.000000000000000000 ) ) ;
#18314=CARTESIAN_POINT ( 'NONE',  ( -36.17180646779264919, 10.42241829745360526, 52.09577041703580846 ) ) ;
#18325=CARTESIAN_POINT ( 'NONE',  ( -9.880269303432738681, -5.935454207752202116, -13.32263710021335612 ) ) ;
#18336=EDGE_CURVE ( 'NONE', #3463, #253, #6089, .T. ) ;
#18341=ORIENTED_EDGE ( 'NONE', *, *, #13179, .F. ) ;
#18345=DIRECTION ( 'NONE',  ( 0.000000000000000000, 0.000000000000000000, 1.000000000000000000 ) ) ;
#18354=CARTESIAN_POINT ( 'NONE',  ( 0.4108105365410483212, 11.92558985988973497, -5.698108176600966246 ) ) ;
#18359=CARTESIAN_POINT ( 'NONE',  ( -9.847437802426064479, -5.936463391119989552, 107.4980644588596874 ) ) ;
#18372=ADVANCED_FACE ( 'NONE', ( #677 ), #8552, .T. ) ;
#18381=EDGE_LOOP ( 'NONE', ( #32134, #17171 ) ) ;
#18383=CARTESIAN_POINT ( 'NONE',  ( 21.09785597605719687, 16.33322284159648063, 94.44875166441873660 ) ) ;
#18387=ORIENTED_EDGE ( 'NONE', *, *, #16112, .F. ) ;
#18394=AXIS2_PLACEMENT_3D ( 'NONE', #26997, #27645, #12232 ) ;
#18400=B_SPLINE_CURVE_WITH_KNOTS ( 'NONE', 3,
 ( #10360, #12833, #5922, #828, #27755, #15593, #15924, #25929, #3446, #20354, #27921, #5438 ),
 .UNSPECIFIED., .F., .F.,
 ( 4, 2, 2, 2, 2, 4 ),
 ( 0.0002033792717032385539, 0.0008000624350769520434, 0.001396745598450665560, 0.001993428761824378968, 0.002291770343511237949, 0.002590111925198097364 ),
 .UNSPECIFIED. ) ;
#18407=ADVANCED_FACE ( 'NONE', ( #8391 ), #30393, .F. ) ;
#18422=CARTESIAN_POINT ( 'NONE',  ( 72.97689775927815958, 2.854128177266946675, 15.17817617591508395 ) ) ;
#18425=CARTESIAN_POINT ( 'NONE',  ( 46.86318297022563684, 10.39302479005550062, 97.56778208447272505 ) ) ;
#18428=CARTESIAN_POINT ( 'NONE',  ( 0.4110235620567528891, 11.92558985988973497, -4.837558254760519816 ) ) ;
#18429=ORIENTED_EDGE ( 'NONE', *, *, #19745, .T. ) ;
#18433=ADVANCED_FACE ( 'NONE', ( #16089 ), #16994, .T. ) ;
#18457=EDGE_CURVE ( 'NONE', #1878, #13269, #5829, .T. ) ;
#18459=AXIS2_PLACEMENT_3D ( 'NONE', #14913, #19989, #17851 ) ;
#18466=CARTESIAN_POINT ( 'NONE',  ( 21.09785597605719332, 12.11061942510878886, 47.04930799450051637 ) ) ;
#18468=CARTESIAN_POINT ( 'NONE',  ( -33.88509152296665405, -2.225152678231165027, 80.77477800364387406 ) ) ;
#18469=EDGE_CURVE ( 'NONE', #17152, #3515, #7612, .T. ) ;
#18470=CARTESIAN_POINT ( 'NONE',  ( 21.09785597605719332, -9.935454207752199451, 119.0493079945005093 ) ) ;
#18483=CARTESIAN_POINT ( 'NONE',  ( 21.09785597605719332, 24.86454579224779948, 18.54930799450050927 ) ) ;
#18485=AXIS2_PLACEMENT_3D ( 'NONE', #5766, #22989, #20533 ) ;
#18486=VERTEX_POINT ( 'NONE', #2083 ) ;
#18490=EDGE_CURVE ( 'NONE', #14332, #9808, #23647, .T. ) ;
#18500=ORIENTED_EDGE ( 'NONE', *, *, #27912, .T. ) ;
#18507=ORIENTED_EDGE ( 'NONE', *, *, #22444, .F. ) ;
#18511=CARTESIAN_POINT ( 'NONE',  ( 53.12892922725793454, 2.565965067347319550, 99.95503537435618568 ) ) ;
#18514=ORIENTED_EDGE ( 'NONE', *, *, #8844, .T. ) ;
#18516=CARTESIAN_POINT ( 'NONE',  ( -36.75957860043340020, -5.923061377617729661, 15.81027635050077151 ) ) ;
#18531=AXIS2_PLACEMENT_3D ( 'NONE', #19602, #29633, #14531 ) ;
#18537=CARTESIAN_POINT ( 'NONE',  ( 21.09785597605719332, 11.92558985988973497, 47.04930799450051637 ) ) ;
#18542=CARTESIAN_POINT ( 'NONE',  ( 21.09785597605719332, -15.93545420775219945, 47.04930799450051637 ) ) ;
#18543=CARTESIAN_POINT ( 'NONE',  ( 21.09785597605719332, -15.43545420775221366, 47.04930799450051637 ) ) ;
#18544=CARTESIAN_POINT ( 'NONE',  ( -45.06166779280744095, -5.721341737285086992, 40.94964444931001424 ) ) ;
#18570=CARTESIAN_POINT ( 'NONE',  ( 52.07598125402753197, -5.935454207809698346, -13.48459002699794063 ) ) ;
#18572=DIRECTION ( 'NONE',  ( 0.000000000000000000, 0.000000000000000000, -1.000000000000000000 ) ) ;
#18581=FACE_OUTER_BOUND ( 'NONE', #13656, .T. ) ;
#18583=CARTESIAN_POINT ( 'NONE',  ( 0.6836613156275018754, 1.925589859889728972, 132.0493079945005377 ) ) ;
#18584=AXIS2_PLACEMENT_3D ( 'NONE', #26917, #14456, #11180 ) ;
#18585=SURFACE_STYLE_FILL_AREA ( #8592 ) ;
#18589=CIRCLE ( 'NONE', #10256, 2.500000000000002220 ) ;
#18594=DIRECTION ( 'NONE',  ( 0.000000000000000000, 0.000000000000000000, -1.000000000000000000 ) ) ;
#18597=ORIENTED_EDGE ( 'NONE', *, *, #23459, .F. ) ;
#18602=CARTESIAN_POINT ( 'NONE',  ( 48.43975086764982052, 9.161285963347379990, -4.318226157935770360 ) ) ;
#18604=CARTESIAN_POINT ( 'NONE',  ( 73.95065972402376531, 11.92558985988973497, 26.63511333407101134 ) ) ;
#18608=EDGE_CURVE ( 'NONE', #3824, #1215, #2685, .T. ) ;
#18610=CIRCLE ( 'NONE', #31193, 55.67821551822382276 ) ;
#18615=CARTESIAN_POINT ( 'NONE',  ( -34.05102927978326477, -3.766592597147156773, 80.60727270474869499 ) ) ;
#18620=ORIENTED_EDGE ( 'NONE', *, *, #12588, .T. ) ;
#18624=DIRECTION ( 'NONE',  ( -1.000000000000000000, -0.000000000000000000, -0.000000000000000000 ) ) ;
#18627=DIRECTION ( 'NONE',  ( -0.000000000000000000, 1.000000000000000000, -0.000000000000000000 ) ) ;
#18629=CARTESIAN_POINT ( 'NONE',  ( 21.09785597605719332, 13.74476430820393347, 47.04930799450051637 ) ) ;
#18632=LINE ( 'NONE', #28979, #19480 ) ;
#18641=CARTESIAN_POINT ( 'NONE',  ( -44.31642079201742490, -5.935454207752207445, 40.32453457621193849 ) ) ;
#18657=EDGE_LOOP ( 'NONE', ( #25884, #8891 ) ) ;
#18660=DIRECTION ( 'NONE',  ( 0.000000000000000000, 0.000000000000000000, -1.000000000000000000 ) ) ;
#18665=CYLINDRICAL_SURFACE ( 'NONE', #13272, 2.500000000000002220 ) ;
#18674=ORIENTED_EDGE ( 'NONE', *, *, #26083, .T. ) ;
#18683=DIRECTION ( 'NONE',  ( 0.000000000000000000, 1.000000000000000000, 0.000000000000000000 ) ) ;
#18685=AXIS2_PLACEMENT_3D ( 'NONE', #8523, #3587, #26067 ) ;
#18690=CARTESIAN_POINT ( 'NONE',  ( 21.09785597605720042, -6.314304012688826795, 113.0177564892293987 ) ) ;
#18695=CARTESIAN_POINT ( 'NONE',  ( -35.23450526646055891, 11.85135420694099651, 40.60670944852148523 ) ) ;
#18701=CARTESIAN_POINT ( 'NONE',  ( 21.09785597605720042, 13.74476430820393347, -8.950692005499485404 ) ) ;
#18715=CARTESIAN_POINT ( 'NONE',  ( 21.09785597605720042, 13.74476430820393347, -7.950692005499485404 ) ) ;
#18719=ORIENTED_EDGE ( 'NONE', *, *, #13062, .T. ) ;
#18729=EDGE_CURVE ( 'NONE', #24958, #27541, #23884, .T. ) ;
#18730=EDGE_CURVE ( 'NONE', #16546, #30985, #31729, .T. ) ;
#18734=FACE_BOUND ( 'NONE', #11808, .T. ) ;
#18740=ORIENTED_EDGE ( 'NONE', *, *, #6625, .F. ) ;
#18751=CARTESIAN_POINT ( 'NONE',  ( 106.0978559760575735, 11.92558985988973497, 26.63511333407112858 ) ) ;
#18754=VERTEX_POINT ( 'NONE', #16016 ) ;
#18757=LINE ( 'NONE', #21874, #25154 ) ;
#18758=DIRECTION ( 'NONE',  ( -0.000000000000000000, 1.000000000000000000, -0.000000000000000000 ) ) ;
#18762=ADVANCED_FACE ( 'NONE', ( #20934 ), #6165, .F. ) ;
#18763=ORIENTED_EDGE ( 'NONE', *, *, #17236, .T. ) ;
#18772=CARTESIAN_POINT ( 'NONE',  ( 81.68521218355431301, -5.935668157269678780, 78.02222375751645700 ) ) ;
#18774=ORIENTED_EDGE ( 'NONE', *, *, #6044, .T. ) ;
#18777=ORIENTED_EDGE ( 'NONE', *, *, #28366, .F. ) ;
#18779=DIRECTION ( 'NONE',  ( 0.000000000000000000, 0.000000000000000000, 1.000000000000000000 ) ) ;
#18782=DIRECTION ( 'NONE',  ( 0.000000000000000000, 0.000000000000000000, 1.000000000000000000 ) ) ;
#18783=CARTESIAN_POINT ( 'NONE',  ( 21.09785597605719332, 24.74924423484549507, 7.113493622051541010 ) ) ;
#18793=EDGE_LOOP ( 'NONE', ( #14459, #11092 ) ) ;
#18794=CARTESIAN_POINT ( 'NONE',  ( -44.02797724526854495, -5.204561149836106182, 41.60063710421776051 ) ) ;
#18795=B_SPLINE_CURVE_WITH_KNOTS ( 'NONE', 3,
 ( #7641, #17635, #10268, #7796, #17797, #27821, #25353, #30451, #9077, #6458, #31407, #6291 ),
 .UNSPECIFIED., .F., .F.,
 ( 4, 2, 2, 2, 2, 4 ),
 ( 0.000000000000000000, 7.988424390431281264E-05, 0.0001597684878086256253, 0.0001997106097607669680, 0.0002396527317129083649, 0.0003195369756171903726 ),
 .UNSPECIFIED. ) ;
#18827=CARTESIAN_POINT ( 'NONE',  ( -3.128431330128486287, 11.18784031540631574, -4.623178182644472223 ) ) ;
#18844=AXIS2_PLACEMENT_3D ( 'NONE', #1038, #12891, #11064 ) ;
#18851=AXIS2_PLACEMENT_3D ( 'NONE', #30324, #28348, #15870 ) ;
#18861=ORIENTED_EDGE ( 'NONE', *, *, #14465, .T. ) ;
#18864=VERTEX_POINT ( 'NONE', #9773 ) ;
#18891=CARTESIAN_POINT ( 'NONE',  ( 52.05217022815784844, -5.936245040125577077, -13.58841950574782587 ) ) ;
#18910=CONICAL_SURFACE ( 'NONE', #1632, 55.00000000000000000, 0.7853981633974552734 ) ;
#18928=CLOSED_SHELL ( 'NONE', ( #27878, #12504, #5547, #30912, #14199, #1509, #21838, #25613, #9339, #28752, #8346, #19374, #6667, #15452, #31101, #12227, #857, #32278, #17380, #8197, #28204, #5952, #21469, #13357, #14435, #14126, #5858, #30443, #24884, #4177, #16202, #15969, #4040, #10690, #9910, #8676, #18372, #24686, #9456, #669, #27801, #15163, #7080, #5968, #10171, #19934, #18208, #13103, #1893, #10872, #12584, #8927, #18433, #7210, #24512, #4442, #9672, #17021, #4969, #892, #13489, #18762, #32171, #17325, #18053, #24270, #3026, #10054, #25172, #11002, #9829, #4740, #11759, #29394, #24428, #27670, #22904, #1115, #1, #19828, #29271, #27021, #22613, #20798, #9041, #13986, #31492, #7816, #10613, #30687, #17789, #24292, #12052, #23529, #31258, #24520, #1791, #32029, #1175, #22154, #26207, #12877, #20233, #24829, #14805, #22590, #25262, #10354, #24025, #14989, #13540, #30028, #31786, #30827, #22783, #18407, #20117, #15641, #11234, #6219, #30220, #22404 ) ) ;
#18937=FACE_OUTER_BOUND ( 'NONE', #6890, .T. ) ;
#18940=CARTESIAN_POINT ( 'NONE',  ( 21.09785597605719332, -5.935454207752083988, -20.13750291342764598 ) ) ;
#18941=AXIS2_PLACEMENT_3D ( 'NONE', #22522, #27463, #7109 ) ;
#18946=CARTESIAN_POINT ( 'NONE',  ( 100.3079064823960493, -16.63545420775219696, 44.54930799450134771 ) ) ;
#18960=EDGE_CURVE ( 'NONE', #5905, #9364, #18610, .T. ) ;
#18965=ORIENTED_EDGE ( 'NONE', *, *, #19053, .F. ) ;
#18967=EDGE_CURVE ( 'NONE', #18206, #31078, #31226, .T. ) ;
#18983=DIRECTION ( 'NONE',  ( 0.000000000000000000, 0.000000000000000000, -1.000000000000000000 ) ) ;
#18989=DIRECTION ( 'NONE',  ( -0.000000000000000000, 1.000000000000000000, -0.000000000000000000 ) ) ;
#19000=LINE ( 'NONE', #29031, #23187 ) ;
#19021=CARTESIAN_POINT ( 'NONE',  ( 72.84673228687861979, 6.668192824305379851, 17.53718116896199675 ) ) ;
#19034=CARTESIAN_POINT ( 'NONE',  ( 21.09785597605720397, -16.72540370141334520, -37.25069200549950210 ) ) ;
#19036=CARTESIAN_POINT ( 'NONE',  ( -9.728297238921268075, -5.935454207752198563, 106.7470117857220373 ) ) ;
#19039=CARTESIAN_POINT ( 'NONE',  ( -7.926226286961589373, 7.326690775934350697, -4.556490565496920553 ) ) ;
#19046=CARTESIAN_POINT ( 'NONE',  ( 21.09785597605719332, -6.704410789454799513, -20.27960450816445359 ) ) ;
#19050=CARTESIAN_POINT ( 'NONE',  ( 21.09785597605719332, -15.93545420775219945, 47.04930799450051637 ) ) ;
#19053=EDGE_CURVE ( 'NONE', #5246, #8335, #7318, .T. ) ;
#19060=LINE ( 'NONE', #6608, #24869 ) ;
#19062=DIRECTION ( 'NONE',  ( 0.000000000000000000, -1.000000000000000000, 0.000000000000000000 ) ) ;
#19074=CARTESIAN_POINT ( 'NONE',  ( -39.55421745345908846, -5.936056828695301490, 77.94890933298111690 ) ) ;
#19075=DIRECTION ( 'NONE',  ( 0.000000000000000000, 0.000000000000000000, -1.000000000000000000 ) ) ;
#19093=CARTESIAN_POINT ( 'NONE',  ( -29.41290960217035533, 10.34548297403109807, 72.88772139469026001 ) ) ;
#19095=CARTESIAN_POINT ( 'NONE',  ( 81.70930933238793159, -5.935454207752202116, 77.87546120947918382 ) ) ;
#19104=CARTESIAN_POINT ( 'NONE',  ( 0.6836613156275018754, 11.92558985988973497, 99.04321908912905315 ) ) ;
#19117=CARTESIAN_POINT ( 'NONE',  ( -30.88776590959009738, 11.92558985988972964, 26.61401058482698545 ) ) ;
#19154=CARTESIAN_POINT ( 'NONE',  ( 41.51205063648688309, 1.925589859889728972, -37.95069200549950494 ) ) ;
#19172=EDGE_CURVE ( 'NONE', #20563, #15480, #30607, .T. ) ;
#19183=CARTESIAN_POINT ( 'NONE',  ( -35.40773169500607054, 11.64114591743160076, 41.11337043081405795 ) ) ;
#19184=DIRECTION ( 'NONE',  ( -0.000000000000000000, -1.000000000000000000, 0.000000000000000000 ) ) ;
#19187=FACE_OUTER_BOUND ( 'NONE', #12532, .T. ) ;
#19200=CARTESIAN_POINT ( 'NONE',  ( -12.54358740205593215, -1.580002914024313254, -7.565473790375000895 ) ) ;
#19206=CIRCLE ( 'NONE', #8216, 56.65825807113184709 ) ;
#19220=CARTESIAN_POINT ( 'NONE',  ( 54.27408594025197175, -4.576799740321103371, -8.853384888801278052 ) ) ;
#19233=EDGE_LOOP ( 'NONE', ( #27245, #26405 ) ) ;
#19234=CARTESIAN_POINT ( 'NONE',  ( -39.55199796652554767, -5.935626912768316998, 77.88283516045706278 ) ) ;
#19236=CARTESIAN_POINT ( 'NONE',  ( -44.35518986140444753, -4.284653979202247776, 42.04930799450063716 ) ) ;
#19239=ORIENTED_EDGE ( 'NONE', *, *, #27431, .T. ) ;
#19241=DIRECTION ( 'NONE',  ( -0.000000000000000000, -1.000000000000000000, -0.000000000000000000 ) ) ;
#19244=DIRECTION ( 'NONE',  ( 0.000000000000000000, 0.000000000000000000, 1.000000000000000000 ) ) ;
#19249=ORIENTED_EDGE ( 'NONE', *, *, #7805, .T. ) ;
#19255=CARTESIAN_POINT ( 'NONE',  ( 52.21187923486668581, -5.935340315990531579, 107.6772108465075490 ) ) ;
#19257=CARTESIAN_POINT ( 'NONE',  ( -31.41618342396850494, 0.9942232071982006758, 79.85214699334892430 ) ) ;
#19258=CARTESIAN_POINT ( 'NONE',  ( 81.65861757311864721, -5.935454078358223917, 78.02743665865710909 ) ) ;
#19261=VERTEX_POINT ( 'NONE', #31884 ) ;
#19267=DIRECTION ( 'NONE',  ( 0.000000000000000000, 0.000000000000000000, 1.000000000000000000 ) ) ;
#19274=CIRCLE ( 'NONE', #6711, 2.500000000000002220 ) ;
#19283=B_SPLINE_CURVE_WITH_KNOTS ( 'NONE', 3,
 ( #10188, #22810, #30369, #8362, #324, #5581, #25439, #27741, #18359, #15107, #20672, #10345 ),
 .UNSPECIFIED., .F., .F.,
 ( 4, 2, 2, 2, 2, 4 ),
 ( 0.000000000000000000, 7.988424390472266816E-05, 0.0001597684878094453363, 0.0001997106097618206498, 0.0002396527317141959905, 0.0003195369756189209219 ),
 .UNSPECIFIED. ) ;
#19284=EDGE_CURVE ( 'NONE', #29304, #28041, #13924, .T. ) ;
#19285=CARTESIAN_POINT ( 'NONE',  ( -63.90214402394282445, 11.92558985988973674, 54.04930799450053769 ) ) ;
#19290=CIRCLE ( 'NONE', #27171, 55.85791022362053582 ) ;
#19297=DIRECTION ( 'NONE',  ( 1.000000000000000000, 0.000000000000000000, -1.224646799147353207E-16 ) ) ;
#19298=VERTEX_POINT ( 'NONE', #5459 ) ;
#19305=EDGE_LOOP ( 'NONE', ( #20816, #16054, #7829, #13782, #825 ) ) ;
#19308=CARTESIAN_POINT ( 'NONE',  ( -12.64026357700385716, -2.474457146986663414, -7.147442258105406232 ) ) ;
#19329=ORIENTED_EDGE ( 'NONE', *, *, #6930, .T. ) ;
#19335=EDGE_LOOP ( 'NONE', ( #29452, #27663, #10878, #14451, #27938, #28955, #26267, #6055, #5939, #29372, #7545, #787, #22326, #3571, #28217, #5513, #2550, #11477, #3030, #18597, #8724, #29119 ) ) ;
#19344=VECTOR ( 'NONE', #7563, 1000.000000000000000 ) ;
#19354=DIRECTION ( 'NONE',  ( 0.000000000000000000, -0.000000000000000000, -1.000000000000000000 ) ) ;
#19366=CARTESIAN_POINT ( 'NONE',  ( -8.645724211769511669, 6.334306897662572489, -4.780293558379808516 ) ) ;
#19374=ADVANCED_FACE ( 'NONE', ( #32222 ), #21773, .T. ) ;
#19375=EDGE_CURVE ( 'NONE', #5070, #20563, #13425, .T. ) ;
#19398=AXIS2_PLACEMENT_3D ( 'NONE', #31712, #26296, #21192 ) ;
#19403=AXIS2_PLACEMENT_3D ( 'NONE', #17918, #23331, #30885 ) ;
#19405=CARTESIAN_POINT ( 'NONE',  ( -29.42591059354393934, 10.36022259761711162, 21.25795413502442699 ) ) ;
#19406=CARTESIAN_POINT ( 'NONE',  ( 52.97684575647971172, -5.738638231773880882, 104.4392655406692256 ) ) ;
#19408=CARTESIAN_POINT ( 'NONE',  ( -39.56997771603464997, -5.935920012143626856, 77.89936816942207543 ) ) ;
#19413=CARTESIAN_POINT ( 'NONE',  ( -39.57405207560572791, -5.935454207752198563, 77.87546120947918382 ) ) ;
#19415=DIRECTION ( 'NONE',  ( -0.000000000000000000, -0.000000000000000000, 1.000000000000000000 ) ) ;
#19427=ORIENTED_EDGE ( 'NONE', *, *, #19375, .T. ) ;
#19430=CARTESIAN_POINT ( 'NONE',  ( -31.71490984672070823, 0.2276820184178854067, 80.17571310813880814 ) ) ;
#19439=FACE_OUTER_BOUND ( 'NONE', #27211, .T. ) ;
#19444=CARTESIAN_POINT ( 'NONE',  ( 21.09785597605719332, -8.535454207752287914, 47.04930799450051637 ) ) ;
#19457=CIRCLE ( 'NONE', #25695, 55.00000000000000000 ) ;
#19479=CARTESIAN_POINT ( 'NONE',  ( -9.248156207842958665, 5.417291301124353531, -4.090610767477680376 ) ) ;
#19480=VECTOR ( 'NONE', #14215, 1000.000000000000000 ) ;
#19485=CARTESIAN_POINT ( 'NONE',  ( 52.07598125554712709, -5.935454207752203004, 107.6091390186649761 ) ) ;
#19487=LINE ( 'NONE', #26233, #12760 ) ;
#19492=ORIENTED_EDGE ( 'NONE', *, *, #12588, .F. ) ;
#19504=B_SPLINE_SURFACE_WITH_KNOTS ( 'NONE', 3, 1, ( 
 ( #2873, #14265 ),
 ( #5352, #15350 ),
 ( #4563, #24756 ),
 ( #408, #27830 ),
 ( #17189, #2273 ),
 ( #22895, #14585 ),
 ( #26890, #1938 ),
 ( #27210, #16702 ),
 ( #9660, #24423 ),
 ( #24262, #19656 ),
 ( #11956, #6875 ),
 ( #29687, #2104 ) ),
 .UNSPECIFIED., .F., .F., .F.,
 ( 4, 1, 1, 1, 1, 1, 1, 1, 1, 4 ),
 ( 2, 2 ),
 ( 0.000000000000000000, 0.06961316558564611956, 0.1171086334586786126, 0.1635501317099198326, 0.2110163436193570607, 0.3800399093095634395, 0.5436454160257098156, 0.6849566023255588831, 0.8083832489416957756, 1.000000000000000000 ),
 ( 0.000000000000000000, 1.000000000000000000 ),
 .UNSPECIFIED. ) ;
#19507=CARTESIAN_POINT ( 'NONE',  ( 51.67049335409638644, 5.388785998227653806, -3.337848843846767721 ) ) ;
#19510=ORIENTED_EDGE ( 'NONE', *, *, #4755, .F. ) ;
#19514=CARTESIAN_POINT ( 'NONE',  ( -10.01358250815963125, -5.935454354499447582, -13.39048028849681771 ) ) ;
#19517=CARTESIAN_POINT ( 'NONE',  ( -39.51359738027355206, -5.935454207752198563, 77.87546120947918382 ) ) ;
#19524=CARTESIAN_POINT ( 'NONE',  ( -45.22803192368630931, -5.771461585458397714, 40.85022782416209708 ) ) ;
#19533=CARTESIAN_POINT ( 'NONE',  ( -9.732626758893591301, 4.638969541771042593, -5.235519273104768168 ) ) ;
#19535=CIRCLE ( 'NONE', #5399, 19.99999999999999645 ) ;
#19544=CARTESIAN_POINT ( 'NONE',  ( 47.79865503179234310, 9.702389020015065313, -3.412202488244239884 ) ) ;
#19561=AXIS2_PLACEMENT_3D ( 'NONE', #4558, #14416, #11628 ) ;
#19563=FACE_BOUND ( 'NONE', #25085, .T. ) ;
#19575=DIRECTION ( 'NONE',  ( -0.000000000000000000, -1.000000000000000000, -0.000000000000000000 ) ) ;
#19580=CARTESIAN_POINT ( 'NONE',  ( -7.324817582041172948, 8.310461108307681144, -3.351769630585352377 ) ) ;
#19587=AXIS2_PLACEMENT_3D ( 'NONE', #10601, #8605, #15509 ) ;
#19593=CARTESIAN_POINT ( 'NONE',  ( -30.88361636257000598, 11.92558985988973141, 67.49515520264003499 ) ) ;
#19600=CARTESIAN_POINT ( 'NONE',  ( -37.21204910874187988, -5.721341737285086992, 15.20211895544695757 ) ) ;
#19602=CARTESIAN_POINT ( 'NONE',  ( 21.09785597605719332, 11.92558985988973497, 47.04930799450051637 ) ) ;
#19626=EDGE_LOOP ( 'NONE', ( #10966, #15286, #13079, #24381 ) ) ;
#19630=DIRECTION ( 'NONE',  ( 0.000000000000000000, -1.000000000000000000, 0.000000000000000000 ) ) ;
#19632=EDGE_CURVE ( 'NONE', #19261, #4546, #9289, .T. ) ;
#19636=CARTESIAN_POINT ( 'NONE',  ( -30.67295000222299706, 6.587260180950779365, 17.48485802005428624 ) ) ;
#19646=CYLINDRICAL_SURFACE ( 'NONE', #6882, 2.500000000000002220 ) ;
#19648=CIRCLE ( 'NONE', #18584, 39.69941114636694124 ) ;
#19656=CARTESIAN_POINT ( 'NONE',  ( -29.27337757263006424, 11.23353061944650655, 22.24400271019782593 ) ) ;
#19664=EDGE_CURVE ( 'NONE', #14591, #32254, #15518, .T. ) ;
#19665=ORIENTED_EDGE ( 'NONE', *, *, #14802, .F. ) ;
#19670=( GEOMETRIC_REPRESENTATION_CONTEXT ( 3 ) GLOBAL_UNCERTAINTY_ASSIGNED_CONTEXT ( ( #25891 ) ) GLOBAL_UNIT_ASSIGNED_CONTEXT ( ( #18266, #3340, #23367 ) ) REPRESENTATION_CONTEXT ( 'NONE', 'WORKASPACE' ) );
#19675=PLANE ( 'NONE',  #11679 ) ;
#19682=CARTESIAN_POINT ( 'NONE',  ( 21.09785597605719332, 12.11061942510878886, 47.04930799450051637 ) ) ;
#19685=CARTESIAN_POINT ( 'NONE',  ( -45.06166779280744095, -5.721341737285086992, 40.94964444931001424 ) ) ;
#19692=CARTESIAN_POINT ( 'NONE',  ( 21.09785597605720042, -8.535454207752287914, 115.0493079945004951 ) ) ;
#19693=ORIENTED_EDGE ( 'NONE', *, *, #18457, .F. ) ;
#19694=CARTESIAN_POINT ( 'NONE',  ( 52.10659382688164243, -5.936607700120022812, 107.4592332772410259 ) ) ;
#19698=DIRECTION ( 'NONE',  ( 0.000000000000000000, -1.000000000000000000, 0.000000000000000000 ) ) ;
#19708=ORIENTED_EDGE ( 'NONE', *, *, #25492, .T. ) ;
#19713=CARTESIAN_POINT ( 'NONE',  ( 21.09785597605719332, -16.43545420775217281, 132.0493079945005377 ) ) ;
#19715=AXIS2_PLACEMENT_3D ( 'NONE', #4067, #14097, #6698 ) ;
#19716=CARTESIAN_POINT ( 'NONE',  ( 52.36305255737380548, 3.903925281081623844, -4.517372811625020468 ) ) ;
#19722=DIRECTION ( 'NONE',  ( 0.000000000000000000, -1.000000000000000000, 0.000000000000000000 ) ) ;
#19726=DIRECTION ( 'NONE',  ( 0.000000000000000000, 1.000000000000000000, 0.000000000000000000 ) ) ;
#19730=CARTESIAN_POINT ( 'NONE',  ( 80.85108986838919520, 8.310461108307681144, 75.47198155259910379 ) ) ;
#19734=CARTESIAN_POINT ( 'NONE',  ( 43.69445516536492846, 11.70027025134008625, -4.173706942055579461 ) ) ;
#19745=EDGE_CURVE ( 'NONE', #10438, #14591, #322, .T. ) ;
#19749=EDGE_CURVE ( 'NONE', #16051, #7822, #30733, .T. ) ;
#19752=FACE_OUTER_BOUND ( 'NONE', #19335, .T. ) ;
#19754=B_SPLINE_CURVE_WITH_KNOTS ( 'NONE', 3,
 ( #22233, #9778, #12567, #19768, #22392, #22729, #7312, #27331, #9935, #19936, #7481, #22556, #20101, #17479, #30131, #27653, #5176, #245, #5981, #28467, #3016, #20903, #880, #25515, #11073, #10907, #13378, #28148, #25989, #21057 ),
 .UNSPECIFIED., .F., .F.,
 ( 4, 2, 2, 2, 2, 2, 2, 2, 2, 2, 2, 2, 2, 2, 4 ),
 ( 0.000000000000000000, 0.001249755272498811022, 0.002499510544997622045, 0.003749265817496432850, 0.004999021089995244090, 0.007498531634992865701, 0.009998042179990488179, 0.01249755272498811152, 0.01374730799748691452, 0.01499706326998571926, 0.01562194090623512423, 0.01624681854248452573, 0.01749657381498331485, 0.01874632908748210397, 0.01999608435998089309 ),
 .UNSPECIFIED. ) ;
#19755=ORIENTED_EDGE ( 'NONE', *, *, #27022, .T. ) ;
#19762=CARTESIAN_POINT ( 'NONE',  ( 71.97287007337540388, 6.453333540778382726, 76.71314589128250816 ) ) ;
#19768=CARTESIAN_POINT ( 'NONE',  ( 72.50791967827838391, 8.582373042058220491, 74.98955504367758351 ) ) ;
#19778=ORIENTED_EDGE ( 'NONE', *, *, #2846, .F. ) ;
#19800=CARTESIAN_POINT ( 'NONE',  ( -34.86662712495122918, -3.622750763374904093, 13.44772519608141437 ) ) ;
#19812=DIRECTION ( 'NONE',  ( 0.000000000000000000, 0.000000000000000000, 1.000000000000000000 ) ) ;
#19813=DIRECTION ( 'NONE',  ( 8.659560562354994488E-17, -0.7071067811865426878, 0.7071067811865524577 ) ) ;
#19823=VECTOR ( 'NONE', #26526, 1000.000000000000114 ) ;
#19827=ORIENTED_EDGE ( 'NONE', *, *, #11861, .F. ) ;
#19828=ADVANCED_FACE ( 'NONE', ( #10511 ), #20506, .F. ) ;
#19853=CARTESIAN_POINT ( 'NONE',  ( 21.09785597605719332, -5.721341737285094098, 47.04930799450051637 ) ) ;
#19863=CARTESIAN_POINT ( 'NONE',  ( -43.35833523721898075, -3.935454207752190126, 42.04930799450051637 ) ) ;
#19875=DIRECTION ( 'NONE',  ( 0.000000000000000000, 0.000000000000000000, 1.000000000000000000 ) ) ;
#19878=CARTESIAN_POINT ( 'NONE',  ( 54.10256253235530721, 0.5083845707908396516, -5.656102003009075396 ) ) ;
#19885=DIRECTION ( 'NONE',  ( 0.000000000000000000, 0.000000000000000000, -1.000000000000000000 ) ) ;
#19886=FACE_BOUND ( 'NONE', #10363, .T. ) ;
#19893=DIRECTION ( 'NONE',  ( 0.000000000000000000, 0.000000000000000000, -1.000000000000000000 ) ) ;
#19895=VECTOR ( 'NONE', #23053, 1000.000000000000000 ) ;
#19896=CARTESIAN_POINT ( 'NONE',  ( 80.85108986838918099, -5.983766253076979069, 79.12126923977233162 ) ) ;
#19905=CARTESIAN_POINT ( 'NONE',  ( -39.39739818181173803, -5.936374393131169214, 77.91251232197767251 ) ) ;
#19910=ORIENTED_EDGE ( 'NONE', *, *, #14901, .F. ) ;
#19921=CONICAL_SURFACE ( 'NONE', #1592, 84.50502525316943547, 0.7853981633974621568 ) ;
#19927=CARTESIAN_POINT ( 'NONE',  ( 21.09785597605719332, -5.986312001189870280, 47.04930799450051637 ) ) ;
#19930=CARTESIAN_POINT ( 'NONE',  ( 71.81585295342675579, 7.161243906346035359, 76.20117120572383840 ) ) ;
#19934=ADVANCED_FACE ( 'NONE', ( #13458 ), #17887, .T. ) ;
#19936=CARTESIAN_POINT ( 'NONE',  ( 73.19123048883250249, 5.308358430270040174, 77.47344046293443398 ) ) ;
#19937=ORIENTED_EDGE ( 'NONE', *, *, #24192, .F. ) ;
#19956=ORIENTED_EDGE ( 'NONE', *, *, #5054, .F. ) ;
#19957=CARTESIAN_POINT ( 'NONE',  ( 76.91269118277453742, -4.491775094913941224, 13.81757365283580796 ) ) ;
#19961=CARTESIAN_POINT ( 'NONE',  ( 21.09785597605719332, 13.06454579224780055, 47.04930799450051637 ) ) ;
#19962=LINE ( 'NONE', #29993, #8935 ) ;
#19966=ORIENTED_EDGE ( 'NONE', *, *, #25855, .T. ) ;
#19973=FACE_OUTER_BOUND ( 'NONE', #22071, .T. ) ;
#19975=CARTESIAN_POINT ( 'NONE',  ( 0.6836613156275053171, 11.92558985988973497, -37.95069200549950494 ) ) ;
#19989=DIRECTION ( 'NONE',  ( 0.000000000000000000, -1.000000000000000000, 0.000000000000000000 ) ) ;
#19990=ORIENTED_EDGE ( 'NONE', *, *, #8808, .F. ) ;
#19995=VECTOR ( 'NONE', #4510, 1000.000000000000000 ) ;
#20004=CARTESIAN_POINT ( 'NONE',  ( -9.975557855541882901, -5.936694392936853859, -13.32360845848466013 ) ) ;
#20007=ORIENTED_EDGE ( 'NONE', *, *, #15268, .T. ) ;
#20023=LINE ( 'NONE', #19692, #19344 ) ;
#20028=PLANE ( 'NONE',  #28568 ) ;
#20029=CONICAL_SURFACE ( 'NONE', #4832, 72.49999999999997158, 0.7853981633974482790 ) ;
#20037=CARTESIAN_POINT ( 'NONE',  ( -37.45475073248209696, -5.768184894878238822, 15.30568074843956516 ) ) ;
#20047=CARTESIAN_POINT ( 'NONE',  ( 21.09785597605719332, -19.93545420775220123, 47.04930799450051637 ) ) ;
#20059=VERTEX_POINT ( 'NONE', #6216 ) ;
#20063=CARTESIAN_POINT ( 'NONE',  ( 21.09785597605719332, -15.72540370141337007, 118.3493079945004922 ) ) ;
#20067=DIRECTION ( 'NONE',  ( -0.000000000000000000, 1.000000000000000000, -0.000000000000000000 ) ) ;
#20069=CARTESIAN_POINT ( 'NONE',  ( 46.84806919170409145, 10.40257568944042887, -3.470939490021768936 ) ) ;
#20074=CARTESIAN_POINT ( 'NONE',  ( -14.16142858629410028, -3.295808585244882849, -12.62465409255485582 ) ) ;
#20091=CARTESIAN_POINT ( 'NONE',  ( 21.09785597605733187, -5.935454207752083988, 47.04930799450051637 ) ) ;
#20095=VERTEX_POINT ( 'NONE', #26401 ) ;
#20100=CIRCLE ( 'NONE', #26370, 72.49999999999997158 ) ;
#20101=CARTESIAN_POINT ( 'NONE',  ( 74.01572245777501280, 2.529769287487848128, 79.09906317329492254 ) ) ;
#20109=VECTOR ( 'NONE', #25033, 1000.000000000000000 ) ;
#20117=ADVANCED_FACE ( 'NONE', ( #16539 ), #29186, .F. ) ;
#20119=CARTESIAN_POINT ( 'NONE',  ( -9.843081575490945312, -5.936629510748248073, 107.7114293576719604 ) ) ;
#20122=CARTESIAN_POINT ( 'NONE',  ( 79.10241889060681331, -5.935454207752202116, 16.07118271501078510 ) ) ;
#20124=DIRECTION ( 'NONE',  ( -0.000000000000000000, -1.000000000000000000, -0.000000000000000000 ) ) ;
#20129=CARTESIAN_POINT ( 'NONE',  ( -12.39242563034483169, -3.977894809549909816, 102.3767317286982603 ) ) ;
#20136=CARTESIAN_POINT ( 'NONE',  ( 81.72488390788849699, -5.936701049740617187, 16.03361580170941991 ) ) ;
#20137=DIRECTION ( 'NONE',  ( -0.000000000000000000, -1.000000000000000000, -0.000000000000000000 ) ) ;
#20150=VECTOR ( 'NONE', #22752, 1000.000000000000000 ) ;
#20159=EDGE_CURVE ( 'NONE', #5895, #4564, #4568, .T. ) ;
#20163=CIRCLE ( 'NONE', #13367, 55.72436264418301732 ) ;
#20198=ORIENTED_EDGE ( 'NONE', *, *, #32405, .F. ) ;
#20202=EDGE_CURVE ( 'NONE', #20095, #17152, #30615, .T. ) ;
#20217=VERTEX_POINT ( 'NONE', #8127 ) ;
#20222=EDGE_CURVE ( 'NONE', #6305, #26270, #10343, .T. ) ;
#20224=CARTESIAN_POINT ( 'NONE',  ( 50.24465560486001436, 7.198184577528759398, 97.74814760920997969 ) ) ;
#20233=ADVANCED_FACE ( 'NONE', ( #29682 ), #9656, .F. ) ;
#20234=EDGE_CURVE ( 'NONE', #5971, #20242, #24472, .T. ) ;
#20237=DIRECTION ( 'NONE',  ( -1.000000000000000000, -0.000000000000000000, -0.000000000000000000 ) ) ;
#20242=VERTEX_POINT ( 'NONE', #24752 ) ;
#20243=CARTESIAN_POINT ( 'NONE',  ( -9.728297238921257417, -5.935454207752202116, 107.7511683020618278 ) ) ;
#20246=ORIENTED_EDGE ( 'NONE', *, *, #10857, .T. ) ;
#20251=DIRECTION ( 'NONE',  ( -1.000000000000000000, -0.000000000000000000, -3.491481338843133355E-15 ) ) ;
#20254=CARTESIAN_POINT ( 'NONE',  ( -9.917836216733666888, -5.936701049740607417, -13.57771993733065408 ) ) ;
#20260=CARTESIAN_POINT ( 'NONE',  ( 21.09785597605719332, 14.77459629858661572, 47.04930799450051637 ) ) ;
#20262=CARTESIAN_POINT ( 'NONE',  ( -10.00793156682730611, -5.936611295272323119, -12.50776140503650247 ) ) ;
#20263=DIRECTION ( 'NONE',  ( 1.000000000000000000, -0.000000000000000000, -0.000000000000000000 ) ) ;
#20265=CARTESIAN_POINT ( 'NONE',  ( 21.09785597605719332, 15.06454579224778456, 47.04930799450051637 ) ) ;
#20267=CARTESIAN_POINT ( 'NONE',  ( 21.09785597605719332, 25.56454579224780232, -32.16074251183835031 ) ) ;
#20270=DIRECTION ( 'NONE',  ( -0.000000000000000000, -1.000000000000000000, -0.000000000000000000 ) ) ;
#20272=CIRCLE ( 'NONE', #9791, 54.29999999999999716 ) ;
#20274=EDGE_CURVE ( 'NONE', #21967, #8138, #9278, .T. ) ;
#20275=CARTESIAN_POINT ( 'NONE',  ( -9.728297238921253864, -5.935454207752203892, 107.6877921759662371 ) ) ;
#20278=ORIENTED_EDGE ( 'NONE', *, *, #5406, .F. ) ;
#20282=CARTESIAN_POINT ( 'NONE',  ( -33.09327977158311285, -0.7531705753110401469, 80.50456572937015665 ) ) ;
#20285=ORIENTED_EDGE ( 'NONE', *, *, #28636, .F. ) ;
#20288=CARTESIAN_POINT ( 'NONE',  ( 80.51541434188031587, -5.922252862938464091, 15.78525142915797019 ) ) ;
#20306=ORIENTED_EDGE ( 'NONE', *, *, #22036, .T. ) ;
#20313=B_SPLINE_SURFACE_WITH_KNOTS ( 'NONE', 3, 1, ( 
 ( #28519, #1248 ),
 ( #8328, #3552 ),
 ( #13578, #20638 ),
 ( #5704, #18325 ) ),
 .UNSPECIFIED., .F., .F., .F.,
 ( 4, 4 ),
 ( 2, 2 ),
 ( 0.9911194921636460320, 1.000000000000000000 ),
 ( 0.000000000000000000, 1.000000000000000000 ),
 .UNSPECIFIED. ) ;
#20315=CARTESIAN_POINT ( 'NONE',  ( -9.728297238921257417, -5.935454207752202116, 107.6607613508313648 ) ) ;
#20354=CARTESIAN_POINT ( 'NONE',  ( -45.02407702159366920, -5.625351695555422360, 52.97525428799637126 ) ) ;
#20385=DIRECTION ( 'NONE',  ( -0.000000000000000000, -1.000000000000000000, -9.698999007525318993E-17 ) ) ;
#20399=ORIENTED_EDGE ( 'NONE', *, *, #15814, .F. ) ;
#20400=CYLINDRICAL_SURFACE ( 'NONE', #746, 19.99999999999999645 ) ;
#20413=ORIENTED_EDGE ( 'NONE', *, *, #10127, .F. ) ;
#20426=CARTESIAN_POINT ( 'NONE',  ( 21.09785597605719332, 24.86454579224779948, 86.74871914086746472 ) ) ;
#20431=CARTESIAN_POINT ( 'NONE',  ( 21.09785597605719332, -5.986312001189870280, 47.04930799450051637 ) ) ;
#20440=CARTESIAN_POINT ( 'NONE',  ( 51.99049785380602628, -5.936920032134866076, -13.40664378015324232 ) ) ;
#20441=CARTESIAN_POINT ( 'NONE',  ( -9.728297238921257417, -5.935454207752202116, 107.6607613508313648 ) ) ;
#20442=CARTESIAN_POINT ( 'NONE',  ( 81.46980107077142463, -5.937394852768786535, 15.98100540722295015 ) ) ;
#20449=CARTESIAN_POINT ( 'NONE',  ( 21.09785597605719687, 24.56454579224780232, 7.349896848133565364 ) ) ;
#20450=CARTESIAN_POINT ( 'NONE',  ( -35.75861581459462002, -4.595165398174183125, 80.20204475166471525 ) ) ;
#20468=ORIENTED_EDGE ( 'NONE', *, *, #32028, .F. ) ;
#20478=AXIS2_PLACEMENT_3D ( 'NONE', #25310, #12846, #510 ) ;
#20486=CARTESIAN_POINT ( 'NONE',  ( -4.902144023942810236, 24.86454579224779948, 49.54930799450078638 ) ) ;
#20490=EDGE_CURVE ( 'NONE', #1152, #23296, #32318, .T. ) ;
#20506=CYLINDRICAL_SURFACE ( 'NONE', #18685, 2.500000000000002220 ) ;
#20524=LINE ( 'NONE', #5762, #28832 ) ;
#20528=EDGE_CURVE ( 'NONE', #23463, #21709, #23954, .T. ) ;
#20533=DIRECTION ( 'NONE',  ( 0.000000000000000000, 0.000000000000000000, -1.000000000000000000 ) ) ;
#20540=CARTESIAN_POINT ( 'NONE',  ( 42.05836384037805686, 11.91446173404583853, 98.83287304499684467 ) ) ;
#20556=CIRCLE ( 'NONE', #12174, 2.500000000000002220 ) ;
#20557=CARTESIAN_POINT ( 'NONE',  ( -39.40147288705622941, -5.935926662576402890, 77.96005242632439547 ) ) ;
#20560=CARTESIAN_POINT ( 'NONE',  ( 21.09785597605719332, 11.92558985988973852, 47.04930799450051637 ) ) ;
#20563=VERTEX_POINT ( 'NONE', #17272 ) ;
#20570=CIRCLE ( 'NONE', #18485, 55.85791022362053582 ) ;
#20588=DIRECTION ( 'NONE',  ( -0.000000000000000000, -0.000000000000000000, 1.000000000000000000 ) ) ;
#20616=CARTESIAN_POINT ( 'NONE',  ( -31.54987825820634839, 11.92645443048831488, 67.99310208698472024 ) ) ;
#20621=ORIENTED_EDGE ( 'NONE', *, *, #18043, .T. ) ;
#20622=DIRECTION ( 'NONE',  ( 1.177206059073821606E-16, -0.2756373558169902815, 0.9612616959383214477 ) ) ;
#20626=CARTESIAN_POINT ( 'NONE',  ( 81.58903466081247302, -5.935454061169748385, 15.93786273650362872 ) ) ;
#20638=CARTESIAN_POINT ( 'NONE',  ( -9.925114359954182675, -5.937449718911893548, -13.32263710021335612 ) ) ;
#20663=CARTESIAN_POINT ( 'NONE',  ( 21.09785597605720397, -16.43545420775217281, 132.0493079945005377 ) ) ;
#20672=CARTESIAN_POINT ( 'NONE',  ( -9.880265915727269643, -5.935454337261168334, 107.5563424404352872 ) ) ;
#20674=EDGE_LOOP ( 'NONE', ( #27492, #9645, #17023, #23829 ) ) ;
#20681=VERTEX_POINT ( 'NONE', #5618 ) ;
#20689=ORIENTED_EDGE ( 'NONE', *, *, #7123, .F. ) ;
#20693=FACE_OUTER_BOUND ( 'NONE', #10553, .T. ) ;
#20699=CARTESIAN_POINT ( 'NONE',  ( 42.88478197795839719, 11.83483724345210142, 98.53854327536406288 ) ) ;
#20703=EDGE_LOOP ( 'NONE', ( #4163, #14300, #25756, #15566 ) ) ;
#20721=CARTESIAN_POINT ( 'NONE',  ( -34.77292974153792215, 11.39147729100211670, 52.68251853679213070 ) ) ;
#20738=CARTESIAN_POINT ( 'NONE',  ( -3.124322268014796844, 11.18949478403750142, 98.72270311105292251 ) ) ;
#20756=CARTESIAN_POINT ( 'NONE',  ( 54.78407068788227008, -1.823725651226680400, -7.696569431702434905 ) ) ;
#20769=CARTESIAN_POINT ( 'NONE',  ( -36.34052844068784083, -5.745355918706371412, 78.84831695185476974 ) ) ;
#20770=CARTESIAN_POINT ( 'NONE',  ( 81.72575882806418690, -5.935340315990521809, 15.93528473569102566 ) ) ;
#20772=CARTESIAN_POINT ( 'NONE',  ( 81.63175399755476747, -5.935454207809698346, 78.02743327247107175 ) ) ;
#20776=CARTESIAN_POINT ( 'NONE',  ( -30.67097509423727786, 6.595730531473362745, 76.60775000090053766 ) ) ;
#20786=CARTESIAN_POINT ( 'NONE',  ( 81.56333945993378620, -5.935454207834600204, 15.93786612339379083 ) ) ;
#20790=ORIENTED_EDGE ( 'NONE', *, *, #6448, .F. ) ;
#20798=ADVANCED_FACE ( 'NONE', ( #9541 ), #4112, .F. ) ;
#20800=EDGE_CURVE ( 'NONE', #31909, #29041, #2130, .T. ) ;
#20802=CARTESIAN_POINT ( 'NONE',  ( -12.63022165813546849, -2.878806504921737730, 102.4552866314799218 ) ) ;
#20805=AXIS2_PLACEMENT_3D ( 'NONE', #7360, #4729, #29522 ) ;
#20814=EDGE_CURVE ( 'NONE', #25945, #11226, #27649, .T. ) ;
#20816=ORIENTED_EDGE ( 'NONE', *, *, #7573, .T. ) ;
#20824=DIRECTION ( 'NONE',  ( 0.000000000000000000, 0.000000000000000000, -1.000000000000000000 ) ) ;
#20841=FACE_OUTER_BOUND ( 'NONE', #11133, .T. ) ;
#20846=DIRECTION ( 'NONE',  ( 0.000000000000000000, 0.000000000000000000, -1.000000000000000000 ) ) ;
#20848=CARTESIAN_POINT ( 'NONE',  ( 81.47236153510795020, -5.936967987714544037, 16.00176942158120141 ) ) ;
#20850=EDGE_CURVE ( 'NONE', #12194, #2898, #8022, .T. ) ;
#20854=EDGE_LOOP ( 'NONE', ( #14148, #26854, #31779, #29427 ) ) ;
#20861=FACE_OUTER_BOUND ( 'NONE', #25809, .T. ) ;
#20865=CARTESIAN_POINT ( 'NONE',  ( 21.09785597605719332, 24.86454579224779948, 75.54930799450052348 ) ) ;
#20874=CARTESIAN_POINT ( 'NONE',  ( -39.50399991082505124, -5.935463013562887191, 77.87581693445018516 ) ) ;
#20879=EDGE_CURVE ( 'NONE', #10718, #27541, #18209, .T. ) ;
#20894=CARTESIAN_POINT ( 'NONE',  ( 47.34331760472088746, 10.07047442526145531, 97.52091674703079605 ) ) ;
#20896=CARTESIAN_POINT ( 'NONE',  ( 0.1373481117363317960, 11.91446173404583853, -4.734257055995808372 ) ) ;
#20903=CARTESIAN_POINT ( 'NONE',  ( 76.74774710317745985, -3.218976025669015417, 80.73895664570260067 ) ) ;
#20925=ORIENTED_EDGE ( 'NONE', *, *, #8766, .F. ) ;
#20934=FACE_OUTER_BOUND ( 'NONE', #13588, .T. ) ;
#20935=CARTESIAN_POINT ( 'NONE',  ( -4.902144023942810236, 25.56454579224779877, 47.04930799450078638 ) ) ;
#20936=FACE_OUTER_BOUND ( 'NONE', #9625, .T. ) ;
#20941=AXIS2_PLACEMENT_3D ( 'NONE', #17805, #5181, #15189 ) ;
#20953=EDGE_LOOP ( 'NONE', ( #32432, #16236 ) ) ;
#20955=CARTESIAN_POINT ( 'NONE',  ( -12.34210598815197812, -0.7249253372050598054, 101.2314873363451966 ) ) ;
#20957=ORIENTED_EDGE ( 'NONE', *, *, #13898, .T. ) ;
#20960=CARTESIAN_POINT ( 'NONE',  ( 80.77181806311267565, 5.388785998227650254, 16.47908017486096099 ) ) ;
#20966=EDGE_CURVE ( 'NONE', #1894, #8733, #4076, .T. ) ;
#20967=AXIS2_PLACEMENT_3D ( 'NONE', #20091, #721, #27484 ) ;
#20976=ORIENTED_EDGE ( 'NONE', *, *, #21150, .F. ) ;
#20978=CARTESIAN_POINT ( 'NONE',  ( 43.71041224836975658, 11.69686719848734313, 99.14099691200772213 ) ) ;
#20979=CARTESIAN_POINT ( 'NONE',  ( 53.55890038120063679, -5.379633064793138963, 104.8034930254145252 ) ) ;
#20984=ORIENTED_EDGE ( 'NONE', *, *, #18189, .T. ) ;
#20986=CARTESIAN_POINT ( 'NONE',  ( -32.52043329404533267, -1.482047863521116060, 13.42356643302901453 ) ) ;
#20989=CARTESIAN_POINT ( 'NONE',  ( 21.09785597605719332, -16.43545420775217281, 47.04930799450051637 ) ) ;
#20994=TOROIDAL_SURFACE ( 'NONE', #26762, 55.59552431147871232, 1.000000000000000000 ) ;
#21005=EDGE_CURVE ( 'NONE', #8194, #29763, #21364, .T. ) ;
#21010=DIRECTION ( 'NONE',  ( 0.000000000000000000, -1.000000000000000000, 0.000000000000000000 ) ) ;
#21030=CARTESIAN_POINT ( 'NONE',  ( -39.43067640719859668, -5.935531758779752032, 77.98141296025164593 ) ) ;
#21040=CARTESIAN_POINT ( 'NONE',  ( 21.09785597605720397, -16.43545420775217281, -37.95069200549950494 ) ) ;
#21041=DIRECTION ( 'NONE',  ( 8.659560562354932858E-17, -0.7071067811865474617, 0.7071067811865474617 ) ) ;
#21049=FACE_OUTER_BOUND ( 'NONE', #17547, .T. ) ;
#21057=CARTESIAN_POINT ( 'NONE',  ( 79.40776106085759523, -5.721341737285999152, 78.89649703355206611 ) ) ;
#21058=ORIENTED_EDGE ( 'NONE', *, *, #9830, .T. ) ;
#21062=CARTESIAN_POINT ( 'NONE',  ( -58.11219453028166981, -15.93545420775219945, 47.04930799450023926 ) ) ;
#21069=DIRECTION ( 'NONE',  ( 0.000000000000000000, 0.000000000000000000, -1.000000000000000000 ) ) ;
#21071=CARTESIAN_POINT ( 'NONE',  ( 73.74367965647046219, 11.91444431924556113, 26.08837878683308986 ) ) ;
#21087=DIRECTION ( 'NONE',  ( 0.000000000000000000, 0.000000000000000000, -1.000000000000000000 ) ) ;
#21115=VERTEX_POINT ( 'NONE', #11100 ) ;
#21131=DIRECTION ( 'NONE',  ( 0.000000000000000000, 0.000000000000000000, 1.000000000000000000 ) ) ;
#21132=CARTESIAN_POINT ( 'NONE',  ( -1.514700296255377054, 11.69686719848734313, -5.042380923006707150 ) ) ;
#21144=DIRECTION ( 'NONE',  ( -1.000000000000000000, 0.000000000000000000, 2.775557561562888984E-15 ) ) ;
#21150=EDGE_CURVE ( 'NONE', #6661, #27983, #21713, .T. ) ;
#21153=EDGE_LOOP ( 'NONE', ( #23148, #22741 ) ) ;
#21154=DIRECTION ( 'NONE',  ( 0.000000000000000000, 1.000000000000000000, 0.000000000000000000 ) ) ;
#21160=CARTESIAN_POINT ( 'NONE',  ( -36.17322415754387066, 10.41998892282475531, 42.00358830701785706 ) ) ;
#21162=VERTEX_POINT ( 'NONE', #20772 ) ;
#21165=DIRECTION ( 'NONE',  ( -3.551608010268815105E-15, 0.000000000000000000, 1.000000000000000000 ) ) ;
#21174=ORIENTED_EDGE ( 'NONE', *, *, #6448, .T. ) ;
#21180=LINE ( 'NONE', #1661, #27449 ) ;
#21190=EDGE_LOOP ( 'NONE', ( #3488, #12037 ) ) ;
#21192=DIRECTION ( 'NONE',  ( 0.000000000000000000, 0.000000000000000000, -1.000000000000000000 ) ) ;
#21211=VECTOR ( 'NONE', #20251, 1000.000000000000000 ) ;
#21214=VECTOR ( 'NONE', #27885, 1000.000000000000000 ) ;
#21219=DIRECTION ( 'NONE',  ( 0.000000000000000000, -1.000000000000000000, 0.000000000000000000 ) ) ;
#21224=CARTESIAN_POINT ( 'NONE',  ( 50.84778885652602298, 6.325917197325531482, -4.782011712722074925 ) ) ;
#21238=CARTESIAN_POINT ( 'NONE',  ( -33.34250707380372347, -2.843755992669095622, 80.78322013955785508 ) ) ;
#21241=VECTOR ( 'NONE', #4747, 1000.000000000000000 ) ;
#21244=EDGE_LOOP ( 'NONE', ( #31458, #11896 ) ) ;
#21250=DIRECTION ( 'NONE',  ( 0.000000000000000000, 0.000000000000000000, -1.000000000000000000 ) ) ;
#21252=CARTESIAN_POINT ( 'NONE',  ( 21.09785597605719687, 25.13358275951983956, 86.68484420190863204 ) ) ;
#21254=EDGE_CURVE ( 'NONE', #2086, #18205, #16152, .T. ) ;
#21257=CARTESIAN_POINT ( 'NONE',  ( -4.902144023942810236, 25.56454579224779877, 49.54930799450078638 ) ) ;
#21258=DIRECTION ( 'NONE',  ( -0.000000000000000000, -1.000000000000000000, -0.000000000000000000 ) ) ;
#21262=EDGE_LOOP ( 'NONE', ( #20413, #8151, #15015, #22056 ) ) ;
#21266=CARTESIAN_POINT ( 'NONE',  ( -43.80892580335221709, -4.771102634759627925, 41.87060378362927793 ) ) ;
#21276=EDGE_CURVE ( 'NONE', #12487, #25630, #14595, .T. ) ;
#21280=VERTEX_POINT ( 'NONE', #2689 ) ;
#21295=CARTESIAN_POINT ( 'NONE',  ( 52.94504501510867556, -5.721341737285968065, -11.26059709029990330 ) ) ;
#21309=ORIENTED_EDGE ( 'NONE', *, *, #27022, .F. ) ;
#21318=CARTESIAN_POINT ( 'NONE',  ( 72.45827002609743772, 9.438446991585321300, 20.02200133371455593 ) ) ;
#21330=CARTESIAN_POINT ( 'NONE',  ( -40.78929413070552101, 0.6853368522271082730, 52.04930799450050927 ) ) ;
#21352=CARTESIAN_POINT ( 'NONE',  ( 71.95763425453002071, 6.496515553941713428, 17.40581666385103077 ) ) ;
#21362=EDGE_LOOP ( 'NONE', ( #26400, #9091, #8959, #14908 ) ) ;
#21364=CIRCLE ( 'NONE', #9324, 2.500000000000002220 ) ;
#21380=AXIS2_PLACEMENT_3D ( 'NONE', #3649, #716, #13204 ) ;
#21397=DIRECTION ( 'NONE',  ( 0.000000000000000000, 0.000000000000000000, 1.000000000000000000 ) ) ;
#21405=FACE_BOUND ( 'NONE', #15241, .T. ) ;
#21410=DIRECTION ( 'NONE',  ( 0.000000000000000000, 1.450913048936738450E-16, -1.000000000000000000 ) ) ;
#21417=CARTESIAN_POINT ( 'NONE',  ( -44.22750734272732132, -5.641423040791120336, 41.10178114657359316 ) ) ;
#21427=AXIS2_PLACEMENT_3D ( 'NONE', #16065, #6550, #16543 ) ;
#21431=EDGE_CURVE ( 'NONE', #11560, #22567, #28364, .T. ) ;
#21437=VERTEX_POINT ( 'NONE', #23674 ) ;
#21441=CARTESIAN_POINT ( 'NONE',  ( 21.09785597605719332, 12.74140866975414887, 47.04930799450051637 ) ) ;
#21446=CARTESIAN_POINT ( 'NONE',  ( -11.94738134238030014, -4.768257113790713042, -9.054433584172935312 ) ) ;
#21447=ORIENTED_EDGE ( 'NONE', *, *, #18189, .F. ) ;
#21466=CARTESIAN_POINT ( 'NONE',  ( -34.31970563170438737, 11.92558985988973674, 40.04930799450050216 ) ) ;
#21467=CARTESIAN_POINT ( 'NONE',  ( 41.51205063648687599, 11.92558985988973497, 99.90211174246701376 ) ) ;
#21469=ADVANCED_FACE ( 'NONE', ( #29080 ), #7249, .F. ) ;
#21473=AXIS2_PLACEMENT_3D ( 'NONE', #15442, #13155, #6079 ) ;
#21477=AXIS2_PLACEMENT_3D ( 'NONE', #439, #10636, #10467 ) ;
#21481=VERTEX_POINT ( 'NONE', #22003 ) ;
#21484=CARTESIAN_POINT ( 'NONE',  ( 72.54327431645151592, 8.281585831149239851, 18.82624325624167838 ) ) ;
#21497=FACE_OUTER_BOUND ( 'NONE', #24009, .T. ) ;
#21499=CARTESIAN_POINT ( 'NONE',  ( -12.43099670031970838, -1.035104995753983959, -7.280064108657495758 ) ) ;
#21524=FACE_BOUND ( 'NONE', #12123, .T. ) ;
#21529=DIRECTION ( 'NONE',  ( -1.000000000000000000, 0.000000000000000000, 0.000000000000000000 ) ) ;
#21537=ORIENTED_EDGE ( 'NONE', *, *, #32028, .T. ) ;
#21538=CARTESIAN_POINT ( 'NONE',  ( -39.56789013741062178, -5.936135285505173442, 77.93152707003946489 ) ) ;
#21554=ORIENTED_EDGE ( 'NONE', *, *, #20800, .T. ) ;
#21586=CARTESIAN_POINT ( 'NONE',  ( -30.88361648749964772, 11.92558985988973141, 26.60346110398183583 ) ) ;
#21594=ORIENTED_EDGE ( 'NONE', *, *, #16959, .T. ) ;
#21605=CARTESIAN_POINT ( 'NONE',  ( 21.09785597605720042, 15.06454579224778456, -7.950692005499485404 ) ) ;
#21611=CARTESIAN_POINT ( 'NONE',  ( -38.53060556916744162, -5.935485795843228551, 78.00951309620023721 ) ) ;
#21615=DIRECTION ( 'NONE',  ( -1.000000000000000000, 0.000000000000000000, 0.000000000000000000 ) ) ;
#21619=CARTESIAN_POINT ( 'NONE',  ( 21.09785597605719332, -5.986312001188950127, 47.04930799450051637 ) ) ;
#21643=AXIS2_PLACEMENT_3D ( 'NONE', #21875, #13861, #1699 ) ;
#21652=CARTESIAN_POINT ( 'NONE',  ( 76.02014513276924390, -2.123693335316784836, 13.33257895622572065 ) ) ;
#21655=DIRECTION ( 'NONE',  ( -4.163336342344334660E-15, 0.000000000000000000, 1.000000000000000000 ) ) ;
#21665=CARTESIAN_POINT ( 'NONE',  ( -35.64882101543633297, 9.925589859889724309, 52.04930799450051637 ) ) ;
#21670=DIRECTION ( 'NONE',  ( 0.000000000000000000, -1.000000000000000000, 0.000000000000000000 ) ) ;
#21672=AXIS2_PLACEMENT_3D ( 'NONE', #26123, #10395, #31064 ) ;
#21673=CARTESIAN_POINT ( 'NONE',  ( -12.32854732834748468, -0.6709275202869608989, -7.106067055362325746 ) ) ;
#21681=CARTESIAN_POINT ( 'NONE',  ( -63.90214402394282445, -3.935454207752183020, 52.04930799450050927 ) ) ;
#21690=CARTESIAN_POINT ( 'NONE',  ( 54.70353123047690502, -3.653843372214150786, -7.997390199024978941 ) ) ;
#21691=EDGE_CURVE ( 'NONE', #20242, #32279, #22126, .T. ) ;
#21692=CARTESIAN_POINT ( 'NONE',  ( -9.728297238921268075, -5.935454207752198563, 106.7470117857220373 ) ) ;
#21703=DIRECTION ( 'NONE',  ( 0.000000000000000000, 0.000000000000000000, -1.000000000000000000 ) ) ;
#21706=CARTESIAN_POINT ( 'NONE',  ( -44.54447070791992758, -4.637414085371450945, 41.95757092055643511 ) ) ;
#21709=VERTEX_POINT ( 'NONE', #22492 ) ;
#21711=AXIS2_PLACEMENT_3D ( 'NONE', #31122, #18624, #18779 ) ;
#21713=B_SPLINE_CURVE_WITH_KNOTS ( 'NONE', 3,
 ( #10932, #13553, #755, #13403, #13249, #23239, #592, #1223, #30638, #25703, #23398, #8774 ),
 .UNSPECIFIED., .F., .F.,
 ( 4, 2, 2, 2, 2, 4 ),
 ( 0.0002262585095220170678, 0.001077298125046782578, 0.001928337740571547899, 0.002779377356096313437, 0.003204897163858691327, 0.003630416971621069650 ),
 .UNSPECIFIED. ) ;
#21720=ORIENTED_EDGE ( 'NONE', *, *, #30075, .T. ) ;
#21722=CARTESIAN_POINT ( 'NONE',  ( 52.07598125554711999, -5.935454207752202116, 107.6772108465075490 ) ) ;
#21736=DIRECTION ( 'NONE',  ( 1.775804005134407553E-15, 0.000000000000000000, 1.000000000000000000 ) ) ;
#21738=CARTESIAN_POINT ( 'NONE',  ( 21.09785597605719332, -19.93545420775220123, 47.04930799450051637 ) ) ;
#21740=DIRECTION ( 'NONE',  ( 0.000000000000000000, 0.000000000000000000, -1.000000000000000000 ) ) ;
#21752=CARTESIAN_POINT ( 'NONE',  ( -44.11954960567759088, -5.396560688972869002, 41.42132194764992903 ) ) ;
#21753=LINE ( 'NONE', #24543, #3819 ) ;
#21759=AXIS2_PLACEMENT_3D ( 'NONE', #22225, #7139, #7304 ) ;
#21763=EDGE_CURVE ( 'NONE', #28192, #7248, #10731, .T. ) ;
#21767=DIRECTION ( 'NONE',  ( 0.000000000000000000, 0.000000000000000000, -1.000000000000000000 ) ) ;
#21771=DIRECTION ( 'NONE',  ( 1.000000000000000000, -0.000000000000000000, -0.000000000000000000 ) ) ;
#21773=TOROIDAL_SURFACE ( 'NONE', #22843, 56.00000000000000000, 1.700000000000000178 ) ;
#21774=CARTESIAN_POINT ( 'NONE',  ( -12.63390874224687899, -2.844921901652555540, -7.393120321654669702 ) ) ;
#21775=( GEOMETRIC_REPRESENTATION_CONTEXT ( 3 ) GLOBAL_UNCERTAINTY_ASSIGNED_CONTEXT ( ( #3240 ) ) GLOBAL_UNIT_ASSIGNED_CONTEXT ( ( #27118, #16773, #31567 ) ) REPRESENTATION_CONTEXT ( 'NONE', 'WORKASPACE' ) );
#21781=DIRECTION ( 'NONE',  ( 0.000000000000000000, -0.000000000000000000, 1.000000000000000000 ) ) ;
#21796=FACE_OUTER_BOUND ( 'NONE', #29717, .T. ) ;
#21808=CARTESIAN_POINT ( 'NONE',  ( 53.16981722132879185, -5.983766253076979069, -12.70392589783158499 ) ) ;
#21812=ORIENTED_EDGE ( 'NONE', *, *, #632, .T. ) ;
#21815=CARTESIAN_POINT ( 'NONE',  ( 79.11899642186367032, -5.573920848077356105, 14.84471408225261690 ) ) ;
#21836=AXIS2_PLACEMENT_3D ( 'NONE', #10243, #20237, #15159 ) ;
#21838=ADVANCED_FACE ( 'NONE', ( #20841 ), #13153, .F. ) ;
#21857=CARTESIAN_POINT ( 'NONE',  ( 52.20929784716416577, -5.935454207834595763, 107.5147914783766510 ) ) ;
#21862=DIRECTION ( 'NONE',  ( 0.000000000000000000, -1.000000000000000000, 0.000000000000000000 ) ) ;
#21867=CARTESIAN_POINT ( 'NONE',  ( -45.02838518323464001, -5.632298750458708980, 41.12626815361094401 ) ) ;
#21868=DIRECTION ( 'NONE',  ( 0.000000000000000000, 0.000000000000000000, -1.000000000000000000 ) ) ;
#21872=CARTESIAN_POINT ( 'NONE',  ( -39.57405207560572791, -5.936352567920400780, 77.94940154167748858 ) ) ;
#21874=CARTESIAN_POINT ( 'NONE',  ( -5.602943079677954685, 9.702389020015065313, -37.95069200549950494 ) ) ;
#21875=CARTESIAN_POINT ( 'NONE',  ( 47.09785597605719687, 24.86454579224779948, 47.04930799450042400 ) ) ;
#21876=ORIENTED_EDGE ( 'NONE', *, *, #7651, .F. ) ;
#21897=EDGE_LOOP ( 'NONE', ( #9854, #1210, #9999, #24014 ) ) ;
#21900=CARTESIAN_POINT ( 'NONE',  ( 21.09785597605719332, -19.93545420775220123, 132.0493079945005377 ) ) ;
#21901=CYLINDRICAL_SURFACE ( 'NONE', #11135, 2.500000000000002220 ) ;
#21903=VECTOR ( 'NONE', #21041, 1000.000000000000114 ) ;
#21922=EDGE_CURVE ( 'NONE', #6650, #313, #5517, .T. ) ;
#21932=CARTESIAN_POINT ( 'NONE',  ( -7.213884129472804219, 8.185031362399401544, 97.59170711626282468 ) ) ;
#21943=CARTESIAN_POINT ( 'NONE',  ( 21.09785597605719332, 25.18020726757345429, 6.561886094526840907 ) ) ;
#21944=DIRECTION ( 'NONE',  ( 1.313185983435984691E-29, -1.000000000000000000, -3.761114140369702165E-15 ) ) ;
#21945=ORIENTED_EDGE ( 'NONE', *, *, #24016, .T. ) ;
#21946=DIRECTION ( 'NONE',  ( 0.000000000000000000, 1.000000000000000000, 0.000000000000000000 ) ) ;
#21954=ORIENTED_EDGE ( 'NONE', *, *, #31143, .F. ) ;
#21967=VERTEX_POINT ( 'NONE', #1629 ) ;
#21970=CARTESIAN_POINT ( 'NONE',  ( 73.78878393608395925, 3.260977705924042347, 15.40761682156110979 ) ) ;
#21994=CIRCLE ( 'NONE', #8885, 55.85791022362053582 ) ;
#21998=CIRCLE ( 'NONE', #26208, 65.75844861871138392 ) ;
#22003=CARTESIAN_POINT ( 'NONE',  ( 21.09785597605719332, -15.93545420775219945, -25.45069200549945165 ) ) ;
#22007=CARTESIAN_POINT ( 'NONE',  ( 21.09785597605719332, -19.93545420775220123, 47.04930799450051637 ) ) ;
#22009=CARTESIAN_POINT ( 'NONE',  ( 52.84805770882741882, -5.769399297529544057, -10.43150399477652179 ) ) ;
#22011=VECTOR ( 'NONE', #2514, 1000.000000000000000 ) ;
#22022=AXIS2_PLACEMENT_3D ( 'NONE', #25642, #23182, #7608 ) ;
#22027=CARTESIAN_POINT ( 'NONE',  ( 54.83597552911822959, -2.474457146986655864, 101.2460582471064328 ) ) ;
#22033=ORIENTED_EDGE ( 'NONE', *, *, #12172, .F. ) ;
#22036=EDGE_CURVE ( 'NONE', #22618, #23145, #27715, .T. ) ;
#22039=CARTESIAN_POINT ( 'NONE',  ( -7.324817582041172948, 8.310461108307681144, -12.62465409255485582 ) ) ;
#22054=CARTESIAN_POINT ( 'NONE',  ( -29.52701465676184611, 10.77837282674672004, 72.12388452301328812 ) ) ;
#22056=ORIENTED_EDGE ( 'NONE', *, *, #26083, .F. ) ;
#22066=CARTESIAN_POINT ( 'NONE',  ( -10.00935122521091003, -5.935651417315361833, -13.46746157186161064 ) ) ;
#22071=EDGE_LOOP ( 'NONE', ( #29226, #14680, #32426, #12945 ) ) ;
#22074=CARTESIAN_POINT ( 'NONE',  ( -30.89191212020314481, 11.92558985988972964, 26.62456132884095794 ) ) ;
#22091=VERTEX_POINT ( 'NONE', #20315 ) ;
#22092=CARTESIAN_POINT ( 'NONE',  ( 78.62428479167849105, -5.811083640285387375, 15.33388578550628090 ) ) ;
#22102=CARTESIAN_POINT ( 'NONE',  ( -7.208542748348993001, 8.190330151142697801, -3.492701709236647911 ) ) ;
#22104=ORIENTED_EDGE ( 'NONE', *, *, #7859, .F. ) ;
#22114=DIRECTION ( 'NONE',  ( 0.000000000000000000, 0.000000000000000000, -1.000000000000000000 ) ) ;
#22117=EDGE_CURVE ( 'NONE', #26412, #29942, #24363, .T. ) ;
#22126=B_SPLINE_CURVE_WITH_KNOTS ( 'NONE', 3,
 ( #27920, #14965, #17246, #27261, #5437, #12674, #20037, #9872 ),
 .UNSPECIFIED., .F., .F.,
 ( 4, 2, 2, 4 ),
 ( 1.743375517060540341E-17, 0.0003981837892567215891, 0.0007963675785134257225, 0.001592735157026818702 ),
 .UNSPECIFIED. ) ;
#22131=CARTESIAN_POINT ( 'NONE',  ( 21.09785597605719332, -9.935454207752199451, 47.04930799450051637 ) ) ;
#22133=VERTEX_POINT ( 'NONE', #20486 ) ;
#22141=CARTESIAN_POINT ( 'NONE',  ( 106.0978559760575735, 1.925589859889728972, 26.63511333407112502 ) ) ;
#22143=DIRECTION ( 'NONE',  ( -3.761114140369701376E-15, -1.000000000000000000, -0.000000000000000000 ) ) ;
#22146=CARTESIAN_POINT ( 'NONE',  ( 21.09785597605719332, -15.43545420775221366, 119.0493079945005093 ) ) ;
#22150=ORIENTED_EDGE ( 'NONE', *, *, #17236, .F. ) ;
#22154=ADVANCED_FACE ( 'NONE', ( #3564 ), #5665, .F. ) ;
#22170=ORIENTED_EDGE ( 'NONE', *, *, #8021, .T. ) ;
#22179=CARTESIAN_POINT ( 'NONE',  ( 50.24971918728039100, 7.161243906346019372, -3.668688982869140691 ) ) ;
#22183=CARTESIAN_POINT ( 'NONE',  ( 21.09785597605719332, -16.63545420775219696, -34.66074251183835031 ) ) ;
#22189=ORIENTED_EDGE ( 'NONE', *, *, #30031, .T. ) ;
#22192=DIRECTION ( 'NONE',  ( 0.000000000000000000, 0.000000000000000000, 1.000000000000000000 ) ) ;
#22193=CARTESIAN_POINT ( 'NONE',  ( -30.47008420211899349, 11.87742387770962615, 25.50481123865409216 ) ) ;
#22194=EDGE_CURVE ( 'NONE', #9438, #11793, #10755, .T. ) ;
#22211=ORIENTED_EDGE ( 'NONE', *, *, #6844, .F. ) ;
#22224=FACE_OUTER_BOUND ( 'NONE', #12623, .T. ) ;
#22225=CARTESIAN_POINT ( 'NONE',  ( 21.09785597605719332, 12.39166260509097484, 47.04930799450051637 ) ) ;
#22233=CARTESIAN_POINT ( 'NONE',  ( 72.46310410352278097, 9.702389020015065313, 73.75010705023584023 ) ) ;
#22238=EDGE_CURVE ( 'NONE', #28492, #8138, #27146, .T. ) ;
#22256=CARTESIAN_POINT ( 'NONE',  ( 75.66689018375404885, -3.025068871688612937, 13.33232285377167337 ) ) ;
#22263=CARTESIAN_POINT ( 'NONE',  ( -38.44000803836371460, -5.928063154200345686, 78.12747986390417054 ) ) ;
#22265=CARTESIAN_POINT ( 'NONE',  ( -30.89758657727378832, 5.676337878349658972, 16.86309542392945104 ) ) ;
#22284=VECTOR ( 'NONE', #6493, 1000.000000000000114 ) ;
#22326=ORIENTED_EDGE ( 'NONE', *, *, #21150, .T. ) ;
#22332=AXIS2_PLACEMENT_3D ( 'NONE', #27805, #24853, #27634 ) ;
#22342=CARTESIAN_POINT ( 'NONE',  ( 53.40509610059028489, 2.044662169668915563, -5.087510015872766189 ) ) ;
#22351=ORIENTED_EDGE ( 'NONE', *, *, #22379, .F. ) ;
#22355=DIRECTION ( 'NONE',  ( 0.000000000000000000, 0.000000000000000000, -1.000000000000000000 ) ) ;
#22356=CIRCLE ( 'NONE', #32327, 84.50000000000002842 ) ;
#22357=CARTESIAN_POINT ( 'NONE',  ( 53.43087011377310347, -5.485531640240836282, 104.0244910283431494 ) ) ;
#22372=EDGE_LOOP ( 'NONE', ( #30286, #20957, #29085, #3692 ) ) ;
#22379=EDGE_CURVE ( 'NONE', #29498, #13639, #10903, .T. ) ;
#22386=VERTEX_POINT ( 'NONE', #27352 ) ;
#22387=CARTESIAN_POINT ( 'NONE',  ( 78.30297900732490746, -5.614579432636275236, 79.11844573034039740 ) ) ;
#22389=CARTESIAN_POINT ( 'NONE',  ( -10.01358589504979513, -5.935454207834595763, -13.41617548937563598 ) ) ;
#22392=CARTESIAN_POINT ( 'NONE',  ( 72.54334031540011551, 8.279996179725053196, 75.27408324235797465 ) ) ;
#22404=ADVANCED_FACE ( 'NONE', ( #2561 ), #15094, .T. ) ;
#22408=CIRCLE ( 'NONE', #6706, 2.500000000000002220 ) ;
#22414=CARTESIAN_POINT ( 'NONE',  ( 75.29460622866322694, -2.474457146986669187, 13.31118844143965951 ) ) ;
#22415=CARTESIAN_POINT ( 'NONE',  ( -43.68704682399115313, -4.539174506989449576, 52.13854715134223738 ) ) ;
#22419=CARTESIAN_POINT ( 'NONE',  ( -12.50781927836251128, -3.653843372214141461, 102.0960061880259815 ) ) ;
#22426=CARTESIAN_POINT ( 'NONE',  ( 52.20929784716416577, -5.935454207834595763, 107.5147914783766510 ) ) ;
#22443=FACE_OUTER_BOUND ( 'NONE', #27526, .T. ) ;
#22444=EDGE_CURVE ( 'NONE', #31580, #28492, #14066, .T. ) ;
#22466=DIRECTION ( 'NONE',  ( 0.000000000000000000, 1.446921688628131436E-16, -1.000000000000000000 ) ) ;
#22478=ORIENTED_EDGE ( 'NONE', *, *, #14598, .T. ) ;
#22481=DIRECTION ( 'NONE',  ( 0.000000000000000000, -1.000000000000000000, 0.000000000000000000 ) ) ;
#22492=CARTESIAN_POINT ( 'NONE',  ( 21.09785597605720042, 14.86454579224779948, 101.2593585008393404 ) ) ;
#22493=CARTESIAN_POINT ( 'NONE',  ( 72.51463730528963936, 10.40182650318959112, 72.80069388813021192 ) ) ;
#22496=CARTESIAN_POINT ( 'NONE',  ( -29.27613032885505007, 8.768497436727981764, 75.00977582921336762 ) ) ;
#22501=CIRCLE ( 'NONE', #4164, 1.000000000000000888 ) ;
#22504=CARTESIAN_POINT ( 'NONE',  ( 21.09785597605720397, -19.93545420775220123, -37.95069200549950494 ) ) ;
#22506=DIRECTION ( 'NONE',  ( 0.000000000000000000, 3.756723415560144304E-15, -1.000000000000000000 ) ) ;
#22517=VECTOR ( 'NONE', #14186, 1000.000000000000000 ) ;
#22518=FACE_OUTER_BOUND ( 'NONE', #4761, .T. ) ;
#22522=CARTESIAN_POINT ( 'NONE',  ( 21.09785597605719332, 17.56454579224779877, 47.04930799450051637 ) ) ;
#22523=CARTESIAN_POINT ( 'NONE',  ( 21.09785597605720042, 12.74140866975414887, 102.9204696617962185 ) ) ;
#22526=DIRECTION ( 'NONE',  ( 0.000000000000000000, -1.000000000000000000, 0.000000000000000000 ) ) ;
#22529=B_SPLINE_CURVE_WITH_KNOTS ( 'NONE', 3,
 ( #24542, #26849, #27504, #27167, #9618, #6828, #4687, #16983 ),
 .UNSPECIFIED., .F., .F.,
 ( 4, 2, 2, 4 ),
 ( 0.0002082711175172216199, 0.0005080769251113473285, 0.0008078827327054731184, 0.001407494347893724481 ),
 .UNSPECIFIED. ) ;
#22541=CARTESIAN_POINT ( 'NONE',  ( 21.09785597605720397, -15.93545420775219945, 119.5493079945004808 ) ) ;
#22543=AXIS2_PLACEMENT_3D ( 'NONE', #30101, #22526, #10390 ) ;
#22551=CARTESIAN_POINT ( 'NONE',  ( 71.55936645880184699, 9.702389020015065313, 73.75010705023584023 ) ) ;
#22552=CARTESIAN_POINT ( 'NONE',  ( -10.01358928193996434, -5.935454061169746609, -13.44187069025445602 ) ) ;
#22553=VECTOR ( 'NONE', #8394, 1000.000000000000000 ) ;
#22555=DIRECTION ( 'NONE',  ( 0.000000000000000000, 0.000000000000000000, 1.000000000000000000 ) ) ;
#22556=CARTESIAN_POINT ( 'NONE',  ( 73.79844651144168211, 3.230235421722119860, 78.70801319132137053 ) ) ;
#22567=VERTEX_POINT ( 'NONE', #12917 ) ;
#22590=ADVANCED_FACE ( 'NONE', ( #30635 ), #23226, .F. ) ;
#22594=CARTESIAN_POINT ( 'NONE',  ( -35.76350089666777876, -4.599861557816947055, 13.89978500458213873 ) ) ;
#22595=CARTESIAN_POINT ( 'NONE',  ( 79.88559988584306382, -5.819500620027728388, 15.36413957712890088 ) ) ;
#22596=CIRCLE ( 'NONE', #16287, 2.000000000000000000 ) ;
#22613=ADVANCED_FACE ( 'NONE', ( #588 ), #10619, .F. ) ;
#22617=CIRCLE ( 'NONE', #2197, 71.99999999999998579 ) ;
#22618=VERTEX_POINT ( 'NONE', #23237 ) ;
#22628=DIRECTION ( 'NONE',  ( -0.000000000000000000, -0.000000000000000000, -1.000000000000000000 ) ) ;
#22631=ORIENTED_EDGE ( 'NONE', *, *, #11130, .T. ) ;
#22637=CIRCLE ( 'NONE', #11635, 55.85791022362053582 ) ;
#22641=CARTESIAN_POINT ( 'NONE',  ( -5.602943079677954685, 9.702389020015065313, -4.315940132965163656 ) ) ;
#22653=DIRECTION ( 'NONE',  ( 1.177206059073964094E-16, -0.2756373558165849391, 0.9612616959384376880 ) ) ;
#22667=EDGE_CURVE ( 'NONE', #21162, #23266, #9932, .T. ) ;
#22676=CARTESIAN_POINT ( 'NONE',  ( 21.09785597605719332, -9.935454207752199451, 47.04930799450051637 ) ) ;
#22690=CARTESIAN_POINT ( 'NONE',  ( 71.48501281440437083, -5.983766253076979069, 79.12126923977230319 ) ) ;
#22692=AXIS2_PLACEMENT_3D ( 'NONE', #19285, #26850, #16831 ) ;
#22701=LINE ( 'NONE', #17279, #12029 ) ;
#22705=CIRCLE ( 'NONE', #26899, 2.500000000000002220 ) ;
#22721=CARTESIAN_POINT ( 'NONE',  ( -3.644339245467521859, 10.95889540305196341, 98.61699126615421562 ) ) ;
#22724=CARTESIAN_POINT ( 'NONE',  ( 79.18332612743283505, -5.935454207752198563, 77.87546120947918382 ) ) ;
#22727=CARTESIAN_POINT ( 'NONE',  ( -35.64882101543633297, 9.925589859889722533, 42.04930799450051637 ) ) ;
#22729=CARTESIAN_POINT ( 'NONE',  ( 72.64112472104469020, 7.651854857428991075, 75.81648953516938150 ) ) ;
#22734=CARTESIAN_POINT ( 'NONE',  ( -10.37754766804345508, -5.881344816830196720, -12.09508678449311070 ) ) ;
#22741=ORIENTED_EDGE ( 'NONE', *, *, #18967, .F. ) ;
#22749=EDGE_CURVE ( 'NONE', #9808, #27983, #19290, .T. ) ;
#22752=DIRECTION ( 'NONE',  ( -0.000000000000000000, -1.000000000000000000, -0.000000000000000000 ) ) ;
#22753=CARTESIAN_POINT ( 'NONE',  ( -30.40347463700609865, 7.917901822120666289, 75.58887676006128231 ) ) ;
#22758=CARTESIAN_POINT ( 'NONE',  ( -30.33894848875469918, 10.49891163461608379, 21.45876492183288420 ) ) ;
#22772=ORIENTED_EDGE ( 'NONE', *, *, #26861, .T. ) ;
#22778=AXIS2_PLACEMENT_3D ( 'NONE', #19050, #26941, #26456 ) ;
#22783=ADVANCED_FACE ( 'NONE', ( #5283 ), #30022, .F. ) ;
#22790=CIRCLE ( 'NONE', #12864, 56.65825807113184709 ) ;
#22791=EDGE_CURVE ( 'NONE', #13157, #1894, #16153, .T. ) ;
#22798=CIRCLE ( 'NONE', #8658, 56.65825807113184709 ) ;
#22799=EDGE_LOOP ( 'NONE', ( #12725, #31072, #7422, #15391 ) ) ;
#22802=CARTESIAN_POINT ( 'NONE',  ( 49.86372208582861276, 7.652955895019247556, 98.59261258995066157 ) ) ;
#22810=CARTESIAN_POINT ( 'NONE',  ( -9.728297238921260970, -5.935454207752201228, 107.6337305256964640 ) ) ;
#22825=CYLINDRICAL_SURFACE ( 'NONE', #21473, 2.500000000000002220 ) ;
#22833=PLANE ( 'NONE',  #10203 ) ;
#22834=CARTESIAN_POINT ( 'NONE',  ( 21.09785597605719332, 11.92558985988973497, -9.608950076631337822 ) ) ;
#22843=AXIS2_PLACEMENT_3D ( 'NONE', #30090, #27775, #32379 ) ;
#22846=CARTESIAN_POINT ( 'NONE',  ( -32.38499150730411458, -1.224855502300924437, 13.47596506989118836 ) ) ;
#22859=CONICAL_SURFACE ( 'NONE', #22332, 67.38776620500242132, 0.5061454830783623793 ) ;
#22862=EDGE_CURVE ( 'NONE', #21437, #19261, #30229, .T. ) ;
#22873=VERTEX_POINT ( 'NONE', #25776 ) ;
#22876=CARTESIAN_POINT ( 'NONE',  ( 80.64537389521012756, -5.931148802125833619, 78.13246447790419325 ) ) ;
#22895=CARTESIAN_POINT ( 'NONE',  ( -38.57628410747783221, -0.7885452029232787874, 13.38511290719907798 ) ) ;
#22897=CARTESIAN_POINT ( 'NONE',  ( -45.06166779280743384, -5.721341737285086992, 53.14897153969102561 ) ) ;
#22904=ADVANCED_FACE ( 'NONE', ( #28248 ), #5764, .F. ) ;
#22910=CARTESIAN_POINT ( 'NONE',  ( -44.11922148153472278, -5.395861642922686663, 52.67658529385213484 ) ) ;
#22918=VERTEX_POINT ( 'NONE', #8382 ) ;
#22927=DIRECTION ( 'NONE',  ( 0.000000000000000000, 0.000000000000000000, -1.000000000000000000 ) ) ;
#22929=CARTESIAN_POINT ( 'NONE',  ( 21.09785597605720397, -16.93042895458276575, 131.5543332476699732 ) ) ;
#22947=AXIS2_PLACEMENT_3D ( 'NONE', #26075, #15749, #13617 ) ;
#22948=EDGE_LOOP ( 'NONE', ( #7186, #30174 ) ) ;
#22952=CARTESIAN_POINT ( 'NONE',  ( 54.27971259635813084, 0.05876815387847823813, 100.8802911971805258 ) ) ;
#22969=CARTESIAN_POINT ( 'NONE',  ( -31.54952026363617179, 11.92645593095197754, 26.10458935450218831 ) ) ;
#22981=B_SPLINE_CURVE_WITH_KNOTS ( 'NONE', 3,
 ( #30376, #22969, #7895, #489, #30544, #17897, #27913, #22758, #2253, #12602, #29997, #15215, #12273, #24738, #19636, #22265, #32295, #7512, #7673, #9643, #17666, #7832, #15379, #24904, #17512, #9806, #27686, #29667, #27527, #30162, #19800, #5048, #4715, #22594, #15056, #12769, #29833, #7341, #25063, #12437 ),
 .UNSPECIFIED., .F., .F.,
 ( 4, 2, 2, 2, 2, 2, 2, 2, 2, 2, 2, 2, 2, 2, 2, 2, 2, 2, 2, 4 ),
 ( 3.469446951953614189E-18, 0.001682718673271781573, 0.003365437346543559676, 0.005048156019815338430, 0.006730874693087115883, 0.008413593366358893336, 0.01009631203963067339, 0.01177903071290245171, 0.01346174938617423177, 0.01682718673271779708, 0.01850990540598957540, 0.02019262407926135719, 0.02103398341589724982, 0.02187534275253314245, 0.02271670208916903508, 0.02355806142580492771, 0.02439942076244081687, 0.02524078009907670950, 0.02608213943571260213, 0.02692349877234849476 ),
 .UNSPECIFIED. ) ;
#22989=DIRECTION ( 'NONE',  ( -0.000000000000000000, -1.000000000000000000, -0.000000000000000000 ) ) ;
#23004=CARTESIAN_POINT ( 'NONE',  ( 21.09785597605719332, -15.93545420775219945, -25.45069200549945165 ) ) ;
#23006=CIRCLE ( 'NONE', #18213, 2.500000000000002220 ) ;
#23007=DIRECTION ( 'NONE',  ( 0.000000000000000000, 0.000000000000000000, -1.000000000000000000 ) ) ;
#23009=CARTESIAN_POINT ( 'NONE',  ( -39.51006936586720286, -5.935674496966103497, 77.97486924391246532 ) ) ;
#23017=CARTESIAN_POINT ( 'NONE',  ( -39.40510812339053359, -5.935838084272694992, 77.96604415839914282 ) ) ;
#23032=CARTESIAN_POINT ( 'NONE',  ( 80.43047408610513571, -5.903366343041404285, 78.33353586572610538 ) ) ;
#23035=CARTESIAN_POINT ( 'NONE',  ( -1.513221900615301818, 11.69718155787697533, -4.169217829025758881 ) ) ;
#23040=CARTESIAN_POINT ( 'NONE',  ( 77.29794470067753309, -4.853532562205578493, 80.02403050357165171 ) ) ;
#23049=ORIENTED_EDGE ( 'NONE', *, *, #11386, .F. ) ;
#23053=DIRECTION ( 'NONE',  ( -0.000000000000000000, -0.000000000000000000, 1.000000000000000000 ) ) ;
#23054=CARTESIAN_POINT ( 'NONE',  ( 53.97939423941235049, -4.961365878511737826, -10.19931710281307247 ) ) ;
#23055=ORIENTED_EDGE ( 'NONE', *, *, #22117, .F. ) ;
#23059=AXIS2_PLACEMENT_3D ( 'NONE', #15062, #5053, #11943 ) ;
#23064=CIRCLE ( 'NONE', #7898, 67.32891250266496286 ) ;
#23068=CARTESIAN_POINT ( 'NONE',  ( -9.813471072924700778, -5.936918610400975460, 107.7389212035124046 ) ) ;
#23077=CARTESIAN_POINT ( 'NONE',  ( -34.85155852797733189, -3.604462483032124354, 80.65629953933577667 ) ) ;
#23091=DIRECTION ( 'NONE',  ( 0.000000000000000000, 0.000000000000000000, 1.000000000000000000 ) ) ;
#23103=CARTESIAN_POINT ( 'NONE',  ( -5.930220226013869222, 9.437824910247670118, 98.40971065117005878 ) ) ;
#23105=ORIENTED_EDGE ( 'NONE', *, *, #8844, .F. ) ;
#23127=CARTESIAN_POINT ( 'NONE',  ( 49.03637579218595732, 8.583949016299408541, 98.45931519117756636 ) ) ;
#23131=CARTESIAN_POINT ( 'NONE',  ( -2.057288477451015840, 11.55930814891847902, -4.886607555839500350 ) ) ;
#23145=VERTEX_POINT ( 'NONE', #25259 ) ;
#23148=ORIENTED_EDGE ( 'NONE', *, *, #3517, .F. ) ;
#23156=CARTESIAN_POINT ( 'NONE',  ( 21.09785597605719332, 12.78350261226561280, 47.04930799450051637 ) ) ;
#23158=CARTESIAN_POINT ( 'NONE',  ( 21.09785597605719332, -16.43042895458278352, 47.04930799450051637 ) ) ;
#23169=CARTESIAN_POINT ( 'NONE',  ( 47.79865503179234310, 9.702389020015065313, -4.315940132965163656 ) ) ;
#23180=ORIENTED_EDGE ( 'NONE', *, *, #4530, .F. ) ;
#23182=DIRECTION ( 'NONE',  ( -0.000000000000000000, 1.000000000000000000, -0.000000000000000000 ) ) ;
#23186=CARTESIAN_POINT ( 'NONE',  ( -34.71505847545616064, 11.47745911305554145, 52.78077050074096377 ) ) ;
#23187=VECTOR ( 'NONE', #4073, 1000.000000000000000 ) ;
#23192=EDGE_LOOP ( 'NONE', ( #28651, #27285 ) ) ;
#23194=CARTESIAN_POINT ( 'NONE',  ( 21.09785597605719332, 11.92558985988973497, 47.04930799450051637 ) ) ;
#23208=LINE ( 'NONE', #30446, #21211 ) ;
#23223=CARTESIAN_POINT ( 'NONE',  ( 49.86503751672583462, 7.651854857429027490, -4.493960750487066669 ) ) ;
#23226=B_SPLINE_SURFACE_WITH_KNOTS ( 'NONE', 3, 1, ( 
 ( #20770, #30786 ),
 ( #28004, #20442 ),
 ( #25700, #30475 ),
 ( #17983, #13077 ) ),
 .UNSPECIFIED., .F., .F., .F.,
 ( 4, 4 ),
 ( 2, 2 ),
 ( 0.9911194921636323762, 1.000000000000000000 ),
 ( 0.000000000000000000, 1.000000000000000000 ),
 .UNSPECIFIED. ) ;
#23236=DIRECTION ( 'NONE',  ( 1.000000000000000000, 0.000000000000000000, 2.775557561562888984E-15 ) ) ;
#23237=CARTESIAN_POINT ( 'NONE',  ( -4.902144023942810236, 25.56454579224779877, 44.54930799450078638 ) ) ;
#23239=CARTESIAN_POINT ( 'NONE',  ( -34.71177954129748855, 11.48555665516351354, 41.32782006312588408 ) ) ;
#23244=CARTESIAN_POINT ( 'NONE',  ( -33.46773820220050766, -1.490757911476732867, 80.67629718822401230 ) ) ;
#23257=DIRECTION ( 'NONE',  ( 0.000000000000000000, 0.000000000000000000, -1.000000000000000000 ) ) ;
#23266=VERTEX_POINT ( 'NONE', #15894 ) ;
#23269=CARTESIAN_POINT ( 'NONE',  ( -6.842391073119661549, 8.582373042058234702, 98.45937169672181710 ) ) ;
#23271=EDGE_CURVE ( 'NONE', #31078, #29942, #946, .T. ) ;
#23273=B_SPLINE_CURVE_WITH_KNOTS ( 'NONE', 3,
 ( #31115, #13399, #3854, #23395, #20769, #902, #3689, #5848, #15851, #8464, #16005, #28487, #28804, #18615, #1220, #16318, #21238, #31271, #26987, #4503, #6479, #31754, #19430, #9268, #19257, #26656, #7132, #2207, #32082, #24516, #31916, #12058, #9103, #14689, #14521, #27144, #24196, #17126, #19093, #22054, #29130, #1716, #14030, #26825, #9596, #24030, #2039, #19593 ),
 .UNSPECIFIED., .F., .F.,
 ( 4, 2, 2, 2, 2, 2, 2, 2, 2, 2, 2, 2, 2, 2, 2, 2, 2, 2, 2, 2, 2, 2, 2, 4 ),
 ( 0.000000000000000000, 0.0008877576229114608882, 0.001331636434367201687, 0.001775515245822942376, 0.002663272868734409878, 0.003551030491645877380, 0.004438788114557345316, 0.005326545737468812818, 0.006214303360380279452, 0.007102060983291746954, 0.008877576229114671549, 0.009765333852026134714, 0.01065309147493759788, 0.01242860672076051554, 0.01420412196658343493, 0.01597963721240634738, 0.01775515245822926677, 0.01953066770405217922, 0.02130618294987509861, 0.02308169819569801107, 0.02396945581860946903, 0.02485721344152092699, 0.02663272868734380475, 0.02840824393316667903 ),
 .UNSPECIFIED. ) ;
#23274=EDGE_CURVE ( 'NONE', #23145, #22133, #3076, .T. ) ;
#23286=EDGE_LOOP ( 'NONE', ( #203, #7448, #18774, #12994, #2667, #15360 ) ) ;
#23290=CARTESIAN_POINT ( 'NONE',  ( 42.60875976922299202, 11.86909835304794569, 99.49998532334635115 ) ) ;
#23293=LINE ( 'NONE', #6060, #1623 ) ;
#23296=VERTEX_POINT ( 'NONE', #11929 ) ;
#23314=AXIS2_PLACEMENT_3D ( 'NONE', #999, #21010, #25624 ) ;
#23322=DIRECTION ( 'NONE',  ( -0.000000000000000000, -1.000000000000000000, -0.000000000000000000 ) ) ;
#23325=CARTESIAN_POINT ( 'NONE',  ( 21.09785597605719332, 25.56454579224779877, 21.04930799450051282 ) ) ;
#23326=CARTESIAN_POINT ( 'NONE',  ( -37.74053575120161952, -5.821578765910089714, 78.65578092815914601 ) ) ;
#23331=DIRECTION ( 'NONE',  ( 0.000000000000000000, -1.000000000000000000, 0.000000000000000000 ) ) ;
#23337=CIRCLE ( 'NONE', #11289, 2.500000000000002220 ) ;
#23348=CARTESIAN_POINT ( 'NONE',  ( -39.46892853597984896, -5.935610090285465823, 77.88162228658642050 ) ) ;
#23350=B_SPLINE_CURVE_WITH_KNOTS ( 'NONE', 3,
 ( #10466, #17999, #10793, #28020, #20136, #30652, #2747, #25550, #7838, #10635, #20626, #20786 ),
 .UNSPECIFIED., .F., .F.,
 ( 4, 2, 2, 2, 2, 4 ),
 ( 0.000000000000000000, 7.696047042371321643E-05, 0.0001154407056355867789, 0.0001539209408474603413, 0.0002308814112711852671, 0.0003078418816949101658 ),
 .UNSPECIFIED. ) ;
#23355=VERTEX_POINT ( 'NONE', #6362 ) ;
#23358=DIRECTION ( 'NONE',  ( 0.000000000000000000, -1.251509963831984395E-16, 1.000000000000000000 ) ) ;
#23366=CARTESIAN_POINT ( 'NONE',  ( -5.602943079677954685, 9.702389020015065313, -3.412202488244239884 ) ) ;
#23367=( NAMED_UNIT ( * ) SI_UNIT ( $, .STERADIAN. ) SOLID_ANGLE_UNIT ( ) );
#23379=ORIENTED_EDGE ( 'NONE', *, *, #25498, .T. ) ;
#23381=DIRECTION ( 'NONE',  ( -0.000000000000000000, 1.000000000000000000, -0.000000000000000000 ) ) ;
#23391=EDGE_CURVE ( 'NONE', #31626, #6406, #22501, .T. ) ;
#23395=CARTESIAN_POINT ( 'NONE',  ( -36.43076496478325765, -5.790431667319170472, 78.73662387569818577 ) ) ;
#23398=CARTESIAN_POINT ( 'NONE',  ( -34.33782038214594223, 11.92558985988973497, 40.19271875144398365 ) ) ;
#23399=VERTEX_POINT ( 'NONE', #21605 ) ;
#23400=CARTESIAN_POINT ( 'NONE',  ( -7.324817582041172948, 8.310461108307681144, 106.8025418868326284 ) ) ;
#23402=CARTESIAN_POINT ( 'NONE',  ( -31.01600359787390815, 11.71173593729433016, 69.58946823766353873 ) ) ;
#23407=FACE_OUTER_BOUND ( 'NONE', #14495, .T. ) ;
#23408=CARTESIAN_POINT ( 'NONE',  ( 21.09785597605719332, 24.86454579224780304, 67.04930799450050927 ) ) ;
#23411=EDGE_LOOP ( 'NONE', ( #14232, #28941 ) ) ;
#23422=EDGE_CURVE ( 'NONE', #20095, #12308, #25963, .T. ) ;
#23423=EDGE_CURVE ( 'NONE', #4546, #9438, #25564, .T. ) ;
#23424=CIRCLE ( 'NONE', #28666, 55.53141649511111666 ) ;
#23428=CARTESIAN_POINT ( 'NONE',  ( -12.43472240872365475, -3.866180060838604771, 103.2125413378014258 ) ) ;
#23444=ORIENTED_EDGE ( 'NONE', *, *, #18227, .F. ) ;
#23446=CARTESIAN_POINT ( 'NONE',  ( 42.05878518372482233, 11.91444431924556469, 99.69513167491371064 ) ) ;
#23447=CARTESIAN_POINT ( 'NONE',  ( 54.52425928046186954, -0.6709275202869728894, 101.2046830443633354 ) ) ;
#23449=CARTESIAN_POINT ( 'NONE',  ( 21.09785597605719332, 25.56454579224779877, 21.04930799450051282 ) ) ;
#23455=DIRECTION ( 'NONE',  ( 1.000000000000000000, -0.000000000000000000, -0.000000000000000000 ) ) ;
#23459=EDGE_CURVE ( 'NONE', #3218, #17109, #28283, .T. ) ;
#23463=VERTEX_POINT ( 'NONE', #12761 ) ;
#23468=EDGE_CURVE ( 'NONE', #3078, #2614, #10999, .T. ) ;
#23472=CARTESIAN_POINT ( 'NONE',  ( 21.09785597605719332, -16.93042895458276575, -37.45571725866892621 ) ) ;
#23478=CARTESIAN_POINT ( 'NONE',  ( 81.60586963689938500, -5.935454207752203892, 16.07118271501079576 ) ) ;
#23496=CARTESIAN_POINT ( 'NONE',  ( 53.90149697474231516, 0.9814505390143266617, 99.57122575047146995 ) ) ;
#23505=FACE_OUTER_BOUND ( 'NONE', #10275, .T. ) ;
#23510=CARTESIAN_POINT ( 'NONE',  ( 51.99726271649544884, -5.936960083300405699, -13.64809480703120137 ) ) ;
#23512=ORIENTED_EDGE ( 'NONE', *, *, #18729, .F. ) ;
#23528=CARTESIAN_POINT ( 'NONE',  ( 21.09785597605719332, 13.74476430820393347, 47.04930799450051637 ) ) ;
#23529=ADVANCED_FACE ( 'NONE', ( #28645 ), #18224, .F. ) ;
#23540=DIRECTION ( 'NONE',  ( -1.000000000000000000, 0.000000000000000000, 0.000000000000000000 ) ) ;
#23545=ORIENTED_EDGE ( 'NONE', *, *, #18120, .T. ) ;
#23569=DIRECTION ( 'NONE',  ( 0.000000000000000000, 1.000000000000000000, 1.446921688628131436E-16 ) ) ;
#23572=EDGE_CURVE ( 'NONE', #29304, #7835, #24593, .T. ) ;
#23575=ORIENTED_EDGE ( 'NONE', *, *, #13179, .T. ) ;
#23579=ORIENTED_EDGE ( 'NONE', *, *, #10165, .T. ) ;
#23593=CARTESIAN_POINT ( 'NONE',  ( 80.77181806311266143, 9.702389020015065313, 20.34850893876557976 ) ) ;
#23611=EDGE_CURVE ( 'NONE', #30294, #3737, #14133, .T. ) ;
#23618=CARTESIAN_POINT ( 'NONE',  ( -36.24635750042178728, -5.700102882051749198, 15.13141875408116022 ) ) ;
#23622=PLANE ( 'NONE',  #21427 ) ;
#23637=CARTESIAN_POINT ( 'NONE',  ( -35.12632216515691397, 11.92558985988973674, 54.04930799450053769 ) ) ;
#23644=ORIENTED_EDGE ( 'NONE', *, *, #8418, .F. ) ;
#23647=LINE ( 'NONE', #9147, #24358 ) ;
#23674=CARTESIAN_POINT ( 'NONE',  ( -36.45222641229887017, 9.925589859889724309, 52.04930799450051637 ) ) ;
#23676=FACE_OUTER_BOUND ( 'NONE', #22799, .T. ) ;
#23696=AXIS2_PLACEMENT_3D ( 'NONE', #26638, #4322, #23852 ) ;
#23699=DIRECTION ( 'NONE',  ( 0.000000000000000000, 0.000000000000000000, -1.000000000000000000 ) ) ;
#23704=CARTESIAN_POINT ( 'NONE',  ( 54.75611978667879498, -3.386628651588837524, -8.728176170384978505 ) ) ;
#23719=EDGE_LOOP ( 'NONE', ( #26829, #27876, #6988, #719 ) ) ;
#23722=CARTESIAN_POINT ( 'NONE',  ( 21.09785597605719332, -5.986312001189870280, -20.31486511684159879 ) ) ;
#23738=CARTESIAN_POINT ( 'NONE',  ( -43.62623615455565584, -4.423456490293570020, 42.00470062833824869 ) ) ;
#23754=VECTOR ( 'NONE', #14745, 1000.000000000000000 ) ;
#23762=FACE_OUTER_BOUND ( 'NONE', #17939, .T. ) ;
#23766=CARTESIAN_POINT ( 'NONE',  ( 100.3079064823960493, -15.93545420775219945, 47.04930799450134771 ) ) ;
#23768=VERTEX_POINT ( 'NONE', #18940 ) ;
#23773=FACE_BOUND ( 'NONE', #5883, .T. ) ;
#23775=ORIENTED_EDGE ( 'NONE', *, *, #31104, .F. ) ;
#23780=CIRCLE ( 'NONE', #31636, 2.500000000000002220 ) ;
#23781=ORIENTED_EDGE ( 'NONE', *, *, #18045, .F. ) ;
#23793=CARTESIAN_POINT ( 'NONE',  ( -63.90214402394282445, 9.925589859889724309, 52.04930799450051637 ) ) ;
#23794=CARTESIAN_POINT ( 'NONE',  ( -35.27310491972505702, 11.80858882337094329, 40.73717082040712256 ) ) ;
#23799=DIRECTION ( 'NONE',  ( 0.000000000000000000, 0.000000000000000000, -1.000000000000000000 ) ) ;
#23807=CARTESIAN_POINT ( 'NONE',  ( -9.869916472764515447, -5.940946157296537855, 106.6954391641310309 ) ) ;
#23824=CARTESIAN_POINT ( 'NONE',  ( 106.0978559760574313, 11.92558985988973497, 67.46350265493050813 ) ) ;
#23829=ORIENTED_EDGE ( 'NONE', *, *, #5126, .F. ) ;
#23839=VECTOR ( 'NONE', #2334, 1000.000000000000000 ) ;
#23840=ORIENTED_EDGE ( 'NONE', *, *, #8021, .F. ) ;
#23852=DIRECTION ( 'NONE',  ( 0.000000000000000000, 0.000000000000000000, 1.000000000000000000 ) ) ;
#23868=EDGE_CURVE ( 'NONE', #18864, #19298, #26733, .T. ) ;
#23883=ORIENTED_EDGE ( 'NONE', *, *, #14234, .F. ) ;
#23884=LINE ( 'NONE', #8477, #29102 ) ;
#23889=CARTESIAN_POINT ( 'NONE',  ( 21.09785597605719332, -6.314304012688826795, 47.04930799450051637 ) ) ;
#23894=CARTESIAN_POINT ( 'NONE',  ( 21.09785597605719332, 14.77459629858661572, 47.04930799450051637 ) ) ;
#23898=EDGE_LOOP ( 'NONE', ( #11598, #21537, #16164, #336 ) ) ;
#23919=ORIENTED_EDGE ( 'NONE', *, *, #7272, .F. ) ;
#23920=CARTESIAN_POINT ( 'NONE',  ( -11.87053376181319386, 0.6013300790671924911, -5.618057101110695228 ) ) ;
#23930=ORIENTED_EDGE ( 'NONE', *, *, #7415, .F. ) ;
#23939=ORIENTED_EDGE ( 'NONE', *, *, #25011, .T. ) ;
#23943=CARTESIAN_POINT ( 'NONE',  ( 100.3079064823960493, 25.56454579224780232, 44.54930799450134771 ) ) ;
#23944=AXIS2_PLACEMENT_3D ( 'NONE', #7187, #21946, #19812 ) ;
#23953=CARTESIAN_POINT ( 'NONE',  ( 77.22212800161737789, -3.812314126620147459, 13.51013469878526152 ) ) ;
#23954=CIRCLE ( 'NONE', #9828, 54.21005050633881694 ) ;
#23973=CARTESIAN_POINT ( 'NONE',  ( 21.09785597605719332, -16.63545420775219696, 47.04930799450051637 ) ) ;
#23976=VERTEX_POINT ( 'NONE', #8590 ) ;
#23993=B_SPLINE_CURVE_WITH_KNOTS ( 'NONE', 3,
 ( #19036, #23807, #16578, #4282, #16261, #4108, #1009, #3632 ),
 .UNSPECIFIED., .F., .F.,
 ( 4, 2, 2, 4 ),
 ( 6.938893903907228378E-18, 0.0004427811193176627936, 0.0008855622386353186482, 0.001771124477270593061 ),
 .UNSPECIFIED. ) ;
#24006=AXIS2_PLACEMENT_3D ( 'NONE', #4806, #25317, #48 ) ;
#24009=EDGE_LOOP ( 'NONE', ( #6971, #30255, #21945, #3232 ) ) ;
#24010=CARTESIAN_POINT ( 'NONE',  ( -39.57300472050416573, -5.936086065851251092, 77.91551484630795699 ) ) ;
#24013=VECTOR ( 'NONE', #3550, 1000.000000000000000 ) ;
#24014=ORIENTED_EDGE ( 'NONE', *, *, #23271, .F. ) ;
#24016=EDGE_CURVE ( 'NONE', #11676, #13013, #3124, .T. ) ;
#24019=CIRCLE ( 'NONE', #28731, 39.93581437244897359 ) ;
#24025=ADVANCED_FACE ( 'NONE', ( #18581 ), #10583, .F. ) ;
#24030=CARTESIAN_POINT ( 'NONE',  ( -30.46736936537216067, 11.87712387757214927, 68.60098163695475648 ) ) ;
#24035=TOROIDAL_SURFACE ( 'NONE', #458, 67.99999999999997158, 4.000000000000000000 ) ;
#24040=CARTESIAN_POINT ( 'NONE',  ( 21.09785597605719332, 12.06852548259731961, 47.04930799450051637 ) ) ;
#24042=LINE ( 'NONE', #31924, #30685 ) ;
#24061=AXIS2_PLACEMENT_3D ( 'NONE', #15426, #167, #30209 ) ;
#24069=ORIENTED_EDGE ( 'NONE', *, *, #12826, .F. ) ;
#24072=DIRECTION ( 'NONE',  ( 0.000000000000000000, 0.000000000000000000, -1.000000000000000000 ) ) ;
#24080=CARTESIAN_POINT ( 'NONE',  ( 21.09785597605719332, 13.74476430820393347, 103.0493079945005093 ) ) ;
#24086=FACE_OUTER_BOUND ( 'NONE', #10153, .T. ) ;
#24096=DIRECTION ( 'NONE',  ( 0.000000000000000000, 0.000000000000000000, -1.000000000000000000 ) ) ;
#24103=AXIS2_PLACEMENT_3D ( 'NONE', #25976, #3486, #13999 ) ;
#24119=DIRECTION ( 'NONE',  ( 0.000000000000000000, 0.000000000000000000, -1.000000000000000000 ) ) ;
#24120=CARTESIAN_POINT ( 'NONE',  ( 77.08942877945061412, -3.654479441960591490, 13.45888422241439919 ) ) ;
#24134=FACE_BOUND ( 'NONE', #31549, .T. ) ;
#24149=CYLINDRICAL_SURFACE ( 'NONE', #14171, 2.000000000000001776 ) ;
#24159=CARTESIAN_POINT ( 'NONE',  ( 53.00177451235461490, 2.793366809690220887, -4.849114461849969082 ) ) ;
#24160=TOROIDAL_SURFACE ( 'NONE', #11596, 48.97546517713167447, 2.000000000000000000 ) ;
#24164=DIRECTION ( 'NONE',  ( -0.000000000000000000, -1.000000000000000000, -0.000000000000000000 ) ) ;
#24178=CARTESIAN_POINT ( 'NONE',  ( 21.09785597605720042, 24.74924423484549507, 86.98512236694949706 ) ) ;
#24179=LINE ( 'NONE', #8759, #22517 ) ;
#24180=CARTESIAN_POINT ( 'NONE',  ( 53.16169625780806740, -5.983766253076982622, 106.7232700815558957 ) ) ;
#24192=EDGE_CURVE ( 'NONE', #8696, #9808, #14185, .T. ) ;
#24195=CARTESIAN_POINT ( 'NONE',  ( 21.09785597605719687, 15.63322284159649556, 94.10733885242261465 ) ) ;
#24196=CARTESIAN_POINT ( 'NONE',  ( -29.34961020680567501, 9.276496357494197653, 74.28030578752274948 ) ) ;
#24202=ORIENTED_EDGE ( 'NONE', *, *, #10127, .T. ) ;
#24222=ORIENTED_EDGE ( 'NONE', *, *, #9635, .T. ) ;
#24223=CARTESIAN_POINT ( 'NONE',  ( -43.86787645162945637, -4.885237077964406538, 41.81402935846817570 ) ) ;
#24234=ORIENTED_EDGE ( 'NONE', *, *, #3520, .F. ) ;
#24244=CARTESIAN_POINT ( 'NONE',  ( -9.880269303432738681, -5.935454207752202116, -10.95525492004900769 ) ) ;
#24248=DIRECTION ( 'NONE',  ( -0.000000000000000000, -1.000000000000000000, -0.000000000000000000 ) ) ;
#24262=CARTESIAN_POINT ( 'NONE',  ( -38.57628410747783221, 11.23353061944650655, 22.24400271019782593 ) ) ;
#24268=EDGE_CURVE ( 'NONE', #29214, #2165, #26211, .T. ) ;
#24270=ADVANCED_FACE ( 'NONE', ( #15137 ), #25, .F. ) ;
#24284=CARTESIAN_POINT ( 'NONE',  ( 72.92745752893763722, 6.334306897662558278, 17.30572780667399968 ) ) ;
#24292=ADVANCED_FACE ( 'NONE', ( #12522 ), #17096, .F. ) ;
#24297=EDGE_CURVE ( 'NONE', #12758, #3218, #6840, .T. ) ;
#24302=CARTESIAN_POINT ( 'NONE',  ( -12.57422076041892645, -1.761407059904331218, -7.664706412628855325 ) ) ;
#24330=VERTEX_POINT ( 'NONE', #12189 ) ;
#24339=AXIS2_PLACEMENT_3D ( 'NONE', #4306, #9067, #14323 ) ;
#24340=CARTESIAN_POINT ( 'NONE',  ( 21.09785597605719332, -16.63545420775219696, -32.16074251183835031 ) ) ;
#24342=CARTESIAN_POINT ( 'NONE',  ( 47.79865503179234310, 9.702389020015065313, 106.7232700815558957 ) ) ;
#24350=CARTESIAN_POINT ( 'NONE',  ( 52.16615856333482526, -5.937394852768787423, 107.4212530892143889 ) ) ;
#24356=CONICAL_SURFACE ( 'NONE', #23314, 54.55130244989821620, 1.291543646475813212 ) ;
#24358=VECTOR ( 'NONE', #21771, 1000.000000000000000 ) ;
#24363=CIRCLE ( 'NONE', #32240, 84.30000000000001137 ) ;
#24367=EDGE_LOOP ( 'NONE', ( #845, #2713 ) ) ;
#24368=DIRECTION ( 'NONE',  ( 0.000000000000000000, 0.000000000000000000, -1.000000000000000000 ) ) ;
#24370=DIRECTION ( 'NONE',  ( -0.000000000000000000, -1.000000000000000000, -0.000000000000000000 ) ) ;
#24377=CARTESIAN_POINT ( 'NONE',  ( 21.09785597605719332, -6.659195188345857552, 47.04930799450051637 ) ) ;
#24381=ORIENTED_EDGE ( 'NONE', *, *, #7538, .F. ) ;
#24391=ORIENTED_EDGE ( 'NONE', *, *, #24268, .T. ) ;
#24392=EDGE_CURVE ( 'NONE', #30056, #5110, #10710, .T. ) ;
#24402=ORIENTED_EDGE ( 'NONE', *, *, #18960, .F. ) ;
#24403=CARTESIAN_POINT ( 'NONE',  ( -38.59984781516420327, -5.935454207752198563, 77.87546120947918382 ) ) ;
#24409=CARTESIAN_POINT ( 'NONE',  ( 81.54161849434414933, -5.935454207752202116, 77.87546120947918382 ) ) ;
#24423=CARTESIAN_POINT ( 'NONE',  ( -29.27337757263006424, 8.768497289655476479, 19.08884019352816352 ) ) ;
#24425=ORIENTED_EDGE ( 'NONE', *, *, #15677, .T. ) ;
#24428=ADVANCED_FACE ( 'NONE', ( #30238 ), #681, .F. ) ;
#24434=CARTESIAN_POINT ( 'NONE',  ( 52.00224528769592780, -5.936959954202218448, -13.39898132534822395 ) ) ;
#24438=EDGE_LOOP ( 'NONE', ( #16506, #17214, #13744, #3878, #10698 ) ) ;
#24461=CARTESIAN_POINT ( 'NONE',  ( -6.840663840071563584, 8.583949016299408541, -4.360699202176528289 ) ) ;
#24467=AXIS2_PLACEMENT_3D ( 'NONE', #12648, #22143, #17059 ) ;
#24472=CIRCLE ( 'NONE', #20805, 67.18681090792858868 ) ;
#24479=CARTESIAN_POINT ( 'NONE',  ( 54.58813758245922543, -3.977894809549914257, -8.278115739697286202 ) ) ;
#24481=DIRECTION ( 'NONE',  ( -0.000000000000000000, 1.000000000000000000, -0.000000000000000000 ) ) ;
#24486=DIRECTION ( 'NONE',  ( 0.000000000000000000, 0.000000000000000000, -1.000000000000000000 ) ) ;
#24487=B_SPLINE_SURFACE_WITH_KNOTS ( 'NONE', 3, 1, ( 
 ( #5135, #27124 ),
 ( #19896, #22690 ),
 ( #9740, #7443 ),
 ( #4642, #12703 ),
 ( #19730, #14663 ),
 ( #24494, #17437 ) ),
 .UNSPECIFIED., .F., .F., .F.,
 ( 4, 1, 1, 4 ),
 ( 2, 2 ),
 ( 0.1800733115436725096, 0.3950736110976382220, 0.6810807126490734387, 1.000000000000000000 ),
 ( 0.000000000000000000, 1.000000000000000000 ),
 .UNSPECIFIED. ) ;
#24492=CARTESIAN_POINT ( 'NONE',  ( -29.53813221254135968, 7.610385968504705723, 18.25503064196351843 ) ) ;
#24494=CARTESIAN_POINT ( 'NONE',  ( 80.85108986838919520, 9.702389020015065313, 73.75010705023588287 ) ) ;
#24495=ORIENTED_EDGE ( 'NONE', *, *, #10165, .F. ) ;
#24505=CARTESIAN_POINT ( 'NONE',  ( 56.35714053840848692, -3.295808585244882849, 97.45038561958638468 ) ) ;
#24507=CARTESIAN_POINT ( 'NONE',  ( 72.15675507252800003, 11.55977609614115664, 23.89582598614757103 ) ) ;
#24512=ADVANCED_FACE ( 'NONE', ( #7749 ), #14718, .T. ) ;
#24516=CARTESIAN_POINT ( 'NONE',  ( -30.22711675696656286, 4.712813290757158491, 77.84736881414806930 ) ) ;
#24520=ADVANCED_FACE ( 'NONE', ( #17748 ), #8081, .F. ) ;
#24529=EDGE_LOOP ( 'NONE', ( #1689, #7582, #6321, #3281 ) ) ;
#24540=DIRECTION ( 'NONE',  ( -0.000000000000000000, -1.000000000000000000, -0.000000000000000000 ) ) ;
#24542=CARTESIAN_POINT ( 'NONE',  ( -45.72330504332160217, -5.935454207752198563, 54.04930799450053058 ) ) ;
#24543=CARTESIAN_POINT ( 'NONE',  ( 21.09785597605720397, -15.93545420775219945, 119.5493079945004808 ) ) ;
#24552=CARTESIAN_POINT ( 'NONE',  ( 21.09785597605719332, 14.86454579224779771, 47.04930799450051637 ) ) ;
#24554=ORIENTED_EDGE ( 'NONE', *, *, #19749, .T. ) ;
#24559=CARTESIAN_POINT ( 'NONE',  ( 21.09785597605719332, -19.93545420775220123, 131.3493079945005491 ) ) ;
#24564=CARTESIAN_POINT ( 'NONE',  ( 21.09785597605720042, 15.56454579224779877, 96.02477317163219084 ) ) ;
#24566=CARTESIAN_POINT ( 'NONE',  ( 21.09785597605719332, 11.92558985988973497, 47.04930799450051637 ) ) ;
#24568=CARTESIAN_POINT ( 'NONE',  ( -8.545635354592475252, 6.496515553941723198, -3.810470283972227978 ) ) ;
#24570=ORIENTED_EDGE ( 'NONE', *, *, #20800, .F. ) ;
#24581=ORIENTED_EDGE ( 'NONE', *, *, #17570, .T. ) ;
#24593=CIRCLE ( 'NONE', #25653, 1.000000000000000000 ) ;
#24598=CARTESIAN_POINT ( 'NONE',  ( 51.92400919103563695, -5.935454207752202116, -12.70392589783158499 ) ) ;
#24600=CIRCLE ( 'NONE', #11003, 56.65825807113184709 ) ;
#24620=ORIENTED_EDGE ( 'NONE', *, *, #14901, .T. ) ;
#24622=CARTESIAN_POINT ( 'NONE',  ( 100.3079064823960493, -16.63545420775219696, 47.04930799450134771 ) ) ;
#24625=CARTESIAN_POINT ( 'NONE',  ( 21.09785597605719332, -16.63545420775219696, 128.7593585008393973 ) ) ;
#24627=CARTESIAN_POINT ( 'NONE',  ( -10.54383519688239090, 3.260977705924062775, -5.641619965526164293 ) ) ;
#24635=VECTOR ( 'NONE', #17427, 1000.000000000000000 ) ;
#24645=AXIS2_PLACEMENT_3D ( 'NONE', #27114, #17589, #4631 ) ;
#24653=DIRECTION ( 'NONE',  ( 0.000000000000000000, -1.000000000000000000, 0.000000000000000000 ) ) ;
#24664=AXIS2_PLACEMENT_3D ( 'NONE', #23894, #31291, #4032 ) ;
#24666=CARTESIAN_POINT ( 'NONE',  ( -30.07837276871502752, 5.259395908821971055, 16.59273893179034332 ) ) ;
#24677=CARTESIAN_POINT ( 'NONE',  ( -9.472371843582571671, 5.388785998227650254, -12.62465409255485582 ) ) ;
#24686=ADVANCED_FACE ( 'NONE', ( #30166 ), #24909, .T. ) ;
#24688=AXIS2_PLACEMENT_3D ( 'NONE', #4624, #29743, #12184 ) ;
#24698=ORIENTED_EDGE ( 'NONE', *, *, #21763, .T. ) ;
#24706=DIRECTION ( 'NONE',  ( 0.000000000000000000, -1.000000000000000000, 0.000000000000000000 ) ) ;
#24707=ORIENTED_EDGE ( 'NONE', *, *, #23391, .T. ) ;
#24710=LINE ( 'NONE', #17802, #20109 ) ;
#24714=DIRECTION ( 'NONE',  ( 1.000000000000000000, -0.000000000000000000, -0.000000000000000000 ) ) ;
#24738=CARTESIAN_POINT ( 'NONE',  ( -30.57062045089658753, 7.039311848382081571, 17.81148138227357336 ) ) ;
#24752=CARTESIAN_POINT ( 'NONE',  ( -38.52112853513683888, -5.935454207752202116, 16.07118271501078510 ) ) ;
#24756=CARTESIAN_POINT ( 'NONE',  ( -29.27337757263006424, -5.432165593243111879, 14.50875660354866703 ) ) ;
#24760=CARTESIAN_POINT ( 'NONE',  ( 21.09785597605719332, 25.56454579224779877, 18.54930799450050927 ) ) ;
#24767=CARTESIAN_POINT ( 'NONE',  ( 52.07152283844947505, -5.935708903123431135, -13.42846411458451428 ) ) ;
#24771=AXIS2_PLACEMENT_3D ( 'NONE', #20267, #27662, #7807 ) ;
#24792=CARTESIAN_POINT ( 'NONE',  ( 21.09785597605719332, 25.56454579224779877, 70.54930799450050927 ) ) ;
#24809=DIRECTION ( 'NONE',  ( 0.000000000000000000, 0.000000000000000000, 1.000000000000000000 ) ) ;
#24822=CARTESIAN_POINT ( 'NONE',  ( 21.09785597605719332, 11.92558985988973497, 47.04930799450051637 ) ) ;
#24829=ADVANCED_FACE ( 'NONE', ( #9592 ), #30295, .F. ) ;
#24836=DIRECTION ( 'NONE',  ( 0.000000000000000000, 0.000000000000000000, -1.000000000000000000 ) ) ;
#24853=DIRECTION ( 'NONE',  ( -0.000000000000000000, -1.000000000000000000, -0.000000000000000000 ) ) ;
#24863=CARTESIAN_POINT ( 'NONE',  ( 71.55936645880184699, 9.702389020015065313, 73.75010705023584023 ) ) ;
#24866=CARTESIAN_POINT ( 'NONE',  ( 72.25012468985910630, 5.370505999354230120, 77.42531960576580730 ) ) ;
#24869=VECTOR ( 'NONE', #11368, 1000.000000000000000 ) ;
#24871=FACE_OUTER_BOUND ( 'NONE', #8693, .T. ) ;
#24874=DIRECTION ( 'NONE',  ( 0.000000000000000000, 0.000000000000000000, -1.000000000000000000 ) ) ;
#24884=ADVANCED_FACE ( 'NONE', ( #4167 ), #18910, .T. ) ;
#24885=ORIENTED_EDGE ( 'NONE', *, *, #3394, .T. ) ;
#24897=CARTESIAN_POINT ( 'NONE',  ( -44.25434836777630210, -5.709091131881068648, 53.11493085759866517 ) ) ;
#24904=CARTESIAN_POINT ( 'NONE',  ( -33.35089495028901041, -1.269481974065232555, 13.46653852984619348 ) ) ;
#24905=CARTESIAN_POINT ( 'NONE',  ( -5.948280841129993668, 9.423225080673429233, -3.404543741840068805 ) ) ;
#24909=CYLINDRICAL_SURFACE ( 'NONE', #1099, 55.00000000000000000 ) ;
#24921=CARTESIAN_POINT ( 'NONE',  ( -39.02270572350619915, 5.305725667695960546, 52.04930799450051637 ) ) ;
#24923=VERTEX_POINT ( 'NONE', #22183 ) ;
#24934=CARTESIAN_POINT ( 'NONE',  ( 51.92400919103563695, -5.935454207752202116, -3.337848843846767721 ) ) ;
#24936=CIRCLE ( 'NONE', #3886, 2.500000000000002220 ) ;
#24948=DIRECTION ( 'NONE',  ( 0.000000000000000000, -1.000000000000000000, 0.000000000000000000 ) ) ;
#24954=ORIENTED_EDGE ( 'NONE', *, *, #23572, .F. ) ;
#24958=VERTEX_POINT ( 'NONE', #12022 ) ;
#24961=CARTESIAN_POINT ( 'NONE',  ( 21.09785597605719332, 12.78350261226561280, -8.675054649682497399 ) ) ;
#24968=CARTESIAN_POINT ( 'NONE',  ( 21.09785597605719332, -15.93545420775219945, 47.04930799450051637 ) ) ;
#24972=DIRECTION ( 'NONE',  ( 0.000000000000000000, 0.000000000000000000, -1.000000000000000000 ) ) ;
#24976=DIRECTION ( 'NONE',  ( 0.000000000000000000, -0.000000000000000000, -1.000000000000000000 ) ) ;
#24989=ORIENTED_EDGE ( 'NONE', *, *, #9337, .F. ) ;
#24993=CARTESIAN_POINT ( 'NONE',  ( -35.11018699695847545, -4.854904164370157815, 14.08771498410514234 ) ) ;
#25001=ORIENTED_EDGE ( 'NONE', *, *, #782, .F. ) ;
#25004=CARTESIAN_POINT ( 'NONE',  ( -58.11219453028166981, 25.56454579224780232, 49.54930799450023926 ) ) ;
#25011=EDGE_CURVE ( 'NONE', #30056, #2086, #14230, .T. ) ;
#25014=DIRECTION ( 'NONE',  ( 5.937205496305277864E-17, -0.8746197071393925215, 0.4848096202463429982 ) ) ;
#25033=DIRECTION ( 'NONE',  ( 0.000000000000000000, -0.8746197071393925215, -0.4848096202463429982 ) ) ;
#25042=ORIENTED_EDGE ( 'NONE', *, *, #15716, .F. ) ;
#25045=EDGE_CURVE ( 'NONE', #29763, #8194, #32055, .T. ) ;
#25052=AXIS2_PLACEMENT_3D ( 'NONE', #10777, #8620, #28329 ) ;
#25054=CARTESIAN_POINT ( 'NONE',  ( 73.76522107166850617, 0.6013300790671820550, 14.08091825663031926 ) ) ;
#25056=DIRECTION ( 'NONE',  ( 0.000000000000000000, 0.000000000000000000, 1.000000000000000000 ) ) ;
#25063=CARTESIAN_POINT ( 'NONE',  ( -37.03867781279360827, -5.627071229729164514, 14.99370382524486089 ) ) ;
#25067=DIRECTION ( 'NONE',  ( -0.000000000000000000, 1.000000000000000000, -0.000000000000000000 ) ) ;
#25081=CIRCLE ( 'NONE', #11957, 55.00000000000000000 ) ;
#25085=EDGE_LOOP ( 'NONE', ( #29709, #26262 ) ) ;
#25091=EDGE_CURVE ( 'NONE', #3409, #2830, #3927, .T. ) ;
#25099=DIRECTION ( 'NONE',  ( 0.000000000000000000, -1.000000000000000000, 0.000000000000000000 ) ) ;
#25110=CARTESIAN_POINT ( 'NONE',  ( 52.83083363940430388, -5.773219817368569373, -11.52912231966167056 ) ) ;
#25122=FACE_OUTER_BOUND ( 'NONE', #7906, .T. ) ;
#25128=EDGE_CURVE ( 'NONE', #10313, #23399, #31802, .T. ) ;
#25129=AXIS2_PLACEMENT_3D ( 'NONE', #20989, #31017, #24096 ) ;
#25138=FACE_OUTER_BOUND ( 'NONE', #9485, .T. ) ;
#25146=LINE ( 'NONE', #25628, #24635 ) ;
#25154=VECTOR ( 'NONE', #19415, 1000.000000000000000 ) ;
#25155=CARTESIAN_POINT ( 'NONE',  ( 53.69468933856271775, -5.264348929021193335, 103.7321922401826981 ) ) ;
#25157=CARTESIAN_POINT ( 'NONE',  ( 21.09785597605719332, 14.86454579224779948, 47.04930799450051637 ) ) ;
#25160=CARTESIAN_POINT ( 'NONE',  ( 47.79865503179234310, 9.702389020015065313, -3.412202488244239884 ) ) ;
#25163=CARTESIAN_POINT ( 'NONE',  ( 21.09785597605719332, -6.704410789454799513, 47.04930799450051637 ) ) ;
#25170=EDGE_CURVE ( 'NONE', #9845, #21115, #27319, .T. ) ;
#25172=ADVANCED_FACE ( 'NONE', ( #6690 ), #27887, .F. ) ;
#25173=DIRECTION ( 'NONE',  ( -0.000000000000000000, -1.000000000000000000, 9.698999007525574140E-17 ) ) ;
#25174=VECTOR ( 'NONE', #18989, 1000.000000000000000 ) ;
#25179=FACE_OUTER_BOUND ( 'NONE', #4439, .T. ) ;
#25188=CARTESIAN_POINT ( 'NONE',  ( -36.98761417531858342, -5.935454207752198563, 77.87546120947918382 ) ) ;
#25191=CARTESIAN_POINT ( 'NONE',  ( 78.96239148643020656, -5.919445383190008236, 78.27029210513457258 ) ) ;
#25205=ORIENTED_EDGE ( 'NONE', *, *, #12914, .F. ) ;
#25221=CARTESIAN_POINT ( 'NONE',  ( 21.09785597605719332, 11.92558985988973497, 47.04930799450051637 ) ) ;
#25223=CARTESIAN_POINT ( 'NONE',  ( -32.36020198612200716, 0.9737162801293415271, 79.86951263711033278 ) ) ;
#25226=ORIENTED_EDGE ( 'NONE', *, *, #186, .F. ) ;
#25228=CARTESIAN_POINT ( 'NONE',  ( -9.504800311772120480, 5.005525289648605991, 98.30203229136020582 ) ) ;
#25231=CARTESIAN_POINT ( 'NONE',  ( 79.37786958444415575, -5.721341737285090545, 15.14745076809877133 ) ) ;
#25241=CARTESIAN_POINT ( 'NONE',  ( 21.09785597605719332, -15.93545420775219945, -37.45069200549951915 ) ) ;
#25259=CARTESIAN_POINT ( 'NONE',  ( -4.902144023942810236, 24.86454579224779948, 44.54930799450078638 ) ) ;
#25261=FACE_OUTER_BOUND ( 'NONE', #31683, .T. ) ;
#25262=ADVANCED_FACE ( 'NONE', ( #4886 ), #32374, .F. ) ;
#25271=CARTESIAN_POINT ( 'NONE',  ( 54.44545748192361145, -4.258649047046827896, 103.5750977336757188 ) ) ;
#25274=CARTESIAN_POINT ( 'NONE',  ( 52.94504501510867556, -5.721341737285968065, -11.26059709029990330 ) ) ;
#25284=FACE_OUTER_BOUND ( 'NONE', #6704, .T. ) ;
#25298=LINE ( 'NONE', #18210, #29730 ) ;
#25301=CARTESIAN_POINT ( 'NONE',  ( -29.27613032885505007, -4.281517947942904634, 80.46297774100551692 ) ) ;
#25302=CARTESIAN_POINT ( 'NONE',  ( 81.58034905098003264, -5.935653941159266367, 16.06701660332827331 ) ) ;
#25310=CARTESIAN_POINT ( 'NONE',  ( 21.09785597605719332, 24.56454579224780232, 47.04930799450051637 ) ) ;
#25317=DIRECTION ( 'NONE',  ( -3.761114140369701376E-15, -1.000000000000000000, -0.000000000000000000 ) ) ;
#25324=CARTESIAN_POINT ( 'NONE',  ( -39.46567364092025798, -5.935459928907636851, 77.98438527425163613 ) ) ;
#25332=CARTESIAN_POINT ( 'NONE',  ( -39.45090951743608088, -5.935454519444268051, 77.98460375324034999 ) ) ;
#25339=CIRCLE ( 'NONE', #30596, 0.2999999999999947153 ) ;
#25341=CARTESIAN_POINT ( 'NONE',  ( 21.09785597605720042, -5.986312001189870280, 114.4134811058426209 ) ) ;
#25343=ORIENTED_EDGE ( 'NONE', *, *, #20966, .F. ) ;
#25344=DIRECTION ( 'NONE',  ( -0.000000000000000000, 1.000000000000000000, -0.000000000000000000 ) ) ;
#25353=CARTESIAN_POINT ( 'NONE',  ( 81.54614529590624272, -5.936959954202220224, 77.95369730613863624 ) ) ;
#25361=CARTESIAN_POINT ( 'NONE',  ( 21.09785597605719332, -19.93545420775220123, 47.04930799450051637 ) ) ;
#25364=CARTESIAN_POINT ( 'NONE',  ( -10.80400125034478087, -5.721341737285083440, -11.23070561388631816 ) ) ;
#25378=CARTESIAN_POINT ( 'NONE',  ( 47.79865503179234310, 9.702389020015065313, -4.315940132965163656 ) ) ;
#25380=CARTESIAN_POINT ( 'NONE',  ( -36.31527284916851528, -5.096557943222667753, 79.79328601240887053 ) ) ;
#25381=CARTESIAN_POINT ( 'NONE',  ( 52.07598125402753197, -5.935454207809698346, -13.48459002699794063 ) ) ;
#25387=EDGE_LOOP ( 'NONE', ( #6168, #16720, #8156, #23049 ) ) ;
#25396=CARTESIAN_POINT ( 'NONE',  ( 21.09785597605719332, 16.33322284159648063, 47.04930799450051637 ) ) ;
#25405=AXIS2_PLACEMENT_3D ( 'NONE', #23325, #28252, #836 ) ;
#25408=CIRCLE ( 'NONE', #21711, 2.000000000000000000 ) ;
#25428=ORIENTED_EDGE ( 'NONE', *, *, #13716, .T. ) ;
#25431=CARTESIAN_POINT ( 'NONE',  ( 100.3079064823960493, -15.93545420775219945, 49.54930799450134771 ) ) ;
#25439=CARTESIAN_POINT ( 'NONE',  ( -9.806533335581546496, -5.936959954202215783, 107.4975973143492212 ) ) ;
#25452=ORIENTED_EDGE ( 'NONE', *, *, #17465, .F. ) ;
#25462=CARTESIAN_POINT ( 'NONE',  ( 21.09785597605719332, 25.56454579224780232, -34.66074251183835031 ) ) ;
#25464=DIRECTION ( 'NONE',  ( -0.000000000000000000, -1.000000000000000000, -0.000000000000000000 ) ) ;
#25465=DIRECTION ( 'NONE',  ( -1.000000000000000000, -0.000000000000000000, -3.491481338843133355E-15 ) ) ;
#25484=ORIENTED_EDGE ( 'NONE', *, *, #11653, .T. ) ;
#25490=CARTESIAN_POINT ( 'NONE',  ( -34.31970563170440158, 11.92558985988973497, 54.04930799450052348 ) ) ;
#25492=EDGE_CURVE ( 'NONE', #23355, #13639, #18632, .T. ) ;
#25498=EDGE_CURVE ( 'NONE', #18486, #7700, #5357, .T. ) ;
#25499=ORIENTED_EDGE ( 'NONE', *, *, #3666, .T. ) ;
#25511=CARTESIAN_POINT ( 'NONE',  ( 75.60381228737249160, -2.946992577399056845, 80.78646212873525201 ) ) ;
#25515=CARTESIAN_POINT ( 'NONE',  ( 77.26108931935814894, -3.866180060838781074, 80.58188637928151365 ) ) ;
#25516=ORIENTED_EDGE ( 'NONE', *, *, #21431, .F. ) ;
#25518=CARTESIAN_POINT ( 'NONE',  ( 21.09785597605719332, -9.935454207752199451, 47.04930799450051637 ) ) ;
#25519=ORIENTED_EDGE ( 'NONE', *, *, #17465, .T. ) ;
#25520=DIRECTION ( 'NONE',  ( 0.000000000000000000, 0.000000000000000000, -1.000000000000000000 ) ) ;
#25534=CARTESIAN_POINT ( 'NONE',  ( -9.801550764381037339, -5.936960083300406588, 107.7467107960321329 ) ) ;
#25541=VECTOR ( 'NONE', #16611, 1000.000000000000000 ) ;
#25550=CARTESIAN_POINT ( 'NONE',  ( 81.68751454973200055, -5.936602078651308290, 15.96907019450728349 ) ) ;
#25552=DIRECTION ( 'NONE',  ( 0.000000000000000000, 1.000000000000000000, 0.000000000000000000 ) ) ;
#25564=B_SPLINE_CURVE_WITH_KNOTS ( 'NONE', 3,
 ( #27680, #10128, #12920, #17824, #22415, #7665, #15208, #7334, #2892, #22910, #17659, #5041, #24897, #4707, #5197, #29660, #17505, #9960 ),
 .UNSPECIFIED., .F., .F.,
 ( 4, 2, 2, 2, 2, 2, 2, 2, 4 ),
 ( 0.0002279586355434578149, 0.0006426580022518073006, 0.001057357368960156786, 0.001472056735668506164, 0.001886756102376855758, 0.002301455469085205569, 0.002716154835793554295, 0.003130854202501903889, 0.003545553569210253483 ),
 .UNSPECIFIED. ) ;
#25568=AXIS2_PLACEMENT_3D ( 'NONE', #16482, #14362, #31596 ) ;
#25573=CARTESIAN_POINT ( 'NONE',  ( 80.77181806311267565, -5.983766253076982622, 14.98546771274985012 ) ) ;
#25574=ORIENTED_EDGE ( 'NONE', *, *, #23611, .F. ) ;
#25577=CARTESIAN_POINT ( 'NONE',  ( 52.78302439342900954, -5.819500620027733717, 105.8370519042862981 ) ) ;
#25589=VECTOR ( 'NONE', #19813, 1000.000000000000000 ) ;
#25612=ORIENTED_EDGE ( 'NONE', *, *, #12657, .T. ) ;
#25613=ADVANCED_FACE ( 'NONE', ( #24871 ), #21901, .F. ) ;
#25616=CARTESIAN_POINT ( 'NONE',  ( 21.09785597605719332, 13.74476430820393347, 47.04930799450051637 ) ) ;
#25617=VECTOR ( 'NONE', #5095, 1000.000000000000000 ) ;
#25621=CARTESIAN_POINT ( 'NONE',  ( 21.09785597605720397, -9.935454207752199451, -24.25069200549945947 ) ) ;
#25624=DIRECTION ( 'NONE',  ( 0.000000000000000000, 0.000000000000000000, -1.000000000000000000 ) ) ;
#25626=DIRECTION ( 'NONE',  ( 0.000000000000000000, 0.000000000000000000, -1.000000000000000000 ) ) ;
#25627=DIRECTION ( 'NONE',  ( 0.000000000000000000, 0.000000000000000000, 1.000000000000000000 ) ) ;
#25628=CARTESIAN_POINT ( 'NONE',  ( 21.09785597605719687, -19.93545420775220123, 27.04930799450051637 ) ) ;
#25630=VERTEX_POINT ( 'NONE', #12405 ) ;
#25642=CARTESIAN_POINT ( 'NONE',  ( 21.09785597605719332, 14.86454579224779948, 47.04930799450051637 ) ) ;
#25648=LINE ( 'NONE', #5474, #12795 ) ;
#25653=AXIS2_PLACEMENT_3D ( 'NONE', #20449, #30478, #18301 ) ;
#25661=LINE ( 'NONE', #8268, #12369 ) ;
#25663=DIRECTION ( 'NONE',  ( -1.000000000000000000, -0.000000000000000000, -0.000000000000000000 ) ) ;
#25672=CARTESIAN_POINT ( 'NONE',  ( -40.78929398160038744, 0.6853371204142075790, 42.04930799450051637 ) ) ;
#25674=ORIENTED_EDGE ( 'NONE', *, *, #370, .T. ) ;
#25686=CARTESIAN_POINT ( 'NONE',  ( 21.09785597605720042, 15.56454579224779877, 101.5493079945004951 ) ) ;
#25693=ORIENTED_EDGE ( 'NONE', *, *, #18960, .T. ) ;
#25695=AXIS2_PLACEMENT_3D ( 'NONE', #4722, #7020, #9649 ) ;
#25699=DIRECTION ( 'NONE',  ( -0.000000000000000000, -1.000000000000000000, 0.000000000000000000 ) ) ;
#25700=CARTESIAN_POINT ( 'NONE',  ( 81.72575882806418690, -5.937449718911897101, 16.02633765848928249 ) ) ;
#25703=CARTESIAN_POINT ( 'NONE',  ( -34.36402903725590363, 11.90988715843502632, 40.33535946719864995 ) ) ;
#25713=DIRECTION ( 'NONE',  ( 1.313185983435984691E-29, -1.000000000000000000, -3.761114140369702165E-15 ) ) ;
#25726=AXIS2_PLACEMENT_3D ( 'NONE', #13619, #18683, #8365 ) ;
#25734=CARTESIAN_POINT ( 'NONE',  ( -7.126919271800058908, 8.279996179725062078, 98.49479233384352028 ) ) ;
#25752=CARTESIAN_POINT ( 'NONE',  ( 54.51561412322114109, -4.114116020023750764, 103.4405055751862079 ) ) ;
#25756=ORIENTED_EDGE ( 'NONE', *, *, #3666, .F. ) ;
#25768=ORIENTED_EDGE ( 'NONE', *, *, #30031, .F. ) ;
#25776=CARTESIAN_POINT ( 'NONE',  ( 21.09785597605719332, 25.56454579224779877, 86.74871914086746472 ) ) ;
#25781=DIRECTION ( 'NONE',  ( 0.000000000000000000, -0.000000000000000000, -1.000000000000000000 ) ) ;
#25792=FACE_OUTER_BOUND ( 'NONE', #25994, .T. ) ;
#25807=CARTESIAN_POINT ( 'NONE',  ( -39.40232922475848909, -5.936135130407838467, 77.93127265747673960 ) ) ;
#25809=EDGE_LOOP ( 'NONE', ( #2934, #15424, #23545, #21876 ) ) ;
#25814=DIRECTION ( 'NONE',  ( -0.000000000000000000, 1.000000000000000000, -0.000000000000000000 ) ) ;
#25821=ORIENTED_EDGE ( 'NONE', *, *, #18043, .F. ) ;
#25822=CARTESIAN_POINT ( 'NONE',  ( 21.09785597605719332, -9.935454207752199451, 47.04930799450051637 ) ) ;
#25830=DIRECTION ( 'NONE',  ( -0.000000000000000000, 1.000000000000000000, -0.000000000000000000 ) ) ;
#25837=CARTESIAN_POINT ( 'NONE',  ( -9.880269303432738681, -5.935454207752202116, -12.56967651669337727 ) ) ;
#25841=CARTESIAN_POINT ( 'NONE',  ( 54.50543043370684870, -4.161241697801258077, -9.378833830732101973 ) ) ;
#25855=EDGE_CURVE ( 'NONE', #23266, #21162, #18795, .T. ) ;
#25857=ORIENTED_EDGE ( 'NONE', *, *, #10166, .T. ) ;
#25868=ORIENTED_EDGE ( 'NONE', *, *, #5668, .F. ) ;
#25871=ORIENTED_EDGE ( 'NONE', *, *, #5668, .T. ) ;
#25884=ORIENTED_EDGE ( 'NONE', *, *, #4340, .F. ) ;
#25885=EDGE_CURVE ( 'NONE', #31909, #32279, #10925, .T. ) ;
#25890=CARTESIAN_POINT ( 'NONE',  ( -11.78368228729793543, -4.961365878511771577, 104.2979330918141585 ) ) ;
#25891=UNCERTAINTY_MEASURE_WITH_UNIT (LENGTH_MEASURE( 1.000000000000000082E-05 ), #18266, 'distance_accuracy_value', 'NONE');
#25896=CARTESIAN_POINT ( 'NONE',  ( 21.09785597605719332, -16.72540370141334520, 47.04930799450051637 ) ) ;
#25899=EDGE_CURVE ( 'NONE', #9845, #31626, #25081, .T. ) ;
#25907=CARTESIAN_POINT ( 'NONE',  ( 44.25300042956540381, 11.55930814891847902, 98.98522354484056507 ) ) ;
#25908=CARTESIAN_POINT ( 'NONE',  ( 50.84143616388391251, 6.334306897662570712, 98.87890954738082883 ) ) ;
#25920=LINE ( 'NONE', #3275, #29343 ) ;
#25929=CARTESIAN_POINT ( 'NONE',  ( -44.94873447355087137, -5.453371160069278467, 52.74359862448790892 ) ) ;
#25931=VECTOR ( 'NONE', #20622, 1000.000000000000000 ) ;
#25933=AXIS2_PLACEMENT_3D ( 'NONE', #31992, #26741, #29367 ) ;
#25945=VERTEX_POINT ( 'NONE', #31249 ) ;
#25954=PRODUCT_DEFINITION ( 'UNKNOWN', '', #18150, #9789 ) ;
#25961=CARTESIAN_POINT ( 'NONE',  ( -39.41385926433662235, -5.936084327709292729, 77.91473385016919906 ) ) ;
#25963=B_SPLINE_CURVE_WITH_KNOTS ( 'NONE', 3,
 ( #9799, #2566, #14888, #2733, #30155, #7504, #27356, #7825, #4874, #25378 ),
 .UNSPECIFIED., .F., .F.,
 ( 4, 2, 2, 2, 4 ),
 ( 0.0006716755660530369584, 0.002413276598758841776, 0.004154877631464646594, 0.005896478664170451411, 0.007638079696876256229 ),
 .UNSPECIFIED. ) ;
#25966=CARTESIAN_POINT ( 'NONE',  ( 21.09785597605719332, 15.63322284159649556, 47.04930799450051637 ) ) ;
#25976=CARTESIAN_POINT ( 'NONE',  ( 21.09785597605719332, 25.56454579224779877, 47.04930799450051637 ) ) ;
#25989=CARTESIAN_POINT ( 'NONE',  ( 79.15081694298606863, -5.581242224120285478, 79.20493092526746182 ) ) ;
#25994=EDGE_LOOP ( 'NONE', ( #27818, #9902, #8158, #11128 ) ) ;
#26000=DIRECTION ( 'NONE',  ( 0.000000000000000000, -0.7071067811865378028, -0.7071067811865573427 ) ) ;
#26016=CARTESIAN_POINT ( 'NONE',  ( 21.09785597605719332, 14.56957104541719694, 47.04930799450051637 ) ) ;
#26036=EDGE_CURVE ( 'NONE', #23355, #28042, #9350, .T. ) ;
#26038=FACE_OUTER_BOUND ( 'NONE', #9741, .T. ) ;
#26039=ORIENTED_EDGE ( 'NONE', *, *, #9337, .T. ) ;
#26049=EDGE_CURVE ( 'NONE', #8721, #23768, #13547, .T. ) ;
#26053=CARTESIAN_POINT ( 'NONE',  ( 52.20364351894168919, -5.936611295272324895, 106.6063773940375228 ) ) ;
#26060=CARTESIAN_POINT ( 'NONE',  ( 47.09785597605719687, 25.56454579224779877, 44.54930799450042400 ) ) ;
#26067=DIRECTION ( 'NONE',  ( 0.000000000000000000, 0.000000000000000000, -1.000000000000000000 ) ) ;
#26068=CARTESIAN_POINT ( 'NONE',  ( -34.91457700022733945, -4.675691201108098660, 13.95142249688010949 ) ) ;
#26075=CARTESIAN_POINT ( 'NONE',  ( 47.09785597605719687, 24.86454579224779948, 47.04930799450042400 ) ) ;
#26083=EDGE_CURVE ( 'NONE', #16169, #21481, #516, .T. ) ;
#26100=DIRECTION ( 'NONE',  ( -0.000000000000000000, -1.000000000000000000, -0.000000000000000000 ) ) ;
#26123=CARTESIAN_POINT ( 'NONE',  ( 21.09785597605719332, -9.935454207752199451, 47.04930799450051637 ) ) ;
#26127=B_SPLINE_CURVE_WITH_KNOTS ( 'NONE', 3,
 ( #25490, #13025, #10725, #3149, #13194, #23186, #20721, #30747, #8254, #18241, #6431, #16588 ),
 .UNSPECIFIED., .F., .F.,
 ( 4, 2, 2, 2, 2, 4 ),
 ( 0.0002000209647945283933, 0.001054195637184463354, 0.001481282973379431742, 0.001908370309574400348, 0.002762544981964341027, 0.003616719654354280840 ),
 .UNSPECIFIED. ) ;
#26150=CIRCLE ( 'NONE', #24061, 67.32891250266496286 ) ;
#26161=CARTESIAN_POINT ( 'NONE',  ( 53.14761115485138276, 2.529769287487982687, -5.868558487217412356 ) ) ;
#26168=VECTOR ( 'NONE', #1370, 1000.000000000000000 ) ;
#26169=VERTEX_POINT ( 'NONE', #28111 ) ;
#26170=AXIS2_PLACEMENT_3D ( 'NONE', #16791, #4491, #28786 ) ;
#26173=CARTESIAN_POINT ( 'NONE',  ( 81.79463805813215060, -5.936463533621012090, 77.90792605297762918 ) ) ;
#26191=FACE_OUTER_BOUND ( 'NONE', #14952, .T. ) ;
#26203=ORIENTED_EDGE ( 'NONE', *, *, #20222, .T. ) ;
#26207=ADVANCED_FACE ( 'NONE', ( #25792 ), #31052, .F. ) ;
#26208=AXIS2_PLACEMENT_3D ( 'NONE', #6172, #23569, #21410 ) ;
#26211=CIRCLE ( 'NONE', #7370, 55.85791022362053582 ) ;
#26233=CARTESIAN_POINT ( 'NONE',  ( -5.602943079677954685, 9.702389020015065313, 132.0493079945005377 ) ) ;
#26246=ORIENTED_EDGE ( 'NONE', *, *, #30471, .F. ) ;
#26256=VERTEX_POINT ( 'NONE', #20865 ) ;
#26262=ORIENTED_EDGE ( 'NONE', *, *, #32139, .F. ) ;
#26265=CARTESIAN_POINT ( 'NONE',  ( 74.00358335591296566, 2.565965067347307116, 15.01823474329995811 ) ) ;
#26267=ORIENTED_EDGE ( 'NONE', *, *, #11893, .T. ) ;
#26270=VERTEX_POINT ( 'NONE', #1007 ) ;
#26289=EDGE_CURVE ( 'NONE', #2830, #6661, #16419, .T. ) ;
#26296=DIRECTION ( 'NONE',  ( 1.000000000000000000, 0.000000000000000000, -1.224646799147353207E-16 ) ) ;
#26301=CARTESIAN_POINT ( 'NONE',  ( 21.09785597605720397, -16.43042895458278352, 119.0543332476699021 ) ) ;
#26306=DIRECTION ( 'NONE',  ( 0.000000000000000000, 0.000000000000000000, -1.000000000000000000 ) ) ;
#26325=LINE ( 'NONE', #6301, #26168 ) ;
#26335=CARTESIAN_POINT ( 'NONE',  ( -30.88361636257000598, 11.92558985988973141, 67.49515520264003499 ) ) ;
#26336=CARTESIAN_POINT ( 'NONE',  ( -58.11219453028166981, -16.63545420775219696, 47.04930799450023926 ) ) ;
#26370=AXIS2_PLACEMENT_3D ( 'NONE', #10468, #28184, #1562 ) ;
#26384=CYLINDRICAL_SURFACE ( 'NONE', #30171, 2.500000000000002220 ) ;
#26385=CARTESIAN_POINT ( 'NONE',  ( 21.09785597605719332, -15.93545420775219945, 128.7593585008393973 ) ) ;
#26391=CARTESIAN_POINT ( 'NONE',  ( -10.61756623293725177, -5.811083640285386487, -10.47712082112068188 ) ) ;
#26400=ORIENTED_EDGE ( 'NONE', *, *, #30522, .F. ) ;
#26401=CARTESIAN_POINT ( 'NONE',  ( 41.51205063648687599, 11.92558985988973497, -5.803495753465989893 ) ) ;
#26405=ORIENTED_EDGE ( 'NONE', *, *, #15620, .F. ) ;
#26408=DIRECTION ( 'NONE',  ( 7.539678551159015339E-17, -0.7880107536067239016, 0.6156614753256557382 ) ) ;
#26412=VERTEX_POINT ( 'NONE', #19034 ) ;
#26447=CIRCLE ( 'NONE', #18055, 56.65825807113184709 ) ;
#26452=CIRCLE ( 'NONE', #30668, 55.00000000000000000 ) ;
#26456=DIRECTION ( 'NONE',  ( 0.000000000000000000, 0.000000000000000000, 1.000000000000000000 ) ) ;
#26480=CARTESIAN_POINT ( 'NONE',  ( -39.53252429583445604, -5.935481122642606522, 77.87649032733463628 ) ) ;
#26487=B_SPLINE_CURVE_WITH_KNOTS ( 'NONE', 3,
 ( #31732, #16939, #22193, #29592, #9242, #26802, #31887, #9404, #19405, #26957, #4480, #7104, #14499, #27123, #24492, #17102, #14660, #24666, #2183, #32224, #13613, #8524, #7928, #12529, #2825, #17600, #12854, #22846, #20986, #17924, #31014, #359, #27612, #3588, #6064, #26068, #24993, #27942, #15308, #10067, #23618, #10382, #18516, #7756 ),
 .UNSPECIFIED., .F., .F.,
 ( 4, 2, 2, 2, 2, 2, 2, 2, 2, 2, 2, 2, 2, 2, 2, 2, 2, 2, 2, 2, 2, 4 ),
 ( 0.000000000000000000, 0.001748345063742785897, 0.003496690127485571793, 0.005245035191228358123, 0.006119207723099748253, 0.006993380254971139250, 0.008741725318713916906, 0.01049007038245669370, 0.01223841544619947048, 0.01398676050994224727, 0.01573510557368502233, 0.01748345063742779912, 0.01923179570117057244, 0.02010596823304195563, 0.02098014076491334229, 0.02272848582865609826, 0.02360265836052748145, 0.02447683089239886464, 0.02535100342427025130, 0.02622517595614163102, 0.02709934848801301768, 0.02797352101988440087 ),
 .UNSPECIFIED. ) ;
#26491=VERTEX_POINT ( 'NONE', #30536 ) ;
#26492=CARTESIAN_POINT ( 'NONE',  ( 72.46310410352296572, 9.702389020015065313, 20.34850893876554778 ) ) ;
#26499=CIRCLE ( 'NONE', #24339, 84.30000000000001137 ) ;
#26502=CARTESIAN_POINT ( 'NONE',  ( 81.78746918506877250, -5.936918610400974572, 77.96063504348295226 ) ) ;
#26508=CARTESIAN_POINT ( 'NONE',  ( 0.1399989214664148496, 11.92558985988973852, 98.82976274952495999 ) ) ;
#26515=ORIENTED_EDGE ( 'NONE', *, *, #28610, .F. ) ;
#26517=DIRECTION ( 'NONE',  ( 0.000000000000000000, 1.000000000000000000, 0.000000000000000000 ) ) ;
#26519=DIRECTION ( 'NONE',  ( 0.000000000000000000, 0.000000000000000000, -1.000000000000000000 ) ) ;
#26521=ORIENTED_EDGE ( 'NONE', *, *, #29076, .F. ) ;
#26526=DIRECTION ( 'NONE',  ( 0.000000000000000000, -0.7071067811865474617, -0.7071067811865474617 ) ) ;
#26539=ORIENTED_EDGE ( 'NONE', *, *, #25170, .F. ) ;
#26541=DIRECTION ( 'NONE',  ( 1.000000000000000000, 0.000000000000000000, -1.110223024625154963E-14 ) ) ;
#26547=CARTESIAN_POINT ( 'NONE',  ( -10.26669494407825134, -5.913508961333113767, -10.73378008532072414 ) ) ;
#26566=EDGE_LOOP ( 'NONE', ( #15028, #6969, #17992, #19990, #26864, #24570, #29322, #8514, #3647, #30317, #9471, #26845, #4565, #18203, #20278, #31005, #30514, #18387, #18500, #16999, #19827, #10491 ) ) ;
#26570=ORIENTED_EDGE ( 'NONE', *, *, #8030, .F. ) ;
#26585=ORIENTED_EDGE ( 'NONE', *, *, #17656, .F. ) ;
#26586=DIRECTION ( 'NONE',  ( 0.000000000000000000, -1.000000000000000000, 0.000000000000000000 ) ) ;
#26589=AXIS2_PLACEMENT_3D ( 'NONE', #3177, #8278, #22555 ) ;
#26591=ORIENTED_EDGE ( 'NONE', *, *, #29233, .T. ) ;
#26592=ORIENTED_EDGE ( 'NONE', *, *, #7125, .F. ) ;
#26620=CARTESIAN_POINT ( 'NONE',  ( 54.71524953585419127, -1.428409478025996160, -6.539106349574636212 ) ) ;
#26622=CARTESIAN_POINT ( 'NONE',  ( 21.09785597605719332, -15.93545420775219945, 47.04930799450051637 ) ) ;
#26638=CARTESIAN_POINT ( 'NONE',  ( 21.09785597605719332, 13.74476430820393347, 103.0493079945005093 ) ) ;
#26656=CARTESIAN_POINT ( 'NONE',  ( -31.14390254341316577, 1.751253714874866141, 79.49571236864932189 ) ) ;
#26659=ORIENTED_EDGE ( 'NONE', *, *, #3709, .T. ) ;
#26661=CARTESIAN_POINT ( 'NONE',  ( 52.07878664889356912, -5.935345006353229813, -13.65255231306078798 ) ) ;
#26665=CARTESIAN_POINT ( 'NONE',  ( 21.09785597605719332, 11.92558985988973497, 47.04930799450051637 ) ) ;
#26674=CARTESIAN_POINT ( 'NONE',  ( 21.09785597605719332, 11.78014697381582643, 47.04930799450051637 ) ) ;
#26676=CARTESIAN_POINT ( 'NONE',  ( 21.09785597605719332, -5.935454207752083988, 47.04930799450039558 ) ) ;
#26699=DIRECTION ( 'NONE',  ( 1.000000000000000000, 0.000000000000000000, 1.224646799147353207E-16 ) ) ;
#26700=FACE_OUTER_BOUND ( 'NONE', #7147, .T. ) ;
#26709=CARTESIAN_POINT ( 'NONE',  ( -44.16105795751995799, -3.935454207752190126, 42.04930799450051637 ) ) ;
#26721=EDGE_LOOP ( 'NONE', ( #1176, #17162, #4415, #18174 ) ) ;
#26733=CIRCLE ( 'NONE', #30938, 1.000000000000000888 ) ;
#26741=DIRECTION ( 'NONE',  ( 0.000000000000000000, -1.000000000000000000, 0.000000000000000000 ) ) ;
#26756=EDGE_CURVE ( 'NONE', #32254, #14591, #23006, .T. ) ;
#26762=AXIS2_PLACEMENT_3D ( 'NONE', #26674, #28981, #3871 ) ;
#26763=CARTESIAN_POINT ( 'NONE',  ( 21.09785597605720397, -9.935454207752199451, -24.95069200549946586 ) ) ;
#26765=CARTESIAN_POINT ( 'NONE',  ( -12.44131731965827292, -3.812314126620122146, -9.074964031059534975 ) ) ;
#26802=CARTESIAN_POINT ( 'NONE',  ( -29.67914774177176795, 11.17072198059736365, 22.77948424423242813 ) ) ;
#26805=CARTESIAN_POINT ( 'NONE',  ( -39.54153637835258905, -5.935542461338363829, 77.87913874700778649 ) ) ;
#26819=VECTOR ( 'NONE', #14494, 1000.000000000000000 ) ;
#26825=CARTESIAN_POINT ( 'NONE',  ( -29.94453746500173352, 11.54296414969715734, 70.26170135685566720 ) ) ;
#26829=ORIENTED_EDGE ( 'NONE', *, *, #25492, .F. ) ;
#26834=CARTESIAN_POINT ( 'NONE',  ( -3.642799471247537113, 10.95964320463251163, 97.72816333341694417 ) ) ;
#26836=CARTESIAN_POINT ( 'NONE',  ( 72.68065935034339020, 11.88159288520708401, 68.55220373536670309 ) ) ;
#26845=ORIENTED_EDGE ( 'NONE', *, *, #30063, .F. ) ;
#26849=CARTESIAN_POINT ( 'NONE',  ( -45.73385703294348303, -5.935454207752201228, 53.94857996627248298 ) ) ;
#26850=DIRECTION ( 'NONE',  ( 0.000000000000000000, 1.000000000000000000, 9.698999007525318993E-17 ) ) ;
#26854=ORIENTED_EDGE ( 'NONE', *, *, #14053, .T. ) ;
#26861=EDGE_CURVE ( 'NONE', #31117, #10313, #11512, .T. ) ;
#26864=ORIENTED_EDGE ( 'NONE', *, *, #29233, .F. ) ;
#26875=CARTESIAN_POINT ( 'NONE',  ( -11.70578502262792320, 0.9814505390143252184, -5.472609761470430101 ) ) ;
#26890=CARTESIAN_POINT ( 'NONE',  ( -38.57628410747783221, 2.267350949466874432, 14.79705809024468088 ) ) ;
#26899=AXIS2_PLACEMENT_3D ( 'NONE', #23449, #11149, #21131 ) ;
#26903=CONICAL_SURFACE ( 'NONE', #14327, 54.50502525316942126, 0.7853981633974552734 ) ;
#26913=CARTESIAN_POINT ( 'NONE',  ( 21.09785597605719332, 11.92558985988973497, 47.04930799450051637 ) ) ;
#26917=CARTESIAN_POINT ( 'NONE',  ( 21.09785597605719332, 24.86454579224779948, 47.04930799450051637 ) ) ;
#26927=CARTESIAN_POINT ( 'NONE',  ( 21.09785597605720397, -19.93545420775220123, -37.95069200549950494 ) ) ;
#26929=CARTESIAN_POINT ( 'NONE',  ( -12.49256779602912459, -3.654479441960576835, -8.942264808892717909 ) ) ;
#26941=DIRECTION ( 'NONE',  ( -0.000000000000000000, 1.000000000000000000, -0.000000000000000000 ) ) ;
#26942=DIRECTION ( 'NONE',  ( -0.000000000000000000, 1.000000000000000000, -0.000000000000000000 ) ) ;
#26947=CARTESIAN_POINT ( 'NONE',  ( 50.76169387283900392, 6.453333540778361410, -3.825706102817799881 ) ) ;
#26957=CARTESIAN_POINT ( 'NONE',  ( -29.38155059246552625, 10.03279525182523813, 20.77577928944664265 ) ) ;
#26970=AXIS2_PLACEMENT_3D ( 'NONE', #17912, #26100, #13163 ) ;
#26973=CARTESIAN_POINT ( 'NONE',  ( 52.07598125554711999, -5.935454207752202116, 97.45038561958638468 ) ) ;
#26976=CARTESIAN_POINT ( 'NONE',  ( 71.61633006602951923, 10.39302479005549884, 21.28398100033225404 ) ) ;
#26987=CARTESIAN_POINT ( 'NONE',  ( -32.86366169284681860, -2.090386383962613781, 80.76226970107140346 ) ) ;
#26993=DIRECTION ( 'NONE',  ( -0.000000000000000000, 1.000000000000000000, -0.000000000000000000 ) ) ;
#26994=ORIENTED_EDGE ( 'NONE', *, *, #13761, .F. ) ;
#26997=CARTESIAN_POINT ( 'NONE',  ( 21.09785597605719332, 11.78014697381582643, 47.04930799450051637 ) ) ;
#27012=VERTEX_POINT ( 'NONE', #10603 ) ;
#27021=ADVANCED_FACE ( 'NONE', ( #28311 ), #12745, .F. ) ;
#27022=EDGE_CURVE ( 'NONE', #31909, #8721, #6639, .T. ) ;
#27036=CARTESIAN_POINT ( 'NONE',  ( -10.78113380436533220, -5.738638231773887100, -10.34064955166817867 ) ) ;
#27037=VERTEX_POINT ( 'NONE', #7974 ) ;
#27045=EDGE_LOOP ( 'NONE', ( #22150, #11680, #29994, #147 ) ) ;
#27054=ORIENTED_EDGE ( 'NONE', *, *, #2306, .T. ) ;
#27055=ORIENTED_EDGE ( 'NONE', *, *, #5995, .F. ) ;
#27056=EDGE_LOOP ( 'NONE', ( #28536, #27683, #30673, #16958, #29689, #24554, #19492, #11321, #7195, #29148, #27787, #14697, #21954, #18200, #23930, #29882 ) ) ;
#27061=CARTESIAN_POINT ( 'NONE',  ( 53.16981722132879185, -5.983766253076979069, -3.337848843846767721 ) ) ;
#27067=DIRECTION ( 'NONE',  ( 0.000000000000000000, 1.000000000000000000, 3.754529891495955404E-16 ) ) ;
#27074=FACE_OUTER_BOUND ( 'NONE', #30545, .T. ) ;
#27088=CARTESIAN_POINT ( 'NONE',  ( -12.24974552980923015, -4.258649047046816349, -9.476481744674682517 ) ) ;
#27098=EDGE_LOOP ( 'NONE', ( #19910, #19427, #3778, #17276 ) ) ;
#27100=AXIS2_PLACEMENT_3D ( 'NONE', #32146, #27377, #22114 ) ;
#27103=VERTEX_POINT ( 'NONE', #28627 ) ;
#27107=APPLICATION_CONTEXT ( 'automotive_design' ) ;
#27108=CARTESIAN_POINT ( 'NONE',  ( 47.79865503179234310, 9.702389020015065313, -3.412202488244239884 ) ) ;
#27114=CARTESIAN_POINT ( 'NONE',  ( 106.0978559760575735, 11.92558985988973497, 26.63511333407112858 ) ) ;
#27116=DIRECTION ( 'NONE',  ( 0.000000000000000000, -0.000000000000000000, -1.000000000000000000 ) ) ;
#27118=( LENGTH_UNIT ( ) NAMED_UNIT ( * ) SI_UNIT ( .MILLI., .METRE. ) );
#27123=CARTESIAN_POINT ( 'NONE',  ( -29.46345852492245854, 8.057491331218018971, 18.62581556740637367 ) ) ;
#27124=CARTESIAN_POINT ( 'NONE',  ( 71.48501281440437083, -5.935454207752202116, 77.87546120947915540 ) ) ;
#27144=CARTESIAN_POINT ( 'NONE',  ( -29.37118047130158871, 8.867344695471309990, 74.71416144101659995 ) ) ;
#27146=CIRCLE ( 'NONE', #30841, 2.000000000000001776 ) ;
#27162=DIRECTION ( 'NONE',  ( 0.000000000000000000, -1.000000000000000000, 0.000000000000000000 ) ) ;
#27167=CARTESIAN_POINT ( 'NONE',  ( -45.63946073596905251, -5.900342692619398477, 53.66495926439285569 ) ) ;
#27171=AXIS2_PLACEMENT_3D ( 'NONE', #28805, #16319, #6480 ) ;
#27172=CIRCLE ( 'NONE', #10959, 2.500000000000002220 ) ;
#27173=ORIENTED_EDGE ( 'NONE', *, *, #23611, .T. ) ;
#27174=VECTOR ( 'NONE', #31210, 1000.000000000000000 ) ;
#27180=CARTESIAN_POINT ( 'NONE',  ( 79.00022925220035575, -5.944439029104267469, 15.86926712089771918 ) ) ;
#27181=DIRECTION ( 'NONE',  ( 0.000000000000000000, 0.000000000000000000, -1.000000000000000000 ) ) ;
#27194=CARTESIAN_POINT ( 'NONE',  ( 52.20506317732528601, -5.935651417315359168, 107.5660775608625954 ) ) ;
#27207=CARTESIAN_POINT ( 'NONE',  ( 21.09785597605720042, 15.06454579224778456, 102.0493079945005093 ) ) ;
#27210=CARTESIAN_POINT ( 'NONE',  ( -38.57628410747783221, 5.786705267067572933, 16.84970013494222840 ) ) ;
#27211=EDGE_LOOP ( 'NONE', ( #30038, #8559, #28266, #19510 ) ) ;
#27212=ORIENTED_EDGE ( 'NONE', *, *, #29820, .F. ) ;
#27235=DIRECTION ( 'NONE',  ( 0.000000000000000000, -1.000000000000000000, 0.000000000000000000 ) ) ;
#27245=ORIENTED_EDGE ( 'NONE', *, *, #1991, .F. ) ;
#27251=AXIS2_PLACEMENT_3D ( 'NONE', #21619, #24248, #13769 ) ;
#27253=DIRECTION ( 'NONE',  ( 0.000000000000000000, 9.698999007525574140E-17, 1.000000000000000000 ) ) ;
#27255=EDGE_CURVE ( 'NONE', #8194, #23976, #12209, .T. ) ;
#27261=CARTESIAN_POINT ( 'NONE',  ( -38.14261667679545553, -5.888571448818344933, 15.70117500735613447 ) ) ;
#27281=CIRCLE ( 'NONE', #19398, 4.000000000000003553 ) ;
#27285=ORIENTED_EDGE ( 'NONE', *, *, #14947, .F. ) ;
#27303=CARTESIAN_POINT ( 'NONE',  ( 71.77352134618342916, 10.95165879486606464, 22.29205552524197742 ) ) ;
#27315=EDGE_LOOP ( 'NONE', ( #25001, #6490, #24581, #15367 ) ) ;
#27319=CIRCLE ( 'NONE', #28893, 1.000000000000000888 ) ;
#27331=CARTESIAN_POINT ( 'NONE',  ( 72.84780449950605430, 6.662067023026803092, 76.56641493775845220 ) ) ;
#27340=B_SPLINE_CURVE_WITH_KNOTS ( 'NONE', 3,
 ( #15097, #15738, #20979, #15906, #13452, #316, #476, #25271, #25752, #2783, #8044, #2937, #12808, #13130, #8518, #5733, #10982, #5900, #23447, #22952, #27897, #28219, #28382, #18511, #28541, #644, #18187, #25908, #6058, #10505, #22802, #3424, #23127, #18033, #10336, #960 ),
 .UNSPECIFIED., .F., .F.,
 ( 4, 2, 2, 2, 2, 2, 2, 2, 2, 2, 2, 2, 2, 2, 2, 2, 2, 4 ),
 ( 8.673617379884035472E-19, 0.001253900128824232598, 0.001880850193236362341, 0.002507800257648492518, 0.003134750322060622044, 0.003761700386472752872, 0.005015600515297014526, 0.005642550579709156196, 0.006269500644121296998, 0.007523400772945580336, 0.008777300901769865410, 0.01003120103059414875, 0.01253900128824272583, 0.01504680154589130639, 0.01630070167471558973, 0.01755460180353986960, 0.01880850193236414947, 0.02006240206118843281 ),
 .UNSPECIFIED. ) ;
#27352=CARTESIAN_POINT ( 'NONE',  ( -9.880269301913145341, -5.935454207809699234, 107.5832060159989965 ) ) ;
#27355=CARTESIAN_POINT ( 'NONE',  ( 78.88094405587852975, -5.913508961333113767, 15.68475707436527777 ) ) ;
#27356=CARTESIAN_POINT ( 'NONE',  ( 45.84005119758191427, 10.95889540305195986, -4.518375277153177549 ) ) ;
#27357=CARTESIAN_POINT ( 'NONE',  ( -44.28695544631906955, -5.935454207752198563, 54.04930799450053058 ) ) ;
#27361=CARTESIAN_POINT ( 'NONE',  ( -38.38918381122095980, -5.922340440260644101, 78.18162856751085599 ) ) ;
#27366=ORIENTED_EDGE ( 'NONE', *, *, #5799, .T. ) ;
#27374=DIRECTION ( 'NONE',  ( -0.000000000000000000, 1.000000000000000000, -0.000000000000000000 ) ) ;
#27376=ORIENTED_EDGE ( 'NONE', *, *, #13503, .F. ) ;
#27377=DIRECTION ( 'NONE',  ( 0.000000000000000000, -1.000000000000000000, 0.000000000000000000 ) ) ;
#27387=EDGE_CURVE ( 'NONE', #23768, #11676, #5622, .T. ) ;
#27394=CIRCLE ( 'NONE', #3812, 56.65825807113184709 ) ;
#27402=CARTESIAN_POINT ( 'NONE',  ( -9.899862315945510360, -5.936215030417555383, -13.38459389407276134 ) ) ;
#27410=DIRECTION ( 'NONE',  ( 1.000000000000000000, -3.759183808608825436E-15, 0.000000000000000000 ) ) ;
#27426=EDGE_CURVE ( 'NONE', #22918, #11299, #13124, .T. ) ;
#27428=AXIS2_PLACEMENT_3D ( 'NONE', #11237, #18758, #30622 ) ;
#27431=EDGE_CURVE ( 'NONE', #11299, #22918, #6288, .T. ) ;
#27437=ORIENTED_EDGE ( 'NONE', *, *, #24016, .F. ) ;
#27442=DIRECTION ( 'NONE',  ( -0.000000000000000000, 1.000000000000000000, -0.000000000000000000 ) ) ;
#27448=CARTESIAN_POINT ( 'NONE',  ( 21.09785597605719332, -8.874820941924726370, 47.04930799450051637 ) ) ;
#27449=VECTOR ( 'NONE', #3797, 1000.000000000000000 ) ;
#27452=DIRECTION ( 'NONE',  ( 0.000000000000000000, -1.000000000000000000, 0.000000000000000000 ) ) ;
#27458=EDGE_CURVE ( 'NONE', #21709, #23463, #8909, .T. ) ;
#27459=CARTESIAN_POINT ( 'NONE',  ( -63.90214402394282445, -3.935454207752190126, 42.04930799450051637 ) ) ;
#27463=DIRECTION ( 'NONE',  ( 0.000000000000000000, -1.000000000000000000, 0.000000000000000000 ) ) ;
#27464=CARTESIAN_POINT ( 'NONE',  ( 44.24821932555909854, 11.56063108660457495, -4.010480718324124005 ) ) ;
#27467=CARTESIAN_POINT ( 'NONE',  ( -39.39739818181173803, -5.936352567920400780, 77.94940154167748858 ) ) ;
#27480=CARTESIAN_POINT ( 'NONE',  ( -9.831337038036075171, -5.937394935145314356, 107.4930705127871704 ) ) ;
#27484=DIRECTION ( 'NONE',  ( 1.000000000000000000, -3.759183808608825436E-15, 0.000000000000000000 ) ) ;
#27488=EDGE_CURVE ( 'NONE', #31589, #27037, #23064, .T. ) ;
#27492=ORIENTED_EDGE ( 'NONE', *, *, #25091, .T. ) ;
#27496=DIRECTION ( 'NONE',  ( 0.000000000000000000, 0.000000000000000000, -1.000000000000000000 ) ) ;
#27504=CARTESIAN_POINT ( 'NONE',  ( -45.71589853820119487, -5.927381377935135198, 53.84747426841368423 ) ) ;
#27510=ORIENTED_EDGE ( 'NONE', *, *, #20528, .F. ) ;
#27513=AXIS2_PLACEMENT_3D ( 'NONE', #24566, #4880, #32293 ) ;
#27525=CARTESIAN_POINT ( 'NONE',  ( -9.949026574332460626, 4.272108154687138892, 98.50954949487454826 ) ) ;
#27526=EDGE_LOOP ( 'NONE', ( #4601, #17383, #19249, #26592 ) ) ;
#27527=CARTESIAN_POINT ( 'NONE',  ( -34.35572742831690363, -2.950474395469078637, 13.32293284703904135 ) ) ;
#27541=VERTEX_POINT ( 'NONE', #16103 ) ;
#27543=CARTESIAN_POINT ( 'NONE',  ( -36.45222641229887017, 9.925589859889724309, 52.04930799450051637 ) ) ;
#27546=CIRCLE ( 'NONE', #4478, 65.96844849472888939 ) ;
#27584=ORIENTED_EDGE ( 'NONE', *, *, #5746, .T. ) ;
#27589=DIRECTION ( 'NONE',  ( 0.000000000000000000, 1.000000000000000000, -9.698999007525574140E-17 ) ) ;
#27594=DIRECTION ( 'NONE',  ( 0.000000000000000000, 0.000000000000000000, -1.000000000000000000 ) ) ;
#27602=FACE_BOUND ( 'NONE', #18657, .T. ) ;
#27605=DIRECTION ( 'NONE',  ( -0.000000000000000000, -1.000000000000000000, -0.000000000000000000 ) ) ;
#27612=CARTESIAN_POINT ( 'NONE',  ( -33.97095292404057432, -3.671323332650886506, 13.46144832333910024 ) ) ;
#27615=CARTESIAN_POINT ( 'NONE',  ( 54.55209231583086904, -4.032327822094588399, 102.4332369668683640 ) ) ;
#27630=AXIS2_PLACEMENT_3D ( 'NONE', #10758, #8281, #18594 ) ;
#27634=DIRECTION ( 'NONE',  ( 0.000000000000000000, 0.000000000000000000, -1.000000000000000000 ) ) ;
#27635=CARTESIAN_POINT ( 'NONE',  ( 41.51205063648687599, 11.92558985988973497, 99.04321908912902472 ) ) ;
#27637=EDGE_CURVE ( 'NONE', #13269, #4386, #29926, .T. ) ;
#27642=CARTESIAN_POINT ( 'NONE',  ( 79.40776106085759523, -5.721341737285999152, 78.89649703355206611 ) ) ;
#27645=DIRECTION ( 'NONE',  ( -0.000000000000000000, 1.000000000000000000, -0.000000000000000000 ) ) ;
#27648=CARTESIAN_POINT ( 'NONE',  ( 78.57866796533406273, -5.769399297529532511, 78.79950972727095859 ) ) ;
#27649=CIRCLE ( 'NONE', #7735, 84.21005050633887379 ) ;
#27653=CARTESIAN_POINT ( 'NONE',  ( 75.28003531790183445, -0.7249253372052035793, 80.48926995870992585 ) ) ;
#27660=FACE_OUTER_BOUND ( 'NONE', #8964, .T. ) ;
#27662=DIRECTION ( 'NONE',  ( -0.000000000000000000, -1.000000000000000000, -0.000000000000000000 ) ) ;
#27663=ORIENTED_EDGE ( 'NONE', *, *, #14802, .T. ) ;
#27664=B_SPLINE_SURFACE_WITH_KNOTS ( 'NONE', 3, 1, ( 
 ( #20243, #15167 ),
 ( #9920, #10091 ),
 ( #27969, #27480 ),
 ( #30268, #2526 ) ),
 .UNSPECIFIED., .F., .F., .F.,
 ( 4, 4 ),
 ( 2, 2 ),
 ( 0.1800733115436725096, 0.1889470565094412413 ),
 ( 0.000000000000000000, 1.000000000000000000 ),
 .UNSPECIFIED. ) ;
#27670=ADVANCED_FACE ( 'NONE', ( #4287 ), #16913, .F. ) ;
#27674=EDGE_CURVE ( 'NONE', #16169, #28880, #8356, .T. ) ;
#27680=CARTESIAN_POINT ( 'NONE',  ( -43.35833523721896654, -3.935454207752183020, 52.04930799450050927 ) ) ;
#27681=CARTESIAN_POINT ( 'NONE',  ( 52.99971320245913375, -5.721341737285090545, 105.3293216028873616 ) ) ;
#27683=ORIENTED_EDGE ( 'NONE', *, *, #13270, .T. ) ;
#27686=CARTESIAN_POINT ( 'NONE',  ( -33.89646034886494874, -2.243811656006899025, 13.32259206650234518 ) ) ;
#27715=LINE ( 'NONE', #4912, #21214 ) ;
#27737=EDGE_LOOP ( 'NONE', ( #29578, #8800, #10721, #23105 ) ) ;
#27741=CARTESIAN_POINT ( 'NONE',  ( -9.833199634961228952, -5.936746300155038014, 107.4930292230181408 ) ) ;
#27747=AXIS2_PLACEMENT_3D ( 'NONE', #25221, #20124, #27181 ) ;
#27752=TOROIDAL_SURFACE ( 'NONE', #30380, 67.99999999999997158, 3.299999999999999822 ) ;
#27755=CARTESIAN_POINT ( 'NONE',  ( -44.62459984291964332, -4.794956837033497621, 52.23427270913660436 ) ) ;
#27766=FACE_OUTER_BOUND ( 'NONE', #9302, .T. ) ;
#27775=DIRECTION ( 'NONE',  ( -0.000000000000000000, 1.000000000000000000, -0.000000000000000000 ) ) ;
#27779=AXIS2_PLACEMENT_3D ( 'NONE', #31260, #31419, #19244 ) ;
#27780=CARTESIAN_POINT ( 'NONE',  ( 48.47771913120614329, 9.127627432390728046, 97.50908689856248657 ) ) ;
#27782=CARTESIAN_POINT ( 'NONE',  ( -39.49588282908369763, -5.935567020298775809, 77.98014135999763141 ) ) ;
#27787=ORIENTED_EDGE ( 'NONE', *, *, #15483, .F. ) ;
#27788=DIRECTION ( 'NONE',  ( 0.000000000000000000, 0.000000000000000000, -1.000000000000000000 ) ) ;
#27791=CARTESIAN_POINT ( 'NONE',  ( -9.880269303432738681, -5.935454207752202116, -3.351769630585352377 ) ) ;
#27801=ADVANCED_FACE ( 'NONE', ( #25122 ), #29854, .T. ) ;
#27805=CARTESIAN_POINT ( 'NONE',  ( 21.09785597605719332, -8.874820941924726370, 47.04930799450051637 ) ) ;
#27818=ORIENTED_EDGE ( 'NONE', *, *, #18336, .T. ) ;
#27821=CARTESIAN_POINT ( 'NONE',  ( 81.55380775071134281, -5.936920032134864300, 77.94194987224879867 ) ) ;
#27827=ORIENTED_EDGE ( 'NONE', *, *, #29810, .T. ) ;
#27830=CARTESIAN_POINT ( 'NONE',  ( -29.27337757263006424, -4.281489722201563985, 13.63563177263803894 ) ) ;
#27832=CYLINDRICAL_SURFACE ( 'NONE', #24771, 2.500000000000002220 ) ;
#27836=ORIENTED_EDGE ( 'NONE', *, *, #26756, .F. ) ;
#27871=ORIENTED_EDGE ( 'NONE', *, *, #31104, .T. ) ;
#27876=ORIENTED_EDGE ( 'NONE', *, *, #16959, .F. ) ;
#27878=ADVANCED_FACE ( 'NONE', ( #14955 ), #16717, .T. ) ;
#27884=ORIENTED_EDGE ( 'NONE', *, *, #15716, .T. ) ;
#27885=DIRECTION ( 'NONE',  ( -0.000000000000000000, -1.000000000000000000, -0.000000000000000000 ) ) ;
#27887=CONICAL_SURFACE ( 'NONE', #8493, 72.00502525316939284, 0.7853981633974482790 ) ;
#27893=ORIENTED_EDGE ( 'NONE', *, *, #17153, .T. ) ;
#27894=CARTESIAN_POINT ( 'NONE',  ( 21.09785597605719332, 16.33322284159648063, -0.3501356754177092911 ) ) ;
#27897=CARTESIAN_POINT ( 'NONE',  ( 54.13680899610202601, 0.4256545730735106781, 100.7294901468369233 ) ) ;
#27898=CARTESIAN_POINT ( 'NONE',  ( 21.09785597605733187, -5.935454207752083988, 47.04930799450051637 ) ) ;
#27904=DIRECTION ( 'NONE',  ( -0.000000000000000000, 1.000000000000000000, -0.000000000000000000 ) ) ;
#27909=ORIENTED_EDGE ( 'NONE', *, *, #337, .F. ) ;
#27912=EDGE_CURVE ( 'NONE', #1878, #16844, #3092, .T. ) ;
#27913=CARTESIAN_POINT ( 'NONE',  ( -30.49450530719115804, 11.01902901830102977, 22.43617484215558022 ) ) ;
#27920=CARTESIAN_POINT ( 'NONE',  ( -38.52112853513683888, -5.935454207752202116, 16.07118271501078510 ) ) ;
#27921=CARTESIAN_POINT ( 'NONE',  ( -45.04500625625952637, -5.676766116611589474, 53.06055232190111326 ) ) ;
#27925=LINE ( 'NONE', #25462, #2880 ) ;
#27931=CARTESIAN_POINT ( 'NONE',  ( 21.09785597605719332, -5.935454207752083988, 47.04930799449963530 ) ) ;
#27938=ORIENTED_EDGE ( 'NONE', *, *, #28464, .T. ) ;
#27942=CARTESIAN_POINT ( 'NONE',  ( -35.49409842342767263, -5.179470286602130713, 14.38986137883322769 ) ) ;
#27955=CARTESIAN_POINT ( 'NONE',  ( -39.41955952844167399, -5.936037113805915588, 77.90964267221822581 ) ) ;
#27967=DIRECTION ( 'NONE',  ( -0.000000000000000000, -1.000000000000000000, -0.000000000000000000 ) ) ;
#27969=CARTESIAN_POINT ( 'NONE',  ( -9.831337038036075171, -5.937394935145314356, 107.7511683020618563 ) ) ;
#27971=FACE_OUTER_BOUND ( 'NONE', #2128, .T. ) ;
#27975=DIRECTION ( 'NONE',  ( 0.000000000000000000, -0.2756373558165849391, -0.9612616959384376880 ) ) ;
#27976=ORIENTED_EDGE ( 'NONE', *, *, #30631, .F. ) ;
#27977=CARTESIAN_POINT ( 'NONE',  ( 74.12754556829368369, -0.2653311271195410437, 80.34416813279683822 ) ) ;
#27980=CARTESIAN_POINT ( 'NONE',  ( -38.21956313268621130, 5.305746783394874377, 42.04930799450051637 ) ) ;
#27983=VERTEX_POINT ( 'NONE', #21466 ) ;
#27992=AXIS2_PLACEMENT_3D ( 'NONE', #24377, #24540, #12080 ) ;
#28003=DIRECTION ( 'NONE',  ( 0.000000000000000000, -1.000000000000000000, 0.000000000000000000 ) ) ;
#28004=CARTESIAN_POINT ( 'NONE',  ( 81.72575882806418690, -5.937394852768786535, 15.98100540722295015 ) ) ;
#28005=ORIENTED_EDGE ( 'NONE', *, *, #29203, .T. ) ;
#28008=CARTESIAN_POINT ( 'NONE',  ( -9.474781401982005136, 5.388785998227653806, 106.8025418868326284 ) ) ;
#28010=CARTESIAN_POINT ( 'NONE',  ( -31.40817747290099859, 3.832457305373850875, 78.38424341102378889 ) ) ;
#28012=EDGE_CURVE ( 'NONE', #28041, #8773, #25920, .T. ) ;
#28013=VERTEX_POINT ( 'NONE', #13310 ) ;
#28020=CARTESIAN_POINT ( 'NONE',  ( 81.71662875395456638, -5.936382080411370055, 16.04580235805854471 ) ) ;
#28028=DIRECTION ( 'NONE',  ( 8.659560562355053653E-17, -0.7071067811865378028, 0.7071067811865573427 ) ) ;
#28038=EDGE_CURVE ( 'NONE', #24958, #10579, #3641, .T. ) ;
#28041=VERTEX_POINT ( 'NONE', #31185 ) ;
#28042=VERTEX_POINT ( 'NONE', #16227 ) ;
#28048=CARTESIAN_POINT ( 'NONE',  ( 52.36191254139992424, -5.922252862938464979, 106.4668663603234933 ) ) ;
#28059=CARTESIAN_POINT ( 'NONE',  ( 45.32414328224286493, 11.18784031540631752, 98.72179417164551296 ) ) ;
#28073=DIRECTION ( 'NONE',  ( 0.000000000000000000, -1.000000000000000000, 0.000000000000000000 ) ) ;
#28076=ORIENTED_EDGE ( 'NONE', *, *, #11776, .F. ) ;
#28086=DIRECTION ( 'NONE',  ( 0.000000000000000000, 0.000000000000000000, -1.000000000000000000 ) ) ;
#28091=CARTESIAN_POINT ( 'NONE',  ( -38.65545646816406133, -5.472247659560185440, 79.55937378679692529 ) ) ;
#28102=CARTESIAN_POINT ( 'NONE',  ( 41.51205063648688309, 1.925589859889728972, 132.0493079945005377 ) ) ;
#28103=CARTESIAN_POINT ( 'NONE',  ( 44.25133798441032695, 11.55977609614116020, 98.10820709097123427 ) ) ;
#28111=CARTESIAN_POINT ( 'NONE',  ( 21.09785597605719332, 25.56454579224779877, 75.54930799450052348 ) ) ;
#28112=CARTESIAN_POINT ( 'NONE',  ( 52.11424208273423631, 4.323180411458207750, 98.49488265617655713 ) ) ;
#28122=CARTESIAN_POINT ( 'NONE',  ( -39.51359738027355206, -5.935454207752198563, 77.87546120947918382 ) ) ;
#28124=EDGE_CURVE ( 'NONE', #28042, #29498, #14106, .T. ) ;
#28136=DIRECTION ( 'NONE',  ( 0.000000000000000000, -1.000000000000000000, 0.000000000000000000 ) ) ;
#28148=CARTESIAN_POINT ( 'NONE',  ( 78.88609142827000653, -5.395280703882846751, 79.46745756311666753 ) ) ;
#28150=DIRECTION ( 'NONE',  ( -4.163336342344333082E-15, 0.000000000000000000, 1.000000000000000000 ) ) ;
#28154=CARTESIAN_POINT ( 'NONE',  ( -10.70116484021380643, -5.771419034597320419, -11.48608978375909651 ) ) ;
#28155=CYLINDRICAL_SURFACE ( 'NONE', #31426, 84.30000000000001137 ) ;
#28164=DIRECTION ( 'NONE',  ( 0.000000000000000000, -1.000000000000000000, -0.000000000000000000 ) ) ;
#28172=CARTESIAN_POINT ( 'NONE',  ( -36.49977054276610033, -5.245772846439738402, 79.63610610625367769 ) ) ;
#28178=DIRECTION ( 'NONE',  ( 0.000000000000000000, 0.000000000000000000, 1.000000000000000000 ) ) ;
#28184=DIRECTION ( 'NONE',  ( 0.000000000000000000, -1.000000000000000000, 0.000000000000000000 ) ) ;
#28192=VERTEX_POINT ( 'NONE', #29037 ) ;
#28204=ADVANCED_FACE ( 'NONE', ( #22443 ), #27752, .F. ) ;
#28208=CARTESIAN_POINT ( 'NONE',  ( 52.14324879758525100, -5.938447472589719389, 106.6451039912369225 ) ) ;
#28217=ORIENTED_EDGE ( 'NONE', *, *, #31509, .T. ) ;
#28219=CARTESIAN_POINT ( 'NONE',  ( 53.82666426033320306, 1.147918989839220805, 100.4501361902863010 ) ) ;
#28226=CARTESIAN_POINT ( 'NONE',  ( 21.09785597605719332, -19.93545420775220123, 47.04930799450051637 ) ) ;
#28231=ORIENTED_EDGE ( 'NONE', *, *, #26049, .F. ) ;
#28233=DIRECTION ( 'NONE',  ( 0.000000000000000000, -1.000000000000000000, -0.000000000000000000 ) ) ;
#28244=CARTESIAN_POINT ( 'NONE',  ( 21.09785597605719332, -16.63545420775219696, 47.04930799450051637 ) ) ;
#28248=FACE_OUTER_BOUND ( 'NONE', #32495, .T. ) ;
#28252=DIRECTION ( 'NONE',  ( -0.000000000000000000, -1.000000000000000000, -0.000000000000000000 ) ) ;
#28257=DIRECTION ( 'NONE',  ( -0.000000000000000000, -1.000000000000000000, -0.000000000000000000 ) ) ;
#28265=DIRECTION ( 'NONE',  ( 1.000000000000000000, -0.000000000000000000, 1.224646799147353207E-16 ) ) ;
#28266=ORIENTED_EDGE ( 'NONE', *, *, #18119, .F. ) ;
#28276=CARTESIAN_POINT ( 'NONE',  ( -39.41422314775386582, -5.935690916112652538, 77.97410326138991365 ) ) ;
#28277=AXIS2_PLACEMENT_3D ( 'NONE', #14626, #19698, #7409 ) ;
#28282=DIRECTION ( 'NONE',  ( 0.000000000000000000, 0.000000000000000000, -1.000000000000000000 ) ) ;
#28283=CIRCLE ( 'NONE', #27747, 55.85791022362053582 ) ;
#28286=DIRECTION ( 'NONE',  ( -0.000000000000000000, -1.000000000000000000, -0.000000000000000000 ) ) ;
#28300=DIRECTION ( 'NONE',  ( -0.000000000000000000, 1.000000000000000000, -0.000000000000000000 ) ) ;
#28311=FACE_OUTER_BOUND ( 'NONE', #15466, .T. ) ;
#28317=DIRECTION ( 'NONE',  ( -0.000000000000000000, -1.000000000000000000, -0.000000000000000000 ) ) ;
#28325=CIRCLE ( 'NONE', #20967, 65.75844861871132707 ) ;
#28329=DIRECTION ( 'NONE',  ( 0.000000000000000000, 0.000000000000000000, 1.000000000000000000 ) ) ;
#28331=ORIENTED_EDGE ( 'NONE', *, *, #21691, .T. ) ;
#28335=FACE_OUTER_BOUND ( 'NONE', #30477, .T. ) ;
#28336=CARTESIAN_POINT ( 'NONE',  ( -31.70221225902718842, 2.889067130208885725, 78.90943617797866239 ) ) ;
#28339=CARTESIAN_POINT ( 'NONE',  ( 21.09785597605719332, -5.721341737285094098, 47.04930799450051637 ) ) ;
#28342=CARTESIAN_POINT ( 'NONE',  ( 106.0978559760576161, -5.935454207751966749, 16.07118271501087747 ) ) ;
#28348=DIRECTION ( 'NONE',  ( -1.313185983435984691E-29, 1.000000000000000000, 3.761114140369702165E-15 ) ) ;
#28355=EDGE_CURVE ( 'NONE', #9654, #16844, #31632, .T. ) ;
#28356=ORIENTED_EDGE ( 'NONE', *, *, #28124, .F. ) ;
#28357=VECTOR ( 'NONE', #17338, 1000.000000000000000 ) ;
#28363=CARTESIAN_POINT ( 'NONE',  ( -12.56040783456439414, -3.386628651588886818, 102.8267921593860450 ) ) ;
#28364=B_SPLINE_CURVE_WITH_KNOTS ( 'NONE', 3,
 ( #18570, #31385, #3480, #18891, #28927, #16437, #23510, #8259, #8420, #5960, #28596, #3154 ),
 .UNSPECIFIED., .F., .F.,
 ( 4, 2, 2, 2, 2, 4 ),
 ( 0.0003195369756188888837, 0.0003994212195236132188, 0.0004793054634283375540, 0.0005192475853806903432, 0.0005591897073330432408, 0.0006390739512377632391 ),
 .UNSPECIFIED. ) ;
#28366=EDGE_CURVE ( 'NONE', #27012, #7822, #3845, .T. ) ;
#28375=CARTESIAN_POINT ( 'NONE',  ( 52.99971320245913375, -5.721341737285090545, 105.3293216028873616 ) ) ;
#28377=ORIENTED_EDGE ( 'NONE', *, *, #6998, .T. ) ;
#28382=CARTESIAN_POINT ( 'NONE',  ( 53.65899080383296393, 1.504766047489273451, 100.3208885721442698 ) ) ;
#28414=DIRECTION ( 'NONE',  ( 0.000000000000000000, 0.000000000000000000, 1.000000000000000000 ) ) ;
#28430=AXIS2_PLACEMENT_3D ( 'NONE', #6609, #19062, #13557 ) ;
#28433=CARTESIAN_POINT ( 'NONE',  ( 21.09785597605720042, 12.11061942510878886, 102.5807244896116401 ) ) ;
#28438=CARTESIAN_POINT ( 'NONE',  ( -39.44085990154519550, -5.935843268867586175, 77.89403126197323957 ) ) ;
#28451=FACE_BOUND ( 'NONE', #4548, .T. ) ;
#28455=CARTESIAN_POINT ( 'NONE',  ( 45.85510844531590635, 10.95165879486606642, 97.72497336462666340 ) ) ;
#28459=B_SPLINE_CURVE_WITH_KNOTS ( 'NONE', 3,
 ( #2196, #25332, #32239, #700, #21030, #536, #10882, #28276, #13504, #10567, #23017, #17935, #20557, #30587, #5796, #5957, #7940, #15951, #15800, #13666, #25807, #3317, #8100, #25961, #27955, #13347, #28438, #18094, #23348, #2991, #20874, #859, #11044, #28122 ),
 .UNSPECIFIED., .F., .F.,
 ( 4, 3, 3, 3, 3, 3, 3, 3, 3, 3, 3, 4 ),
 ( 0.0002238713945714089102, 0.0002443349429672130708, 0.0002647477377446432801, 0.0002776748598345243793, 0.0002880592449434732339, 0.0002985192223745329241, 0.0003079983821794234989, 0.0003223271915421464210, 0.0003453054321472419971, 0.0003848690401466044967, 0.0004381801683341408253, 0.0004477427891427999311 ),
 .UNSPECIFIED. ) ;
#28464=EDGE_CURVE ( 'NONE', #17233, #29191, #28325, .T. ) ;
#28467=CARTESIAN_POINT ( 'NONE',  ( 76.38709588317641419, -2.706209967030163366, 80.78504949309299832 ) ) ;
#28487=CARTESIAN_POINT ( 'NONE',  ( -34.62367702067368924, -4.391527280237080610, 80.32849845693385760 ) ) ;
#28492=VERTEX_POINT ( 'NONE', #15817 ) ;
#28494=DIRECTION ( 'NONE',  ( 0.000000000000000000, -1.000000000000000000, 0.000000000000000000 ) ) ;
#28496=CARTESIAN_POINT ( 'NONE',  ( -33.33845461267002008, -1.245420574899409383, 80.62684019938389213 ) ) ;
#28519=CARTESIAN_POINT ( 'NONE',  ( -10.01616728275229740, -5.935340315990530691, -13.57859485750651629 ) ) ;
#28523=CARTESIAN_POINT ( 'NONE',  ( -12.63788552253510211, -2.706209967029991503, 102.3385479016197479 ) ) ;
#28536=ORIENTED_EDGE ( 'NONE', *, *, #12094, .T. ) ;
#28539=EDGE_LOOP ( 'NONE', ( #17264, #18507, #21058, #31575 ) ) ;
#28541=CARTESIAN_POINT ( 'NONE',  ( 52.73954714899677754, 3.260977705924045011, 99.74023595452713664 ) ) ;
#28543=VECTOR ( 'NONE', #1028, 1000.000000000000000 ) ;
#28563=CIRCLE ( 'NONE', #29620, 71.99999999999998579 ) ;
#28567=DIRECTION ( 'NONE',  ( -0.000000000000000000, 1.000000000000000000, -0.000000000000000000 ) ) ;
#28568=AXIS2_PLACEMENT_3D ( 'NONE', #30059, #27589, #27253 ) ;
#28569=ORIENTED_EDGE ( 'NONE', *, *, #11811, .T. ) ;
#28576=CARTESIAN_POINT ( 'NONE',  ( 106.0978559760576161, -5.935454207752202116, 16.07118271501088458 ) ) ;
#28596=CARTESIAN_POINT ( 'NONE',  ( 51.92400919103565116, -5.935454207752203892, -13.58917618696519725 ) ) ;
#28605=DIRECTION ( 'NONE',  ( 1.000000000000000000, -0.000000000000000000, -0.000000000000000000 ) ) ;
#28610=EDGE_CURVE ( 'NONE', #10609, #14793, #12875, .T. ) ;
#28613=SURFACE_SIDE_STYLE ('',( #18585 ) ) ;
#28627=CARTESIAN_POINT ( 'NONE',  ( 72.46310410352296572, 9.702389020015065313, 20.34850893876554778 ) ) ;
#28630=CARTESIAN_POINT ( 'NONE',  ( 49.03810302523404374, 8.582373042058245360, -4.360755707720810115 ) ) ;
#28636=EDGE_CURVE ( 'NONE', #7566, #28192, #25146, .T. ) ;
#28641=CARTESIAN_POINT ( 'NONE',  ( 81.73558347630492449, -5.936245040125570860, 78.00362224660160848 ) ) ;
#28645=FACE_OUTER_BOUND ( 'NONE', #981, .T. ) ;
#28651=ORIENTED_EDGE ( 'NONE', *, *, #6400, .F. ) ;
#28656=DIRECTION ( 'NONE',  ( 0.000000000000000000, 0.000000000000000000, -1.000000000000000000 ) ) ;
#28665=CARTESIAN_POINT ( 'NONE',  ( -44.16023901230963133, -5.485428030315304682, 41.32037469003774532 ) ) ;
#28666=AXIS2_PLACEMENT_3D ( 'NONE', #19682, #27235, #14777 ) ;
#28672=ORIENTED_EDGE ( 'NONE', *, *, #18119, .T. ) ;
#28682=DIRECTION ( 'NONE',  ( 0.000000000000000000, 0.000000000000000000, 1.000000000000000000 ) ) ;
#28687=CARTESIAN_POINT ( 'NONE',  ( 21.09785597605719332, 25.56454579224780232, 126.2593585008393831 ) ) ;
#28701=DIRECTION ( 'NONE',  ( -1.000000000000000000, 0.000000000000000000, 0.000000000000000000 ) ) ;
#28703=ORIENTED_EDGE ( 'NONE', *, *, #18469, .F. ) ;
#28727=CARTESIAN_POINT ( 'NONE',  ( 72.46537437338240295, 9.162376348828955130, 19.70867165547888789 ) ) ;
#28731=AXIS2_PLACEMENT_3D ( 'NONE', #14970, #12682, #24972 ) ;
#28734=FACE_OUTER_BOUND ( 'NONE', #24529, .T. ) ;
#28752=ADVANCED_FACE ( 'NONE', ( #28734 ), #3301, .F. ) ;
#28774=B_SPLINE_CURVE_WITH_KNOTS ( 'NONE', 3,
 ( #23366, #30604, #10417, #13368, #235, #10898, #23035, #18265, #12892, #20896, #18428, #15498 ),
 .UNSPECIFIED., .F., .F.,
 ( 4, 2, 2, 2, 2, 4 ),
 ( 0.0003422200191418650270, 0.002082436906217388032, 0.003822653793292911037, 0.005562870680368433608, 0.006432979123906195328, 0.007303087567443957047 ),
 .UNSPECIFIED. ) ;
#28786=DIRECTION ( 'NONE',  ( 0.000000000000000000, 0.000000000000000000, -1.000000000000000000 ) ) ;
#28787=CARTESIAN_POINT ( 'NONE',  ( 47.79865503179234310, 9.702389020015065313, 97.45038561958638468 ) ) ;
#28804=CARTESIAN_POINT ( 'NONE',  ( -34.43190828144128091, -4.192658519183404486, 80.43389084567178315 ) ) ;
#28805=CARTESIAN_POINT ( 'NONE',  ( 21.09785597605719332, 11.92558985988973497, 47.04930799450051637 ) ) ;
#28806=AXIS2_PLACEMENT_3D ( 'NONE', #5505, #8131, #25520 ) ;
#28819=AXIS2_PLACEMENT_3D ( 'NONE', #30761, #25663, #3335 ) ;
#28822=CARTESIAN_POINT ( 'NONE',  ( 21.09785597605719332, 25.56454579224779877, 47.04930799450051637 ) ) ;
#28829=LINE ( 'NONE', #3720, #24013 ) ;
#28832=VECTOR ( 'NONE', #30555, 1000.000000000000000 ) ;
#28846=CONICAL_SURFACE ( 'NONE', #31471, 39.63553620740810857, 0.6632251157578421541 ) ;
#28862=CARTESIAN_POINT ( 'NONE',  ( 21.09785597605719332, -15.93545420775219945, 119.0493079945005093 ) ) ;
#28864=FACE_BOUND ( 'NONE', #21244, .T. ) ;
#28866=CARTESIAN_POINT ( 'NONE',  ( 0.1369267683895796783, 11.91444431924556469, -5.596515685912667237 ) ) ;
#28880=VERTEX_POINT ( 'NONE', #22146 ) ;
#28893=AXIS2_PLACEMENT_3D ( 'NONE', #24080, #21615, #1600 ) ;
#28896=CARTESIAN_POINT ( 'NONE',  ( -36.45222641229887017, 9.925589859889722533, 42.04930799450051637 ) ) ;
#28897=DIRECTION ( 'NONE',  ( 0.000000000000000000, 0.000000000000000000, 1.000000000000000000 ) ) ;
#28903=CARTESIAN_POINT ( 'NONE',  ( 21.09785597605719332, -15.93545420775219945, 47.04930799450051637 ) ) ;
#28906=AXIS2_PLACEMENT_3D ( 'NONE', #19927, #2046, #9770 ) ;
#28917=CARTESIAN_POINT ( 'NONE',  ( -12.31990217110675800, -4.114116020023733888, -9.341889586185132544 ) ) ;
#28927=CARTESIAN_POINT ( 'NONE',  ( 52.03879352760534260, -5.936629510748245409, -13.61281336867091696 ) ) ;
#28941=ORIENTED_EDGE ( 'NONE', *, *, #3195, .T. ) ;
#28949=LINE ( 'NONE', #16134, #4780 ) ;
#28955=ORIENTED_EDGE ( 'NONE', *, *, #1578, .T. ) ;
#28970=CARTESIAN_POINT ( 'NONE',  ( 52.02704899015044759, -5.937394935145313468, -13.39445452378610568 ) ) ;
#28977=FACE_OUTER_BOUND ( 'NONE', #20953, .T. ) ;
#28979=CARTESIAN_POINT ( 'NONE',  ( 21.09785597605719332, 25.56454579224779877, 23.54930799450051637 ) ) ;
#28980=EDGE_CURVE ( 'NONE', #16546, #5971, #13964, .T. ) ;
#28981=DIRECTION ( 'NONE',  ( -0.000000000000000000, 1.000000000000000000, -0.000000000000000000 ) ) ;
#29002=AXIS2_PLACEMENT_3D ( 'NONE', #13003, #4961, #7916 ) ;
#29019=DIRECTION ( 'NONE',  ( -0.000000000000000000, -0.000000000000000000, -1.000000000000000000 ) ) ;
#29027=ORIENTED_EDGE ( 'NONE', *, *, #3292, .F. ) ;
#29030=DIRECTION ( 'NONE',  ( -0.000000000000000000, 1.000000000000000000, -0.000000000000000000 ) ) ;
#29031=CARTESIAN_POINT ( 'NONE',  ( 21.09785597605720042, 12.39166260509097484, 101.6006104443987397 ) ) ;
#29037=CARTESIAN_POINT ( 'NONE',  ( 21.09785597605719687, 25.56454579224779877, 27.04930799450051637 ) ) ;
#29041=VERTEX_POINT ( 'NONE', #22641 ) ;
#29050=CARTESIAN_POINT ( 'NONE',  ( 77.89472409461923519, -4.535950511381784622, 13.85981127911711575 ) ) ;
#29056=FACE_BOUND ( 'NONE', #13905, .T. ) ;
#29058=CARTESIAN_POINT ( 'NONE',  ( -45.63949534714383560, -5.900352476715130301, 40.43365730525594870 ) ) ;
#29067=ORIENTED_EDGE ( 'NONE', *, *, #12911, .T. ) ;
#29076=EDGE_CURVE ( 'NONE', #16751, #29171, #32398, .T. ) ;
#29080=FACE_OUTER_BOUND ( 'NONE', #27045, .T. ) ;
#29085=ORIENTED_EDGE ( 'NONE', *, *, #10627, .T. ) ;
#29090=CARTESIAN_POINT ( 'NONE',  ( 21.09785597605719332, 12.06852548259731961, 47.04930799450051637 ) ) ;
#29099=ORIENTED_EDGE ( 'NONE', *, *, #21763, .F. ) ;
#29102=VECTOR ( 'NONE', #8311, 1000.000000000000000 ) ;
#29104=CARTESIAN_POINT ( 'NONE',  ( 21.09785597605719332, -5.721341737285094098, 47.04930799450051637 ) ) ;
#29106=CIRCLE ( 'NONE', #17576, 47.39944366991822733 ) ;
#29109=CARTESIAN_POINT ( 'NONE',  ( -39.54762467759688604, -5.935999211605547998, 77.95416007536729808 ) ) ;
#29119=ORIENTED_EDGE ( 'NONE', *, *, #18608, .T. ) ;
#29130=CARTESIAN_POINT ( 'NONE',  ( -29.57396024870593365, 10.91176617787883174, 71.86136379807102514 ) ) ;
#29134=CARTESIAN_POINT ( 'NONE',  ( 51.97542764375435809, -5.937448199248382075, -13.39445452378610568 ) ) ;
#29148=ORIENTED_EDGE ( 'NONE', *, *, #6998, .F. ) ;
#29152=AXIS2_PLACEMENT_3D ( 'NONE', #19853, #7717, #4770 ) ;
#29157=B_SPLINE_CURVE_WITH_KNOTS ( 'NONE', 3,
 ( #27543, #24921, #12618, #2434 ),
 .UNSPECIFIED., .F., .F.,
 ( 4, 4 ),
 ( 0.07560733880179559829, 0.09146776418496910255 ),
 .UNSPECIFIED. ) ;
#29171=VERTEX_POINT ( 'NONE', #21295 ) ;
#29178=CIRCLE ( 'NONE', #7157, 55.72436264418301732 ) ;
#29186=CYLINDRICAL_SURFACE ( 'NONE', #19715, 2.000000000000001776 ) ;
#29191=VERTEX_POINT ( 'NONE', #8520 ) ;
#29203=EDGE_CURVE ( 'NONE', #2086, #8185, #23293, .T. ) ;
#29214=VERTEX_POINT ( 'NONE', #31326 ) ;
#29218=TOROIDAL_SURFACE ( 'NONE', #26589, 39.69941114636694834, 0.3000000000000000444 ) ;
#29226=ORIENTED_EDGE ( 'NONE', *, *, #7398, .F. ) ;
#29233=EDGE_CURVE ( 'NONE', #29041, #24330, #17499, .T. ) ;
#29239=EDGE_CURVE ( 'NONE', #13343, #8733, #10677, .T. ) ;
#29244=CYLINDRICAL_SURFACE ( 'NONE', #17718, 55.00000000000000000 ) ;
#29245=CARTESIAN_POINT ( 'NONE',  ( 53.31593463385092235, -5.523138741469208135, -10.01380679907181737 ) ) ;
#29246=FACE_BOUND ( 'NONE', #21153, .T. ) ;
#29264=CARTESIAN_POINT ( 'NONE',  ( -39.55665669155531106, -5.935685895218067998, 77.88576325833030012 ) ) ;
#29265=CARTESIAN_POINT ( 'NONE',  ( -63.90214402394282445, 9.925589859889736744, 40.04930799450051637 ) ) ;
#29271=ADVANCED_FACE ( 'NONE', ( #3425 ), #19646, .F. ) ;
#29275=CARTESIAN_POINT ( 'NONE',  ( 56.35714053840848692, -3.295808585244882849, 106.7232700815558957 ) ) ;
#29281=CARTESIAN_POINT ( 'NONE',  ( 52.07598125554711999, -5.935454207752202116, 107.4212530892143889 ) ) ;
#29304=VERTEX_POINT ( 'NONE', #21943 ) ;
#29307=ORIENTED_EDGE ( 'NONE', *, *, #7381, .T. ) ;
#29322=ORIENTED_EDGE ( 'NONE', *, *, #25885, .T. ) ;
#29333=CARTESIAN_POINT ( 'NONE',  ( -12.57649835094935931, -1.714651486836148209, -6.690735631693065066 ) ) ;
#29341=FACE_BOUND ( 'NONE', #18258, .T. ) ;
#29343=VECTOR ( 'NONE', #26408, 1000.000000000000114 ) ;
#29361=ORIENTED_EDGE ( 'NONE', *, *, #27488, .T. ) ;
#29365=EDGE_LOOP ( 'NONE', ( #10378, #16782, #2709, #7923, #12181 ) ) ;
#29367=DIRECTION ( 'NONE',  ( 0.000000000000000000, 0.000000000000000000, -1.000000000000000000 ) ) ;
#29369=DIRECTION ( 'NONE',  ( 0.000000000000000000, -1.000000000000000000, 0.000000000000000000 ) ) ;
#29370=CARTESIAN_POINT ( 'NONE',  ( 51.92400919103565116, -5.935454207752198563, -11.03616215687537583 ) ) ;
#29372=ORIENTED_EDGE ( 'NONE', *, *, #10970, .T. ) ;
#29381=FACE_BOUND ( 'NONE', #13473, .T. ) ;
#29383=CARTESIAN_POINT ( 'NONE',  ( -45.38828485498197551, -5.820282895468940509, 40.73516372632767002 ) ) ;
#29390=AXIS2_PLACEMENT_3D ( 'NONE', #28822, #26517, #4029 ) ;
#29394=ADVANCED_FACE ( 'NONE', ( #7522 ), #11590, .T. ) ;
#29396=CARTESIAN_POINT ( 'NONE',  ( -11.63095230821880044, 1.147918989839226578, -6.351520201285235423 ) ) ;
#29410=CARTESIAN_POINT ( 'NONE',  ( 73.54637414377801008, 11.88152873911358753, 68.55296476473189671 ) ) ;
#29412=ORIENTED_EDGE ( 'NONE', *, *, #2449, .T. ) ;
#29418=CARTESIAN_POINT ( 'NONE',  ( 54.39271611435331977, -0.2653311271195929466, -5.980381597736087684 ) ) ;
#29425=CARTESIAN_POINT ( 'NONE',  ( -10.01358589504979513, -5.935454207834595763, -13.41617548937563598 ) ) ;
#29427=ORIENTED_EDGE ( 'NONE', *, *, #11344, .F. ) ;
#29435=ORIENTED_EDGE ( 'NONE', *, *, #13865, .F. ) ;
#29436=CARTESIAN_POINT ( 'NONE',  ( -39.57232266946287780, -5.935998081906530111, 77.90559678797934851 ) ) ;
#29445=FACE_OUTER_BOUND ( 'NONE', #29365, .T. ) ;
#29452=ORIENTED_EDGE ( 'NONE', *, *, #2553, .T. ) ;
#29457=CARTESIAN_POINT ( 'NONE',  ( -30.89191207862503674, 11.92558985988972609, 67.47405476605740660 ) ) ;
#29459=CARTESIAN_POINT ( 'NONE',  ( 21.09785597605719332, -19.93545420775220123, 47.04930799450051637 ) ) ;
#29467=LINE ( 'NONE', #12560, #19995 ) ;
#29468=DIRECTION ( 'NONE',  ( 0.000000000000000000, 0.000000000000000000, -1.000000000000000000 ) ) ;
#29471=CARTESIAN_POINT ( 'NONE',  ( 79.10241889060681331, -5.935454207752202116, 16.07118271501078510 ) ) ;
#29481=CARTESIAN_POINT ( 'NONE',  ( -63.90214402394282445, -5.935454207752198563, 77.87546120947918382 ) ) ;
#29487=EDGE_LOOP ( 'NONE', ( #14418, #26521, #25428, #3406, #2635 ) ) ;
#29488=STYLED_ITEM('',(#32515),#1464);
#29489=ORIENTED_EDGE ( 'NONE', *, *, #16961, .T. ) ;
#29492=B_SPLINE_CURVE_WITH_KNOTS ( 'NONE', 3,
 ( #6725, #21815, #4093, #1800, #4426, #32000, #29050, #13797, #3945, #23953, #24120, #14448, #14287, #1469, #21652, #6571, #1636, #16564, #1957, #3775, #11660, #31680, #8863, #26265, #21970, #11487, #6243, #24284, #19021, #11823, #9519, #21484, #31835, #28727, #21318, #31523 ),
 .UNSPECIFIED., .F., .F.,
 ( 4, 2, 2, 2, 2, 2, 2, 2, 2, 2, 2, 2, 2, 2, 2, 2, 2, 4 ),
 ( 2.453269466693398698E-18, 0.001253900128824240621, 0.001880850193236375352, 0.002507800257648510299, 0.003134750322060645029, 0.003761700386472778893, 0.005015600515297048353, 0.005642550579709183084, 0.006269500644121316947, 0.007523400772945588143, 0.008777300901769856736, 0.01003120103059412793, 0.01253900128824268247, 0.01504680154589123874, 0.01630070167471552034, 0.01755460180353980021, 0.01880850193236408008, 0.02006240206118835995 ),
 .UNSPECIFIED. ) ;
#29498=VERTEX_POINT ( 'NONE', #18483 ) ;
#29522=DIRECTION ( 'NONE',  ( 0.000000000000000000, 1.420067270486643379E-16, -1.000000000000000000 ) ) ;
#29537=VERTEX_POINT ( 'NONE', #11271 ) ;
#29539=CARTESIAN_POINT ( 'NONE',  ( 47.79865503179234310, 9.702389020015065313, -3.337848843846767721 ) ) ;
#29546=CARTESIAN_POINT ( 'NONE',  ( -9.880269303432738681, -5.935454207752202116, -13.48461434800281289 ) ) ;
#29549=DIRECTION ( 'NONE',  ( -1.000000000000000000, -0.000000000000000000, -3.491481338843133355E-15 ) ) ;
#29565=CARTESIAN_POINT ( 'NONE',  ( -10.80400125034478087, -5.721341737285083440, -11.23070561388631816 ) ) ;
#29573=LINE ( 'NONE', #23824, #13506 ) ;
#29578=ORIENTED_EDGE ( 'NONE', *, *, #21005, .F. ) ;
#29584=FACE_BOUND ( 'NONE', #21190, .T. ) ;
#29585=DIRECTION ( 'NONE',  ( 0.000000000000000000, 0.000000000000000000, 1.000000000000000000 ) ) ;
#29587=DIRECTION ( 'NONE',  ( 0.000000000000000000, 0.000000000000000000, -1.000000000000000000 ) ) ;
#29589=DIRECTION ( 'NONE',  ( 0.000000000000000000, 0.000000000000000000, 1.000000000000000000 ) ) ;
#29590=ORIENTED_EDGE ( 'NONE', *, *, #30020, .T. ) ;
#29592=CARTESIAN_POINT ( 'NONE',  ( -30.11252088733392895, 11.69089543585256230, 24.41124053607467559 ) ) ;
#29613=CARTESIAN_POINT ( 'NONE',  ( 52.21187923486668581, -5.935340315990531579, 107.4212530892143889 ) ) ;
#29614=ORIENTED_EDGE ( 'NONE', *, *, #20159, .T. ) ;
#29616=AXIS2_PLACEMENT_3D ( 'NONE', #31357, #3944, #24119 ) ;
#29620=AXIS2_PLACEMENT_3D ( 'NONE', #18543, #16090, #3620 ) ;
#29622=AXIS2_PLACEMENT_3D ( 'NONE', #21738, #6815, #24368 ) ;
#29623=AXIS2_PLACEMENT_3D ( 'NONE', #14654, #14044, #12192 ) ;
#29630=CARTESIAN_POINT ( 'NONE',  ( 72.32087091261323053, 11.70027025134008625, 69.64590718380839007 ) ) ;
#29633=DIRECTION ( 'NONE',  ( -0.000000000000000000, -1.000000000000000000, -0.000000000000000000 ) ) ;
#29639=CARTESIAN_POINT ( 'NONE',  ( 21.09785597605719332, 15.56454579224779877, 47.04930799450051637 ) ) ;
#29651=VECTOR ( 'NONE', #25344, 1000.000000000000000 ) ;
#29659=CARTESIAN_POINT ( 'NONE',  ( 78.07303900989995782, -5.485531640240845164, 14.71629385678478741 ) ) ;
#29660=CARTESIAN_POINT ( 'NONE',  ( -44.30819669882302492, -5.921088224254131838, 53.77189712903503960 ) ) ;
#29665=CARTESIAN_POINT ( 'NONE',  ( -5.602943079677954685, 9.702389020015065313, 97.51081847724526597 ) ) ;
#29667=CARTESIAN_POINT ( 'NONE',  ( -34.19711200706005627, -2.717459485359273508, 13.31095004307637097 ) ) ;
#29672=CARTESIAN_POINT ( 'NONE',  ( 81.54161849434414933, -5.937448199248381187, 77.92687966219790496 ) ) ;
#29682=FACE_OUTER_BOUND ( 'NONE', #99, .T. ) ;
#29687=CARTESIAN_POINT ( 'NONE',  ( -38.57628410747783221, 11.92558985988973497, 26.63511333407100778 ) ) ;
#29689=ORIENTED_EDGE ( 'NONE', *, *, #10404, .F. ) ;
#29690=DIRECTION ( 'NONE',  ( -0.000000000000000000, -1.000000000000000000, -0.000000000000000000 ) ) ;
#29709=ORIENTED_EDGE ( 'NONE', *, *, #14598, .F. ) ;
#29717=EDGE_LOOP ( 'NONE', ( #31182, #7514, #274, #19956, #32121, #11259 ) ) ;
#29718=CARTESIAN_POINT ( 'NONE',  ( 100.3079064823960493, 25.56454579224780232, 49.54930799450134771 ) ) ;
#29727=CARTESIAN_POINT ( 'NONE',  ( 21.09785597605719332, -15.43545420775221366, 47.04930799450051637 ) ) ;
#29730=VECTOR ( 'NONE', #7903, 1000.000000000000114 ) ;
#29743=DIRECTION ( 'NONE',  ( 0.000000000000000000, -1.000000000000000000, 0.000000000000000000 ) ) ;
#29755=DIRECTION ( 'NONE',  ( 0.000000000000000000, -1.000000000000000000, 0.000000000000000000 ) ) ;
#29763=VERTEX_POINT ( 'NONE', #7314 ) ;
#29765=CARTESIAN_POINT ( 'NONE',  ( -39.57405207560572791, -5.935416493863505671, 77.98611552785908430 ) ) ;
#29778=B_SPLINE_CURVE_WITH_KNOTS ( 'NONE', 3,
 ( #25231, #29998, #22595, #14897, #17833, #20288, #15216, #114, #10136, #7513 ),
 .UNSPECIFIED., .F., .F.,
 ( 4, 2, 2, 2, 4 ),
 ( 0.000000000000000000, 0.0008384749106984304813, 0.001257712366047627778, 0.001467331093722245563, 0.001676949821396863131 ),
 .UNSPECIFIED. ) ;
#29782=AXIS2_PLACEMENT_3D ( 'NONE', #24552, #29821, #29982 ) ;
#29791=DIRECTION ( 'NONE',  ( 0.000000000000000000, -0.2756373558169902815, -0.9612616959383214477 ) ) ;
#29793=CARTESIAN_POINT ( 'NONE',  ( 77.87624645123068490, -5.321843574075664662, 79.54248989857433116 ) ) ;
#29810=EDGE_CURVE ( 'NONE', #1894, #13157, #17365, .T. ) ;
#29811=VERTEX_POINT ( 'NONE', #9780 ) ;
#29816=ORIENTED_EDGE ( 'NONE', *, *, #20850, .T. ) ;
#29820=EDGE_CURVE ( 'NONE', #10313, #31117, #2166, .T. ) ;
#29821=DIRECTION ( 'NONE',  ( -0.000000000000000000, 1.000000000000000000, -0.000000000000000000 ) ) ;
#29833=CARTESIAN_POINT ( 'NONE',  ( -36.50219711772859910, -5.247624208983634908, 14.46472410127245212 ) ) ;
#29849=AXIS2_PLACEMENT_3D ( 'NONE', #18197, #5259, #15269 ) ;
#29854=CONICAL_SURFACE ( 'NONE', #4152, 40.18714373493281755, 0.6632251157578421541 ) ;
#29868=DIRECTION ( 'NONE',  ( -0.000000000000000000, -0.000000000000000000, 1.000000000000000000 ) ) ;
#29872=ORIENTED_EDGE ( 'NONE', *, *, #27674, .T. ) ;
#29877=DIRECTION ( 'NONE',  ( 0.000000000000000000, 0.000000000000000000, -1.000000000000000000 ) ) ;
#29880=CARTESIAN_POINT ( 'NONE',  ( 52.18101245946036215, -5.931148802125862041, -12.49820992465276603 ) ) ;
#29882=ORIENTED_EDGE ( 'NONE', *, *, #6408, .F. ) ;
#29899=CONICAL_SURFACE ( 'NONE', #16314, 67.99999999999998579, 0.5061454830783623793 ) ;
#29912=CARTESIAN_POINT ( 'NONE',  ( 54.51844488531325084, -0.6526263882323822818, -6.154918745024390070 ) ) ;
#29919=CARTESIAN_POINT ( 'NONE',  ( 21.09785597605719332, -15.93545420775219945, -32.16074251183835031 ) ) ;
#29926=CIRCLE ( 'NONE', #28277, 67.18681090792856025 ) ;
#29930=CARTESIAN_POINT ( 'NONE',  ( 54.75981606833478565, -3.374355247260691471, 101.8796202869974508 ) ) ;
#29942=VERTEX_POINT ( 'NONE', #1050 ) ;
#29945=VECTOR ( 'NONE', #14208, 1000.000000000000000 ) ;
#29962=CARTESIAN_POINT ( 'NONE',  ( 71.60189677428111565, 8.508769500014674136, 75.06167927591030775 ) ) ;
#29970=DIRECTION ( 'NONE',  ( -0.000000000000000000, 1.000000000000000000, -0.000000000000000000 ) ) ;
#29979=VERTEX_POINT ( 'NONE', #15833 ) ;
#29982=DIRECTION ( 'NONE',  ( 0.000000000000000000, 0.000000000000000000, -1.000000000000000000 ) ) ;
#29986=CARTESIAN_POINT ( 'NONE',  ( 74.63411498000290578, -1.331120222581886559, 13.45026064251962694 ) ) ;
#29989=DIRECTION ( 'NONE',  ( -0.000000000000000000, 1.000000000000000000, -0.000000000000000000 ) ) ;
#29993=CARTESIAN_POINT ( 'NONE',  ( -58.11219453028166981, 25.56454579224780232, 44.54930799450023216 ) ) ;
#29994=ORIENTED_EDGE ( 'NONE', *, *, #7805, .F. ) ;
#29995=CARTESIAN_POINT ( 'NONE',  ( -9.930143012320160167, -5.943281723642242831, 105.0325699373949249 ) ) ;
#29997=CARTESIAN_POINT ( 'NONE',  ( -30.26475270700094811, 9.131486844526902402, 19.66223557630849328 ) ) ;
#29998=CARTESIAN_POINT ( 'NONE',  ( 79.63325375431691100, -5.771419034597325748, 15.25028717822974222 ) ) ;
#30006=AXIS2_PLACEMENT_3D ( 'NONE', #4307, #9726, #29585 ) ;
#30020=EDGE_CURVE ( 'NONE', #6712, #14793, #6947, .T. ) ;
#30021=CIRCLE ( 'NONE', #5382, 65.75844861871132707 ) ;
#30022=B_SPLINE_SURFACE_WITH_KNOTS ( 'NONE', 3, 1, ( 
 ( #4504, #2961 ),
 ( #10207, #12059 ),
 ( #13158, #5599 ),
 ( #12679, #22496 ),
 ( #5442, #189 ),
 ( #8072, #3120 ),
 ( #15288, #7739 ),
 ( #5111, #501 ),
 ( #31917, #25301 ),
 ( #28091, #7583 ),
 ( #15447, #15597 ),
 ( #17738, #2040 ) ),
 .UNSPECIFIED., .F., .F., .F.,
 ( 4, 1, 1, 1, 1, 1, 1, 1, 1, 4 ),
 ( 2, 2 ),
 ( 0.000000000000000000, 0.1905276476008422870, 0.3132527668879307448, 0.4537607744431124135, 0.6164363868674446190, 0.7844992633237182211, 0.8316956887180538827, 0.8778732246798023331, 0.9250987397538774637, 1.000000000000000000 ),
 ( 0.000000000000000000, 1.000000000000000000 ),
 .UNSPECIFIED. ) ;
#30023=EDGE_LOOP ( 'NONE', ( #19778, #1986, #25612, #870 ) ) ;
#30027=ORIENTED_EDGE ( 'NONE', *, *, #3175, .T. ) ;
#30028=ADVANCED_FACE ( 'NONE', ( #14014 ), #13852, .F. ) ;
#30031=EDGE_CURVE ( 'NONE', #29811, #3515, #16784, .T. ) ;
#30034=CARTESIAN_POINT ( 'NONE',  ( -9.938224104479729704, -5.936921830459688465, -13.33304460041354211 ) ) ;
#30038=ORIENTED_EDGE ( 'NONE', *, *, #7350, .F. ) ;
#30042=DIRECTION ( 'NONE',  ( 0.000000000000000000, -1.000000000000000000, -1.446921688628131436E-16 ) ) ;
#30054=CARTESIAN_POINT ( 'NONE',  ( 52.17126980765626598, -5.936694392936854747, 107.4222244474858172 ) ) ;
#30056=VERTEX_POINT ( 'NONE', #11713 ) ;
#30059=CARTESIAN_POINT ( 'NONE',  ( -63.90214402394282445, 11.92558985988973497, 26.63511333407100778 ) ) ;
#30063=EDGE_CURVE ( 'NONE', #16546, #3409, #30905, .T. ) ;
#30067=DIRECTION ( 'NONE',  ( 0.000000000000000000, -1.000000000000000000, -0.000000000000000000 ) ) ;
#30069=ORIENTED_EDGE ( 'NONE', *, *, #32352, .F. ) ;
#30073=CIRCLE ( 'NONE', #30006, 19.99999999999999645 ) ;
#30075=EDGE_CURVE ( 'NONE', #3078, #3737, #11129, .T. ) ;
#30086=CARTESIAN_POINT ( 'NONE',  ( 21.09785597605719332, 25.56454579224779877, 75.54930799450052348 ) ) ;
#30090=CARTESIAN_POINT ( 'NONE',  ( 21.09785597605719332, 13.74476430820393347, 47.04930799450051637 ) ) ;
#30093=CARTESIAN_POINT ( 'NONE',  ( 52.07598125554711999, -5.935454207752202116, 105.0538709090500333 ) ) ;
#30101=CARTESIAN_POINT ( 'NONE',  ( 21.09785597605719332, 15.56454579224779877, 47.04930799450051637 ) ) ;
#30103=CARTESIAN_POINT ( 'NONE',  ( -14.16142858629410028, -3.295808585244882849, -3.351769630585352377 ) ) ;
#30113=CARTESIAN_POINT ( 'NONE',  ( 21.09785597605720042, -8.874820941924726370, 114.4370741995029448 ) ) ;
#30118=CARTESIAN_POINT ( 'NONE',  ( 80.31073949092039754, -5.884593569754257736, 78.41992512317908393 ) ) ;
#30122=AXIS2_PLACEMENT_3D ( 'NONE', #26016, #11104, #21087 ) ;
#30125=CARTESIAN_POINT ( 'NONE',  ( 77.73252811823751074, -5.211355130743528186, 79.66972472706787300 ) ) ;
#30129=LINE ( 'NONE', #13053, #4591 ) ;
#30131=CARTESIAN_POINT ( 'NONE',  ( 74.78853601277438656, 0.3723237022603859137, 80.12755559773067660 ) ) ;
#30145=AXIS2_PLACEMENT_3D ( 'NONE', #22007, #14644, #19875 ) ;
#30150=CARTESIAN_POINT ( 'NONE',  ( -9.760762082419509156, -5.936463533621010313, 107.7460900765755980 ) ) ;
#30154=CARTESIAN_POINT ( 'NONE',  ( 77.78074022173946389, -5.264348929021202217, 14.45247463199519267 ) ) ;
#30155=CARTESIAN_POINT ( 'NONE',  ( 44.24985019830227628, 11.56016961077985350, -4.887484607911599888 ) ) ;
#30162=CARTESIAN_POINT ( 'NONE',  ( -34.69359713753573260, -3.406866929052813742, 13.39243194667643344 ) ) ;
#30166=FACE_OUTER_BOUND ( 'NONE', #22372, .T. ) ;
#30171=AXIS2_PLACEMENT_3D ( 'NONE', #11612, #4224, #18660 ) ;
#30174=ORIENTED_EDGE ( 'NONE', *, *, #8799, .T. ) ;
#30200=PLANE ( 'NONE',  #32276 ) ;
#30202=CARTESIAN_POINT ( 'NONE',  ( 51.92400919103565116, -5.935454207752198563, -12.64839579672098679 ) ) ;
#30203=CARTESIAN_POINT ( 'NONE',  ( 21.09785597605719332, 11.92558985988973497, 47.04930799450051637 ) ) ;
#30205=ORIENTED_EDGE ( 'NONE', *, *, #28366, .T. ) ;
#30209=DIRECTION ( 'NONE',  ( 0.000000000000000000, 0.000000000000000000, -1.000000000000000000 ) ) ;
#30211=CARTESIAN_POINT ( 'NONE',  ( 52.20929784716416577, -5.935454207834595763, 107.5147914783766510 ) ) ;
#30212=ORIENTED_EDGE ( 'NONE', *, *, #25128, .T. ) ;
#30214=DIRECTION ( 'NONE',  ( 0.000000000000000000, 0.000000000000000000, -1.000000000000000000 ) ) ;
#30220=ADVANCED_FACE ( 'NONE', ( #2187 ), #12155, .F. ) ;
#30222=CIRCLE ( 'NONE', #31781, 2.500000000000002220 ) ;
#30229=LINE ( 'NONE', #23793, #31885 ) ;
#30238=FACE_OUTER_BOUND ( 'NONE', #30664, .T. ) ;
#30242=ORIENTED_EDGE ( 'NONE', *, *, #32322, .T. ) ;
#30248=CIRCLE ( 'NONE', #21836, 3.300000000000000711 ) ;
#30249=CARTESIAN_POINT ( 'NONE',  ( 47.79865503179234310, 9.702389020015065313, 97.51081847724526597 ) ) ;
#30255=ORIENTED_EDGE ( 'NONE', *, *, #6844, .T. ) ;
#30268=CARTESIAN_POINT ( 'NONE',  ( -9.883074696779189594, -5.935345006353231589, 107.7511683020618705 ) ) ;
#30274=CARTESIAN_POINT ( 'NONE',  ( 80.74398714568756930, -5.940946157296531638, 78.01708044332235659 ) ) ;
#30281=CARTESIAN_POINT ( 'NONE',  ( -9.993688792838534951, -5.936209625872266749, -13.51616825880646111 ) ) ;
#30286=ORIENTED_EDGE ( 'NONE', *, *, #25899, .T. ) ;
#30288=DIRECTION ( 'NONE',  ( 0.000000000000000000, 0.000000000000000000, -1.000000000000000000 ) ) ;
#30294=VERTEX_POINT ( 'NONE', #17928 ) ;
#30295=B_SPLINE_SURFACE_WITH_KNOTS ( 'NONE', 3, 1, ( 
 ( #19255, #29613 ),
 ( #7126, #24350 ),
 ( #4499, #9262 ),
 ( #21722, #29281 ) ),
 .UNSPECIFIED., .F., .F., .F.,
 ( 4, 4 ),
 ( 2, 2 ),
 ( 0.9911194921636459210, 1.000000000000000000 ),
 ( 0.000000000000000000, 1.000000000000000000 ),
 .UNSPECIFIED. ) ;
#30313=CARTESIAN_POINT ( 'NONE',  ( -31.35900179296935519, 11.88363633076758674, 68.52907228695418951 ) ) ;
#30315=ORIENTED_EDGE ( 'NONE', *, *, #13912, .F. ) ;
#30316=CARTESIAN_POINT ( 'NONE',  ( -11.90685058024091170, 0.5083845707908509759, 99.75471799201011436 ) ) ;
#30317=ORIENTED_EDGE ( 'NONE', *, *, #8975, .F. ) ;
#30320=EDGE_CURVE ( 'NONE', #28041, #22873, #15336, .T. ) ;
#30324=CARTESIAN_POINT ( 'NONE',  ( 21.09785597605719332, -5.935454207752083988, 47.04930799450039558 ) ) ;
#30328=CARTESIAN_POINT ( 'NONE',  ( 21.09785597605719332, 13.74476430820393347, 47.04930799450051637 ) ) ;
#30331=DIRECTION ( 'NONE',  ( 0.000000000000000000, -1.000000000000000000, -0.000000000000000000 ) ) ;
#30336=CARTESIAN_POINT ( 'NONE',  ( -63.90214402394282445, -5.935454207752198563, 54.04930799450053058 ) ) ;
#30339=ORIENTED_EDGE ( 'NONE', *, *, #28012, .F. ) ;
#30340=CARTESIAN_POINT ( 'NONE',  ( 21.09785597605719332, -9.935454207752199451, 47.04930799450051637 ) ) ;
#30369=CARTESIAN_POINT ( 'NONE',  ( -9.733400645194006273, -5.935667572904992362, 107.6074630748240537 ) ) ;
#30376=CARTESIAN_POINT ( 'NONE',  ( -31.75494777190936802, 11.92558985988973674, 26.63511333407100778 ) ) ;
#30380=AXIS2_PLACEMENT_3D ( 'NONE', #30340, #17363, #32478 ) ;
#30393=PLANE ( 'NONE',  #1827 ) ;
#30406=DIRECTION ( 'NONE',  ( 0.000000000000000000, 0.000000000000000000, 1.000000000000000000 ) ) ;
#30419=DIRECTION ( 'NONE',  ( 0.000000000000000000, -0.2756373558165849391, -0.9612616959384376880 ) ) ;
#30427=CARTESIAN_POINT ( 'NONE',  ( 21.09785597605719332, -5.935454207752083988, 47.04930799449963530 ) ) ;
#30439=LINE ( 'NONE', #12726, #29651 ) ;
#30443=ADVANCED_FACE ( 'NONE', ( #9659 ), #3265, .T. ) ;
#30444=CARTESIAN_POINT ( 'NONE',  ( -1.500160953227123395, 11.69997306056223607, 99.14540122386770804 ) ) ;
#30446=CARTESIAN_POINT ( 'NONE',  ( 106.0978559760574029, 9.702389020015065313, 73.75010705023596813 ) ) ;
#30451=CARTESIAN_POINT ( 'NONE',  ( 81.54157720457462233, -5.936746300155055778, 77.98036360551803625 ) ) ;
#30456=VERTEX_POINT ( 'NONE', #32312 ) ;
#30463=DIRECTION ( 'NONE',  ( 0.000000000000000000, 0.000000000000000000, -1.000000000000000000 ) ) ;
#30465=AXIS2_PLACEMENT_3D ( 'NONE', #5286, #27442, #5603 ) ;
#30471=EDGE_CURVE ( 'NONE', #3737, #5905, #19000, .T. ) ;
#30475=CARTESIAN_POINT ( 'NONE',  ( 81.46980107077142463, -5.937449718911897101, 16.02633765848928249 ) ) ;
#30477=EDGE_LOOP ( 'NONE', ( #16332, #558, #619, #20925 ) ) ;
#30478=DIRECTION ( 'NONE',  ( 1.000000000000000000, -0.000000000000000000, 1.224646799147353207E-16 ) ) ;
#30481=CARTESIAN_POINT ( 'NONE',  ( -34.18913700378557508, -2.705599144416646951, 80.78811439151294849 ) ) ;
#30486=CARTESIAN_POINT ( 'NONE',  ( -11.52256075650998035, -5.211355130743549502, 103.6839801366810292 ) ) ;
#30510=VECTOR ( 'NONE', #1366, 1000.000000000000000 ) ;
#30514=ORIENTED_EDGE ( 'NONE', *, *, #3709, .F. ) ;
#30522=EDGE_CURVE ( 'NONE', #25945, #29942, #10478, .T. ) ;
#30530=CARTESIAN_POINT ( 'NONE',  ( -10.74933306299440083, -5.721341737285946749, 105.3592130793008721 ) ) ;
#30531=AXIS2_PLACEMENT_3D ( 'NONE', #11313, #28701, #6384 ) ;
#30536=CARTESIAN_POINT ( 'NONE',  ( 21.09785597605720042, 12.26495659406217342, 103.5194520131186096 ) ) ;
#30544=CARTESIAN_POINT ( 'NONE',  ( -30.86621176729672200, 11.58648227300037803, 23.99474104113578221 ) ) ;
#30545=EDGE_LOOP ( 'NONE', ( #7140, #27212, #30212, #29027 ) ) ;
#30550=EDGE_CURVE ( 'NONE', #4386, #9438, #2593, .T. ) ;
#30555=DIRECTION ( 'NONE',  ( 8.659560562354994488E-17, -0.7071067811865426878, 0.7071067811865524577 ) ) ;
#30575=CARTESIAN_POINT ( 'NONE',  ( 49.40425470046338319, 8.190330151142697801, 97.59131769823768821 ) ) ;
#30583=ORIENTED_EDGE ( 'NONE', *, *, #14643, .F. ) ;
#30587=CARTESIAN_POINT ( 'NONE',  ( -39.39994726806853009, -5.935969479811864069, 77.95691600913359309 ) ) ;
#30595=CIRCLE ( 'NONE', #15403, 54.30000000000000426 ) ;
#30596=AXIS2_PLACEMENT_3D ( 'NONE', #11082, #23540, #8288 ) ;
#30604=CARTESIAN_POINT ( 'NONE',  ( -5.147605652606496385, 10.07047442526145531, -3.422300758029766854 ) ) ;
#30607=LINE ( 'NONE', #8118, #11844 ) ;
#30611=VECTOR ( 'NONE', #31867, 1000.000000000000000 ) ;
#30615=LINE ( 'NONE', #1934, #18173 ) ;
#30622=DIRECTION ( 'NONE',  ( 0.000000000000000000, 0.000000000000000000, -1.000000000000000000 ) ) ;
#30631=EDGE_CURVE ( 'NONE', #22618, #29979, #138, .T. ) ;
#30635=FACE_OUTER_BOUND ( 'NONE', #22948, .T. ) ;
#30638=CARTESIAN_POINT ( 'NONE',  ( -34.42886191242200056, 11.85135941024610418, 40.60668834306612496 ) ) ;
#30652=CARTESIAN_POINT ( 'NONE',  ( 81.72311593397060392, -5.936969727347467085, 16.00772641743157720 ) ) ;
#30659=EDGE_CURVE ( 'NONE', #15925, #4643, #31065, .T. ) ;
#30664=EDGE_LOOP ( 'NONE', ( #20285, #32077, #11438, #27884 ) ) ;
#30668=AXIS2_PLACEMENT_3D ( 'NONE', #18629, #18149, #18308 ) ;
#30673=ORIENTED_EDGE ( 'NONE', *, *, #32319, .F. ) ;
#30685=VECTOR ( 'NONE', #29791, 1000.000000000000000 ) ;
#30687=ADVANCED_FACE ( 'NONE', ( #26038 ), #20313, .F. ) ;
#30689=AXIS2_PLACEMENT_3D ( 'NONE', #8579, #30751, #13672 ) ;
#30692=DIRECTION ( 'NONE',  ( 8.659560562355053653E-17, -0.7071067811865378028, 0.7071067811865573427 ) ) ;
#30699=CYLINDRICAL_SURFACE ( 'NONE', #29849, 54.29999999999999716 ) ;
#30712=DIRECTION ( 'NONE',  ( -0.000000000000000000, 1.000000000000000000, -0.000000000000000000 ) ) ;
#30714=AXIS2_PLACEMENT_3D ( 'NONE', #28244, #30712, #28086 ) ;
#30717=DIRECTION ( 'NONE',  ( 0.000000000000000000, -1.000000000000000000, -0.000000000000000000 ) ) ;
#30733=CIRCLE ( 'NONE', #29152, 66.44011198581388555 ) ;
#30738=CARTESIAN_POINT ( 'NONE',  ( 54.69690332803826749, -1.331120222581874346, 100.5855669984461258 ) ) ;
#30747=CARTESIAN_POINT ( 'NONE',  ( -34.95779894681891165, 11.10722333531405148, 52.41483564559372610 ) ) ;
#30751=DIRECTION ( 'NONE',  ( 0.000000000000000000, 1.000000000000000000, 0.000000000000000000 ) ) ;
#30761=CARTESIAN_POINT ( 'NONE',  ( 21.09785597605719332, -9.935454207752199451, -20.95069200549946231 ) ) ;
#30781=VERTEX_POINT ( 'NONE', #5879 ) ;
#30786=CARTESIAN_POINT ( 'NONE',  ( 81.46980107077142463, -5.935340315990521809, 15.93528473569102566 ) ) ;
#30798=ORIENTED_EDGE ( 'NONE', *, *, #11046, .F. ) ;
#30804=CARTESIAN_POINT ( 'NONE',  ( -35.16155806787664062, 11.92558985988975806, 53.76629232714613238 ) ) ;
#30806=DIRECTION ( 'NONE',  ( -0.000000000000000000, 1.000000000000000000, -0.000000000000000000 ) ) ;
#30821=CARTESIAN_POINT ( 'NONE',  ( -11.98523041842830850, -4.708525186292168208, 104.0193796289731409 ) ) ;
#30827=ADVANCED_FACE ( 'NONE', ( #17147 ), #4206, .F. ) ;
#30841=AXIS2_PLACEMENT_3D ( 'NONE', #3891, #19297, #11286 ) ;
#30864=ORIENTED_EDGE ( 'NONE', *, *, #3195, .F. ) ;
#30885=DIRECTION ( 'NONE',  ( 0.000000000000000000, 0.000000000000000000, 1.000000000000000000 ) ) ;
#30902=EDGE_CURVE ( 'NONE', #28880, #14836, #21753, .T. ) ;
#30905=B_SPLINE_CURVE_WITH_KNOTS ( 'NONE', 3,
 ( #31414, #21867, #8917, #16303, #11382, #21706, #19236, #31737 ),
 .UNSPECIFIED., .F., .F.,
 ( 4, 2, 2, 4 ),
 ( 0.0005577589035164437319, 0.001153159837334056647, 0.001748560771151669779, 0.002939362638786875877 ),
 .UNSPECIFIED. ) ;
#30912=ADVANCED_FACE ( 'NONE', ( #7153 ), #27832, .F. ) ;
#30913=FACE_OUTER_BOUND ( 'NONE', #8792, .T. ) ;
#30917=ORIENTED_EDGE ( 'NONE', *, *, #21431, .T. ) ;
#30923=CARTESIAN_POINT ( 'NONE',  ( -4.653529917572326369, 10.40182650318958579, 98.46608932373301570 ) ) ;
#30938=AXIS2_PLACEMENT_3D ( 'NONE', #15174, #12397, #32256 ) ;
#30941=CARTESIAN_POINT ( 'NONE',  ( 47.79865503179234310, 9.702389020015065313, -4.315940132965163656 ) ) ;
#30958=EDGE_LOOP ( 'NONE', ( #22351, #23840 ) ) ;
#30963=CARTESIAN_POINT ( 'NONE',  ( -36.86121898886836590, -5.510771003736198992, 79.29205363043402599 ) ) ;
#30967=DIRECTION ( 'NONE',  ( 0.000000000000000000, 0.000000000000000000, -1.000000000000000000 ) ) ;
#30985=VERTEX_POINT ( 'NONE', #22897 ) ;
#30987=CARTESIAN_POINT ( 'NONE',  ( -11.32029359255892764, -5.395280703882725959, 104.8375434467133118 ) ) ;
#30998=CARTESIAN_POINT ( 'NONE',  ( 21.09785597605719332, 12.06852548259731961, -8.628907523723306383 ) ) ;
#30999=DIRECTION ( 'NONE',  ( 0.000000000000000000, 1.000000000000000000, 0.000000000000000000 ) ) ;
#31005=ORIENTED_EDGE ( 'NONE', *, *, #4262, .F. ) ;
#31014=CARTESIAN_POINT ( 'NONE',  ( -33.25903338348492611, -2.742229146546061980, 13.28678055525370993 ) ) ;
#31017=DIRECTION ( 'NONE',  ( -0.000000000000000000, -1.000000000000000000, -0.000000000000000000 ) ) ;
#31021=CARTESIAN_POINT ( 'NONE',  ( 47.09785597605719687, 25.56454579224779877, 47.04930799450042400 ) ) ;
#31052=PLANE ( 'NONE',  #8830 ) ;
#31064=DIRECTION ( 'NONE',  ( 0.000000000000000000, 0.000000000000000000, -1.000000000000000000 ) ) ;
#31065=CIRCLE ( 'NONE', #16892, 2.500000000000002220 ) ;
#31072=ORIENTED_EDGE ( 'NONE', *, *, #22862, .T. ) ;
#31077=CARTESIAN_POINT ( 'NONE',  ( 72.64898409407776114, 3.957035103101694151, 15.81524687697156928 ) ) ;
#31078=VERTEX_POINT ( 'NONE', #32431 ) ;
#31079=DIRECTION ( 'NONE',  ( 1.000000000000000000, 0.000000000000000000, -1.110223024625154963E-14 ) ) ;
#31085=FILL_AREA_STYLE_COLOUR ( '', #3441 ) ;
#31100=EDGE_CURVE ( 'NONE', #6039, #5895, #25339, .T. ) ;
#31101=ADVANCED_FACE ( 'NONE', ( #1057 ), #26903, .F. ) ;
#31104=EDGE_CURVE ( 'NONE', #2726, #13343, #8565, .T. ) ;
#31115=CARTESIAN_POINT ( 'NONE',  ( -36.98761417531858342, -5.935454207752198563, 77.87546120947918382 ) ) ;
#31117=VERTEX_POINT ( 'NONE', #25686 ) ;
#31120=CIRCLE ( 'NONE', #12793, 71.29999999999996874 ) ;
#31122=CARTESIAN_POINT ( 'NONE',  ( 21.09785597605719332, 16.86454579224779948, -1.584744370635042587 ) ) ;
#31143=EDGE_CURVE ( 'NONE', #12308, #29171, #10915, .T. ) ;
#31148=ORIENTED_EDGE ( 'NONE', *, *, #23274, .T. ) ;
#31156=DIRECTION ( 'NONE',  ( 1.000000000000000000, 0.000000000000000000, -1.110223024625154963E-14 ) ) ;
#31157=CARTESIAN_POINT ( 'NONE',  ( 21.09785597605719332, 25.13358275951983956, 7.413771787092404253 ) ) ;
#31160=ORIENTED_EDGE ( 'NONE', *, *, #12950, .F. ) ;
#31182=ORIENTED_EDGE ( 'NONE', *, *, #31895, .T. ) ;
#31185=CARTESIAN_POINT ( 'NONE',  ( 21.09785597605720042, 25.18020726757345429, 87.53672989447419184 ) ) ;
#31187=ORIENTED_EDGE ( 'NONE', *, *, #32280, .T. ) ;
#31192=LINE ( 'NONE', #23472, #31757 ) ;
#31193=AXIS2_PLACEMENT_3D ( 'NONE', #24040, #1552, #7141 ) ;
#31197=ORIENTED_EDGE ( 'NONE', *, *, #29810, .F. ) ;
#31199=CARTESIAN_POINT ( 'NONE',  ( -35.17013276111289599, 11.90988849664400284, 40.33535627974906390 ) ) ;
#31210=DIRECTION ( 'NONE',  ( 1.000000000000000000, -0.000000000000000000, -0.000000000000000000 ) ) ;
#31220=EDGE_CURVE ( 'NONE', #27541, #10718, #3310, .T. ) ;
#31226=CIRCLE ( 'NONE', #29622, 84.30000000000001137 ) ;
#31230=ORIENTED_EDGE ( 'NONE', *, *, #26049, .T. ) ;
#31249=CARTESIAN_POINT ( 'NONE',  ( 21.09785597605720397, -16.63545420775219696, 131.2593585008393973 ) ) ;
#31253=EDGE_LOOP ( 'NONE', ( #25857, #779 ) ) ;
#31255=DIRECTION ( 'NONE',  ( 1.000000000000000000, -0.000000000000000000, -0.000000000000000000 ) ) ;
#31258=ADVANCED_FACE ( 'NONE', ( #29445 ), #15357, .F. ) ;
#31260=CARTESIAN_POINT ( 'NONE',  ( 21.09785597605719332, 11.78014697381582643, 102.6448323059792358 ) ) ;
#31261=CARTESIAN_POINT ( 'NONE',  ( 21.09785597605719332, 14.56957104541719694, 47.04930799450051637 ) ) ;
#31271=CARTESIAN_POINT ( 'NONE',  ( -33.01793443960422536, -2.346508597185796852, 80.78329740893839528 ) ) ;
#31283=DIRECTION ( 'NONE',  ( -0.000000000000000000, -1.000000000000000000, 0.000000000000000000 ) ) ;
#31291=DIRECTION ( 'NONE',  ( -0.000000000000000000, -1.000000000000000000, -0.000000000000000000 ) ) ;
#31295=ORIENTED_EDGE ( 'NONE', *, *, #22444, .T. ) ;
#31297=CARTESIAN_POINT ( 'NONE',  ( -43.49322394822878834, -4.178071014601207445, 42.04930799450081480 ) ) ;
#31298=B_SPLINE_CURVE_WITH_KNOTS ( 'NONE', 3,
 ( #5765, #674, #15772, #3451, #5284, #20848, #3289, #343, #8547, #25302, #23478, #13326 ),
 .UNSPECIFIED., .F., .F.,
 ( 4, 2, 2, 2, 2, 4 ),
 ( 0.0003078418816949101658, 0.0003848023521186742855, 0.0004232825873305365045, 0.0004617628225423987235, 0.0005387232929661524890, 0.0006156837633899062004 ),
 .UNSPECIFIED. ) ;
#31322=CARTESIAN_POINT ( 'NONE',  ( 21.09785597605719332, -16.43042895458278352, 47.04930799450051637 ) ) ;
#31326=CARTESIAN_POINT ( 'NONE',  ( -30.88361648749964772, 11.92558985988973141, 26.60346110398183583 ) ) ;
#31357=CARTESIAN_POINT ( 'NONE',  ( 21.09785597605719332, -15.93545420775219945, 47.04930799450051637 ) ) ;
#31362=CIRCLE ( 'NONE', #15633, 2.500000000000002220 ) ;
#31363=FACE_BOUND ( 'NONE', #12830, .T. ) ;
#31372=CARTESIAN_POINT ( 'NONE',  ( 0.6836613156275053171, 11.92558985988973497, -37.95069200549950494 ) ) ;
#31385=CARTESIAN_POINT ( 'NONE',  ( 52.07598464021349116, -5.935454078358230134, -13.51145360256171557 ) ) ;
#31407=CARTESIAN_POINT ( 'NONE',  ( 81.60489042199095877, -5.935454337261173663, 78.02742988628502019 ) ) ;
#31414=CARTESIAN_POINT ( 'NONE',  ( -45.06166779280744095, -5.721341737285086992, 40.94964444931001424 ) ) ;
#31419=DIRECTION ( 'NONE',  ( -1.000000000000000000, 0.000000000000000000, 0.000000000000000000 ) ) ;
#31426=AXIS2_PLACEMENT_3D ( 'NONE', #2715, #23381, #7649 ) ;
#31434=DIRECTION ( 'NONE',  ( 0.000000000000000000, -1.000000000000000000, 0.000000000000000000 ) ) ;
#31458=ORIENTED_EDGE ( 'NONE', *, *, #20879, .F. ) ;
#31465=EDGE_CURVE ( 'NONE', #23296, #1152, #28459, .T. ) ;
#31466=EDGE_CURVE ( 'NONE', #13013, #11449, #5454, .T. ) ;
#31471=AXIS2_PLACEMENT_3D ( 'NONE', #14597, #28003, #10289 ) ;
#31481=CARTESIAN_POINT ( 'NONE',  ( -8.048943652745618849, 7.198184577528760286, -3.649531620208970484 ) ) ;
#31492=ADVANCED_FACE ( 'NONE', ( #23505 ), #8414, .F. ) ;
#31493=ORIENTED_EDGE ( 'NONE', *, *, #30550, .F. ) ;
#31498=EDGE_CURVE ( 'NONE', #12308, #7388, #25648, .T. ) ;
#31509=EDGE_CURVE ( 'NONE', #9808, #19261, #26127, .T. ) ;
#31522=CARTESIAN_POINT ( 'NONE',  ( -35.89521036423793987, 10.88979515353705807, 41.81960461513401839 ) ) ;
#31523=CARTESIAN_POINT ( 'NONE',  ( 72.46310410352296572, 9.702389020015065313, 20.34850893876554778 ) ) ;
#31539=ORIENTED_EDGE ( 'NONE', *, *, #27488, .F. ) ;
#31546=EDGE_CURVE ( 'NONE', #32110, #7248, #21180, .T. ) ;
#31549=EDGE_LOOP ( 'NONE', ( #2530, #10846 ) ) ;
#31554=DIRECTION ( 'NONE',  ( 0.000000000000000000, 0.000000000000000000, -1.000000000000000000 ) ) ;
#31567=( NAMED_UNIT ( * ) SI_UNIT ( $, .STERADIAN. ) SOLID_ANGLE_UNIT ( ) );
#31575=ORIENTED_EDGE ( 'NONE', *, *, #17570, .F. ) ;
#31577=CARTESIAN_POINT ( 'NONE',  ( -39.56501946919145496, -5.936124025396923187, 77.93580931442834014 ) ) ;
#31580=VERTEX_POINT ( 'NONE', #16748 ) ;
#31589=VERTEX_POINT ( 'NONE', #19046 ) ;
#31596=DIRECTION ( 'NONE',  ( 0.000000000000000000, 0.000000000000000000, -1.000000000000000000 ) ) ;
#31597=CARTESIAN_POINT ( 'NONE',  ( 81.79977007715724824, -5.936747322758277434, 77.92211803829925998 ) ) ;
#31603=ORIENTED_EDGE ( 'NONE', *, *, #7350, .T. ) ;
#31626=VERTEX_POINT ( 'NONE', #18715 ) ;
#31632=B_SPLINE_CURVE_WITH_KNOTS ( 'NONE', 3,
 ( #10964, #23103, #3555, #23269, #25734, #3239, #13585, #13276, #8333, #621, #15715, #15886, #10651, #8180, #18171, #20955, #5882, #16035, #780, #28523, #20802, #3396, #28363, #23428, #935, #30821, #25890, #30987, #8497, #5332 ),
 .UNSPECIFIED., .F., .F.,
 ( 4, 2, 2, 2, 2, 2, 2, 2, 2, 2, 2, 2, 2, 2, 4 ),
 ( 0.000000000000000000, 0.001249755272498796928, 0.002499510544997593856, 0.003749265817496392952, 0.004999021089995192048, 0.007498531634992787638, 0.009998042179990382361, 0.01249755272498797795, 0.01374730799748676707, 0.01499706326998555272, 0.01562194090623493514, 0.01624681854248431756, 0.01749657381498308586, 0.01874632908748184723, 0.01999608435998061207 ),
 .UNSPECIFIED. ) ;
#31636=AXIS2_PLACEMENT_3D ( 'NONE', #21062, #21219, #23699 ) ;
#31638=CARTESIAN_POINT ( 'NONE',  ( -4.902144023942810236, 24.86454579224779948, 47.04930799450078638 ) ) ;
#31643=EDGE_CURVE ( 'NONE', #12487, #27983, #31703, .T. ) ;
#31645=CARTESIAN_POINT ( 'NONE',  ( -38.57070939289658895, -5.937181781424613725, 77.94502167843351970 ) ) ;
#31650=CARTESIAN_POINT ( 'NONE',  ( -41.59221397235413775, 0.6853201964616114639, 42.04930799450051637 ) ) ;
#31661=DIRECTION ( 'NONE',  ( 0.000000000000000000, -1.000000000000000000, 0.000000000000000000 ) ) ;
#31679=FACE_OUTER_BOUND ( 'NONE', #966, .T. ) ;
#31680=CARTESIAN_POINT ( 'NONE',  ( 74.49868417184303837, 1.147918989839205040, 14.32049971022470558 ) ) ;
#31683=EDGE_LOOP ( 'NONE', ( #12696, #9292, #12579, #10111 ) ) ;
#31697=CARTESIAN_POINT ( 'NONE',  ( -11.80969419479644777, -4.922489993312313850, -10.15873547626677365 ) ) ;
#31703=LINE ( 'NONE', #9214, #1755 ) ;
#31712=CARTESIAN_POINT ( 'NONE',  ( 21.09785597605720042, -9.935454207752199451, 115.0493079945004951 ) ) ;
#31719=CARTESIAN_POINT ( 'NONE',  ( 21.09785597605720397, -19.93545420775220123, -37.25069200549950210 ) ) ;
#31726=AXIS2_PLACEMENT_3D ( 'NONE', #18701, #16250, #14124 ) ;
#31729=CIRCLE ( 'NONE', #288, 66.44011198581388555 ) ;
#31732=CARTESIAN_POINT ( 'NONE',  ( -30.88361648749964772, 11.92558985988973141, 26.60346110398183583 ) ) ;
#31737=CARTESIAN_POINT ( 'NONE',  ( -44.16105795751995799, -3.935454207752190126, 42.04930799450051637 ) ) ;
#31742=FACE_OUTER_BOUND ( 'NONE', #6573, .T. ) ;
#31754=CARTESIAN_POINT ( 'NONE',  ( -31.82365885725337051, -0.03213146785430506802, 80.27334318690746784 ) ) ;
#31757=VECTOR ( 'NONE', #14112, 1000.000000000000000 ) ;
#31764=ORIENTED_EDGE ( 'NONE', *, *, #7256, .F. ) ;
#31775=CARTESIAN_POINT ( 'NONE',  ( -44.31161278331510545, -5.876499408311634198, 40.60422303027608848 ) ) ;
#31776=VECTOR ( 'NONE', #32497, 1000.000000000000000 ) ;
#31778=ORIENTED_EDGE ( 'NONE', *, *, #782, .T. ) ;
#31779=ORIENTED_EDGE ( 'NONE', *, *, #32139, .T. ) ;
#31781=AXIS2_PLACEMENT_3D ( 'NONE', #4011, #31434, #16317 ) ;
#31786=ADVANCED_FACE ( 'NONE', ( #14798 ), #20028, .F. ) ;
#31787=ORIENTED_EDGE ( 'NONE', *, *, #10627, .F. ) ;
#31788=ORIENTED_EDGE ( 'NONE', *, *, #14679, .T. ) ;
#31800=CARTESIAN_POINT ( 'NONE',  ( -12.61912916467185042, -3.025068871688601391, -7.519726213196242348 ) ) ;
#31802=LINE ( 'NONE', #10709, #3740 ) ;
#31826=CARTESIAN_POINT ( 'NONE',  ( 49.52052953415556402, 8.310461108307681144, -12.70392589783158499 ) ) ;
#31835=CARTESIAN_POINT ( 'NONE',  ( 72.50786317273436055, 8.583949016299403212, 19.11078817837193711 ) ) ;
#31846=CARTESIAN_POINT ( 'NONE',  ( -45.71603902977910394, -5.927433539347818581, 40.25072284635503195 ) ) ;
#31849=ORIENTED_EDGE ( 'NONE', *, *, #7415, .T. ) ;
#31855=CARTESIAN_POINT ( 'NONE',  ( -12.61887306221779248, -2.123693335316770181, -7.872981162211413420 ) ) ;
#31867=DIRECTION ( 'NONE',  ( 1.000000000000000000, -0.000000000000000000, -0.000000000000000000 ) ) ;
#31869=CARTESIAN_POINT ( 'NONE',  ( 72.46987649561761202, 10.07216359114295834, 73.29268005255001128 ) ) ;
#31884=CARTESIAN_POINT ( 'NONE',  ( -35.64882101543633297, 9.925589859889724309, 52.04930799450051637 ) ) ;
#31885=VECTOR ( 'NONE', #8546, 1000.000000000000000 ) ;
#31887=CARTESIAN_POINT ( 'NONE',  ( -29.57057120148431650, 10.93554979939848693, 22.25697859473322637 ) ) ;
#31888=VECTOR ( 'NONE', #28233, 1000.000000000000000 ) ;
#31895=EDGE_CURVE ( 'NONE', #25630, #32279, #22981, .T. ) ;
#31899=CARTESIAN_POINT ( 'NONE',  ( -39.39739818181173803, -5.935454207752198563, 77.87546120947918382 ) ) ;
#31900=DIRECTION ( 'NONE',  ( 0.000000000000000000, 0.000000000000000000, 1.000000000000000000 ) ) ;
#31909=VERTEX_POINT ( 'NONE', #17344 ) ;
#31916=CARTESIAN_POINT ( 'NONE',  ( -30.09469955099472216, 5.197876425781705834, 77.54511166671605338 ) ) ;
#31917=CARTESIAN_POINT ( 'NONE',  ( -38.65545646816406133, -4.281517947942904634, 80.46297774100551692 ) ) ;
#31924=CARTESIAN_POINT ( 'NONE',  ( 21.09785597605719332, 13.06454579224780055, -7.694940604469596934 ) ) ;
#31947=EDGE_CURVE ( 'NONE', #21115, #3553, #9968, .T. ) ;
#31953=ORIENTED_EDGE ( 'NONE', *, *, #13950, .T. ) ;
#31956=FACE_OUTER_BOUND ( 'NONE', #19626, .T. ) ;
#31961=CARTESIAN_POINT ( 'NONE',  ( -9.918530130619847895, 4.323180411458210415, -4.396266667175535048 ) ) ;
#31992=CARTESIAN_POINT ( 'NONE',  ( 21.09785597605719332, -16.63545420775219696, 47.04930799450051637 ) ) ;
#31994=CARTESIAN_POINT ( 'NONE',  ( 47.79865503179234310, 9.702389020015065313, -12.70392589783158499 ) ) ;
#32000=CARTESIAN_POINT ( 'NONE',  ( 78.03121069986417524, -4.668720686625185579, 13.94775564540398172 ) ) ;
#32028=EDGE_CURVE ( 'NONE', #31626, #9845, #26452, .T. ) ;
#32029=ADVANCED_FACE ( 'NONE', ( #20936 ), #1081, .F. ) ;
#32039=CARTESIAN_POINT ( 'NONE',  ( -30.89605511857125464, 11.92558985988973497, 67.46350265493038023 ) ) ;
#32043=CARTESIAN_POINT ( 'NONE',  ( 53.59103788013077008, -5.321843574075685979, -9.729082480673143962 ) ) ;
#32055=CIRCLE ( 'NONE', #8463, 2.500000000000002220 ) ;
#32059=CARTESIAN_POINT ( 'NONE',  ( 52.46240689619265396, -5.913508961333112879, 104.8323960743217782 ) ) ;
#32061=CARTESIAN_POINT ( 'NONE',  ( -39.51359738027355206, -5.935454207752198563, 77.87546120947918382 ) ) ;
#32068=CARTESIAN_POINT ( 'NONE',  ( -10.96598430569368432, -5.983766253076982622, -12.62465409255485582 ) ) ;
#32072=CARTESIAN_POINT ( 'NONE',  ( 72.68275509767009623, 11.86918370369814113, 25.53922971596723102 ) ) ;
#32077=ORIENTED_EDGE ( 'NONE', *, *, #16193, .F. ) ;
#32082=CARTESIAN_POINT ( 'NONE',  ( -30.51040964360577235, 3.734882690806572203, 78.42680211664418266 ) ) ;
#32091=CARTESIAN_POINT ( 'NONE',  ( 21.09785597605719332, 25.18020726757345429, 47.04930799450051637 ) ) ;
#32104=DIRECTION ( 'NONE',  ( 0.000000000000000000, -1.000000000000000000, 0.000000000000000000 ) ) ;
#32110=VERTEX_POINT ( 'NONE', #23408 ) ;
#32117=EDGE_CURVE ( 'NONE', #6039, #8138, #32375, .T. ) ;
#32121=ORIENTED_EDGE ( 'NONE', *, *, #2952, .F. ) ;
#32134=ORIENTED_EDGE ( 'NONE', *, *, #13324, .F. ) ;
#32139=EDGE_CURVE ( 'NONE', #649, #3624, #18589, .T. ) ;
#32146=CARTESIAN_POINT ( 'NONE',  ( -58.11219453028166981, -15.93545420775219945, 47.04930799450023926 ) ) ;
#32147=LINE ( 'NONE', #27207, #25589 ) ;
#32162=CARTESIAN_POINT ( 'NONE',  ( 52.02891158707559782, -5.936746300155039791, -13.39441323401713468 ) ) ;
#32171=ADVANCED_FACE ( 'NONE', ( #19886, #21405, #19563, #2177, #16496, #28977 ), #11262, .T. ) ;
#32200=CIRCLE ( 'NONE', #8623, 2.500000000000003553 ) ;
#32206=CARTESIAN_POINT ( 'NONE',  ( 51.70051226388650178, 5.005525289648587339, -4.203416302359093137 ) ) ;
#32218=LINE ( 'NONE', #30086, #26819 ) ;
#32219=EDGE_CURVE ( 'NONE', #14793, #12758, #5516, .T. ) ;
#32220=VERTEX_POINT ( 'NONE', #17261 ) ;
#32222=FACE_OUTER_BOUND ( 'NONE', #32285, .T. ) ;
#32224=CARTESIAN_POINT ( 'NONE',  ( -30.48931983364116149, 3.805300331231239230, 15.71226580949866936 ) ) ;
#32230=CARTESIAN_POINT ( 'NONE',  ( 42.60075171692322726, 11.88159288520707868, -4.533495379785729362 ) ) ;
#32233=CARTESIAN_POINT ( 'NONE',  ( 21.09785597605719332, 25.56454579224780232, -29.66074251183834676 ) ) ;
#32239=CARTESIAN_POINT ( 'NONE',  ( -39.44404620663942751, -5.935468836302990603, 77.98403960728234097 ) ) ;
#32240=AXIS2_PLACEMENT_3D ( 'NONE', #25896, #461, #16043 ) ;
#32242=VERTEX_POINT ( 'NONE', #6328 ) ;
#32254=VERTEX_POINT ( 'NONE', #18946 ) ;
#32256=DIRECTION ( 'NONE',  ( 0.000000000000000000, 0.000000000000000000, -1.000000000000000000 ) ) ;
#32257=EDGE_CURVE ( 'NONE', #6406, #19298, #24042, .T. ) ;
#32260=CARTESIAN_POINT ( 'NONE',  ( 21.09785597605719332, -6.314304012688826795, 47.04930799450051637 ) ) ;
#32264=CARTESIAN_POINT ( 'NONE',  ( -9.955189926603260631, -5.936918531481698125, -13.56792535344213313 ) ) ;
#32266=CARTESIAN_POINT ( 'NONE',  ( 21.09785597605719332, 13.06454579224780055, 47.04930799450051637 ) ) ;
#32269=DIRECTION ( 'NONE',  ( 0.000000000000000000, 1.000000000000000000, 0.000000000000000000 ) ) ;
#32274=CONICAL_SURFACE ( 'NONE', #822, 40.18714373493281755, 0.6632251157578421541 ) ;
#32276=AXIS2_PLACEMENT_3D ( 'NONE', #4763, #30042, #22466 ) ;
#32278=ADVANCED_FACE ( 'NONE', ( #19439 ), #9188, .F. ) ;
#32279=VERTEX_POINT ( 'NONE', #19600 ) ;
#32280=EDGE_CURVE ( 'NONE', #7700, #18486, #27546, .T. ) ;
#32285=EDGE_LOOP ( 'NONE', ( #11521, #2509, #27173, #4580 ) ) ;
#32286=CARTESIAN_POINT ( 'NONE',  ( 75.54028429221254726, -2.844921901652561758, 13.31754327619664480 ) ) ;
#32293=DIRECTION ( 'NONE',  ( 0.000000000000000000, 0.000000000000000000, -1.000000000000000000 ) ) ;
#32295=CARTESIAN_POINT ( 'NONE',  ( -31.01960144644215944, 5.215771264367748294, 16.56563741377133070 ) ) ;
#32301=CARTESIAN_POINT ( 'NONE',  ( 52.18940074495291270, -5.936209625872266749, 107.6147842478074494 ) ) ;
#32302=DIRECTION ( 'NONE',  ( 0.000000000000000000, 0.000000000000000000, -1.000000000000000000 ) ) ;
#32307=ORIENTED_EDGE ( 'NONE', *, *, #32473, .T. ) ;
#32312=CARTESIAN_POINT ( 'NONE',  ( 21.09785597605720042, 11.92558985988973497, 103.7075660656323635 ) ) ;
#32318=B_SPLINE_CURVE_WITH_KNOTS ( 'NONE', 3,
 ( #32061, #12205, #26480, #26805, #1524, #19234, #29264, #1857, #9742, #17106, #6780, #19408, #4321, #29436, #14338, #3993, #24010, #6946, #14013, #4151, #21538, #31577, #9082, #19074, #29109, #7278, #15467, #23009, #27782, #15311, #25324, #7762, #10559, #5466 ),
 .UNSPECIFIED., .F., .F.,
 ( 4, 3, 3, 3, 3, 3, 3, 3, 3, 3, 3, 4 ),
 ( 0.000000000000000000, 2.818012925147974601E-05, 4.462336330430042420E-05, 5.702956313105841864E-05, 6.695137021320823726E-05, 7.690940289137861662E-05, 8.645711199579805470E-05, 0.0001018866409727163031, 0.0001271972541734457814, 0.0001703223122919903497, 0.0002159547541428134365, 0.0002238713945714089373 ),
 .UNSPECIFIED. ) ;
#32319=EDGE_CURVE ( 'NONE', #6712, #30456, #22798, .T. ) ;
#32322=EDGE_CURVE ( 'NONE', #17291, #5246, #17498, .T. ) ;
#32327=AXIS2_PLACEMENT_3D ( 'NONE', #24968, #26942, #27594 ) ;
#32331=LINE ( 'NONE', #9839, #15362 ) ;
#32340=CARTESIAN_POINT ( 'NONE',  ( 52.38208384728245193, -5.903366343041437148, -12.28331011554775465 ) ) ;
#32352=EDGE_CURVE ( 'NONE', #28041, #29304, #13908, .T. ) ;
#32363=CARTESIAN_POINT ( 'NONE',  ( 73.03464857846923053, 11.56016961077985350, 70.20130221674578763 ) ) ;
#32374=B_SPLINE_SURFACE_WITH_KNOTS ( 'NONE', 3, 1, ( 
 ( #14899, #24409 ),
 ( #1920, #29672 ),
 ( #2256, #32459 ),
 ( #9971, #15059 ) ),
 .UNSPECIFIED., .F., .F., .F.,
 ( 4, 4 ),
 ( 2, 2 ),
 ( 0.1800733115436725096, 0.1889470565094412691 ),
 ( 0.000000000000000000, 1.000000000000000000 ),
 .UNSPECIFIED. ) ;
#32375=LINE ( 'NONE', #21252, #22284 ) ;
#32379=DIRECTION ( 'NONE',  ( 0.000000000000000000, 0.000000000000000000, 1.000000000000000000 ) ) ;
#32380=CARTESIAN_POINT ( 'NONE',  ( 21.09785597605719332, 25.56454579224779877, 21.04930799450051282 ) ) ;
#32386=CARTESIAN_POINT ( 'NONE',  ( 42.05571303064796496, 11.92558985988973141, -4.731146760523925465 ) ) ;
#32398=B_SPLINE_CURVE_WITH_KNOTS ( 'NONE', 3,
 ( #30202, #12484, #29880, #32340, #10181, #9850, #25110, #25274 ),
 .UNSPECIFIED., .F., .F.,
 ( 4, 2, 2, 4 ),
 ( 1.734723475976807094E-17, 0.0004427811193176344959, 0.0008855622386352516445, 0.001771124477270482039 ),
 .UNSPECIFIED. ) ;
#32405=EDGE_CURVE ( 'NONE', #20217, #5246, #23208, .T. ) ;
#32421=CARTESIAN_POINT ( 'NONE',  ( -9.880269303432738681, -5.935454207752202116, -13.48461434800281289 ) ) ;
#32426=ORIENTED_EDGE ( 'NONE', *, *, #8345, .F. ) ;
#32431=CARTESIAN_POINT ( 'NONE',  ( 21.09785597605719332, -19.93545420775220123, 131.3493079945005491 ) ) ;
#32432=ORIENTED_EDGE ( 'NONE', *, *, #7599, .F. ) ;
#32454=CARTESIAN_POINT ( 'NONE',  ( -10.65234575671300021, -5.769399297529553827, 104.5301199837775812 ) ) ;
#32459=CARTESIAN_POINT ( 'NONE',  ( 81.54161849434414933, -5.937394935145312580, 77.97850100859398026 ) ) ;
#32473=EDGE_CURVE ( 'NONE', #18486, #31589, #5644, .T. ) ;
#32478=DIRECTION ( 'NONE',  ( 0.000000000000000000, 0.000000000000000000, -1.000000000000000000 ) ) ;
#32489=AXIS2_PLACEMENT_3D ( 'NONE', #31021, #16069, #21144 ) ;
#32495=EDGE_LOOP ( 'NONE', ( #23512, #919, #25871, #4014 ) ) ;
#32497=DIRECTION ( 'NONE',  ( 0.000000000000000000, -1.000000000000000000, -0.000000000000000000 ) ) ;
#32509=COLOUR_RGB('Dark Blue',0.08,0.2,0.34);
#32510=FILL_AREA_STYLE_COLOUR('',#32509);
#32511=FILL_AREA_STYLE('',(#32510));
#32512=SURFACE_STYLE_FILL_AREA(#32511);
#32513=SURFACE_SIDE_STYLE('',(#32512));
#32514=SURFACE_STYLE_USAGE(.BOTH.,#32513);
#32515=PRESENTATION_STYLE_ASSIGNMENT((#32514));
ENDSEC;
END-ISO-10303-21;
